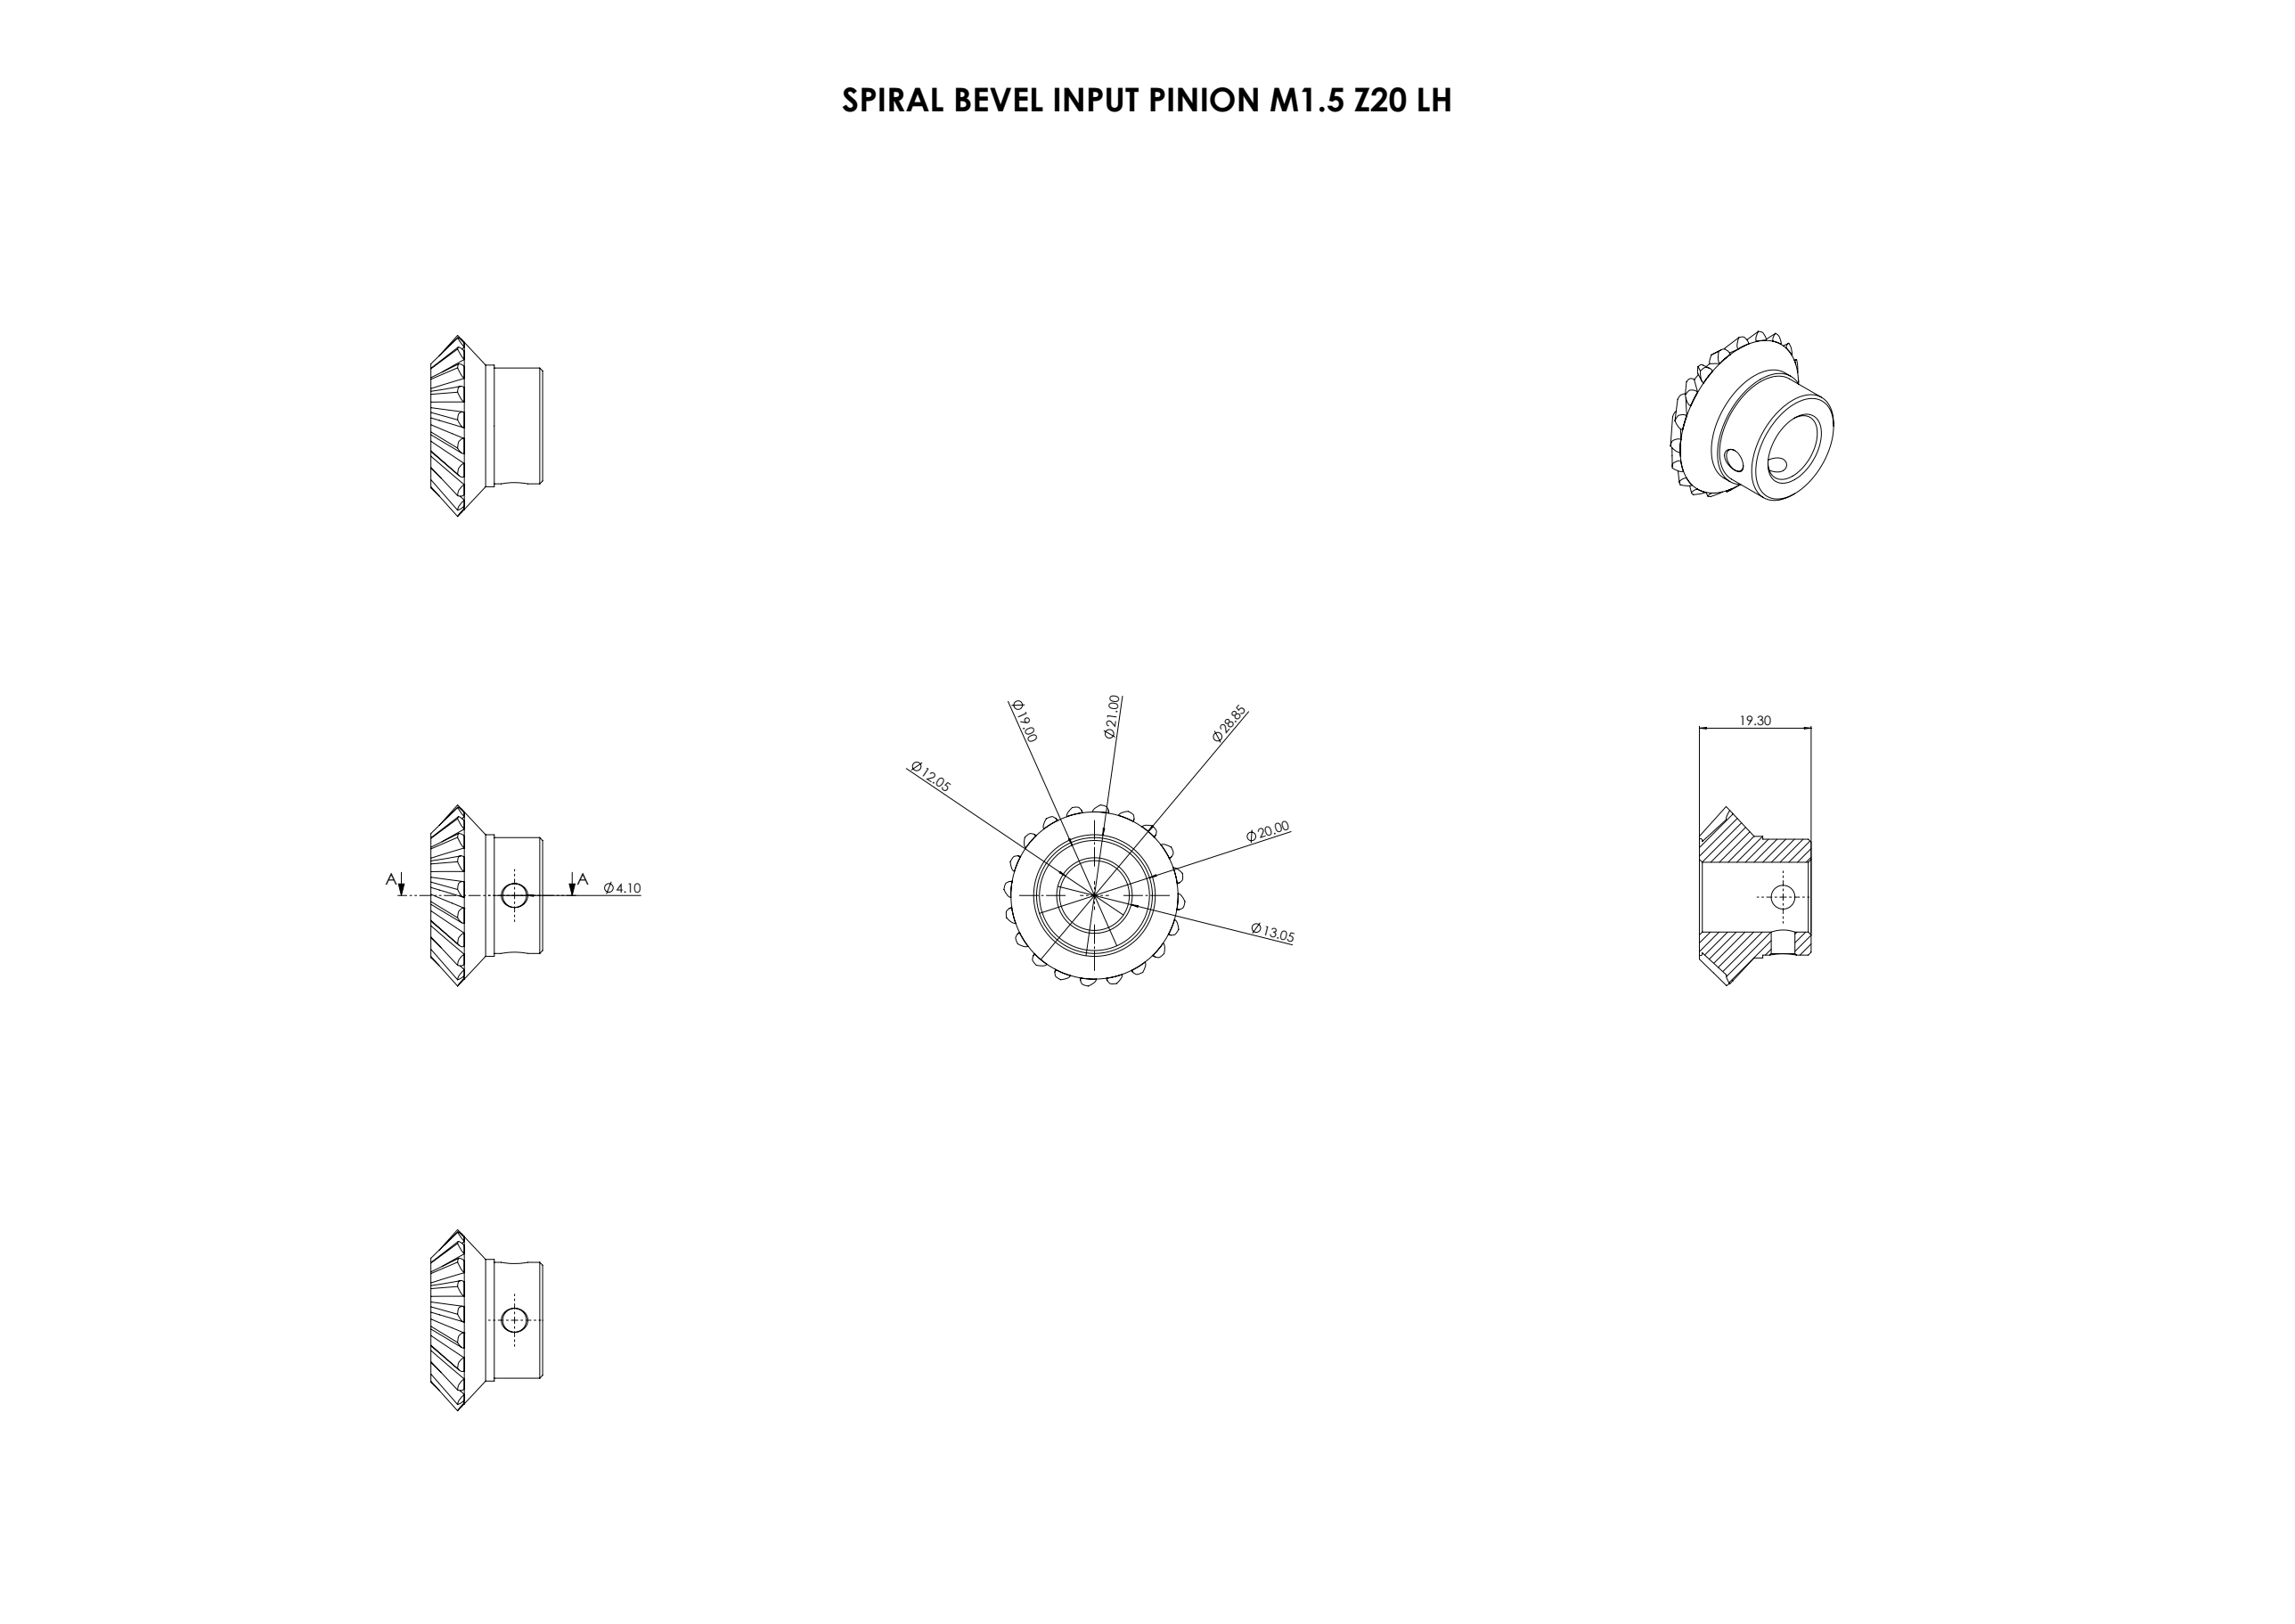
ISO-10303-21;
HEADER;
/* Generated by software containing ST-Developer
 * from STEP Tools, Inc. (www.steptools.com) 
 */

FILE_DESCRIPTION(
/* description */ (''),
/* implementation_level */ '2;1');

FILE_NAME(
/* name */ '02_Spiral_Bevel_Input_Pinion_M1.5_Z20_LH.step',
/* time_stamp */ '2026-10-11T09:12:28-07:00',
/* author */ (''),
/* organization */ (''),
/* preprocessor_version */ 'ST-DEVELOPER v20.2',
/* originating_system */ 'Autodesk Translation Framework v15.15.0.0',
/* authorisation */ '');

FILE_SCHEMA (('AUTOMOTIVE_DESIGN { 1 0 10303 214 3 1 1 }'));
ENDSEC;

DATA;
#10=MECHANICAL_DESIGN_GEOMETRIC_PRESENTATION_REPRESENTATION('',(#648),#23254);
#93=B_SPLINE_SURFACE_WITH_KNOTS('',3,3,((#12095,#12096,#12097,#12098),(#12099,
#12100,#12101,#12102),(#12103,#12104,#12105,#12106),(#12107,#12108,#12109,
#12110),(#12111,#12112,#12113,#12114),(#12115,#12116,#12117,#12118)),
 .UNSPECIFIED.,.F.,.F.,.F.,(4,1,1,4),(4,4),(0.,0.285714285714286,0.571428571428571,
1.),(0.,1.),.UNSPECIFIED.);
#94=B_SPLINE_SURFACE_WITH_KNOTS('',3,3,((#12155,#12156,#12157,#12158),(#12159,
#12160,#12161,#12162),(#12163,#12164,#12165,#12166),(#12167,#12168,#12169,
#12170),(#12171,#12172,#12173,#12174),(#12175,#12176,#12177,#12178)),
 .UNSPECIFIED.,.F.,.F.,.F.,(4,1,1,4),(4,4),(0.,0.285714285714286,0.571428571428571,
1.),(0.,1.),.UNSPECIFIED.);
#95=B_SPLINE_SURFACE_WITH_KNOTS('',3,3,((#12215,#12216,#12217,#12218),(#12219,
#12220,#12221,#12222),(#12223,#12224,#12225,#12226),(#12227,#12228,#12229,
#12230),(#12231,#12232,#12233,#12234),(#12235,#12236,#12237,#12238)),
 .UNSPECIFIED.,.F.,.F.,.F.,(4,1,1,4),(4,4),(0.,0.285714285714286,0.571428571428571,
1.),(0.,1.),.UNSPECIFIED.);
#96=B_SPLINE_SURFACE_WITH_KNOTS('',3,3,((#12275,#12276,#12277,#12278),(#12279,
#12280,#12281,#12282),(#12283,#12284,#12285,#12286),(#12287,#12288,#12289,
#12290),(#12291,#12292,#12293,#12294),(#12295,#12296,#12297,#12298)),
 .UNSPECIFIED.,.F.,.F.,.F.,(4,1,1,4),(4,4),(0.,0.285714285714286,0.571428571428571,
1.),(0.,1.),.UNSPECIFIED.);
#97=B_SPLINE_SURFACE_WITH_KNOTS('',3,3,((#12335,#12336,#12337,#12338),(#12339,
#12340,#12341,#12342),(#12343,#12344,#12345,#12346),(#12347,#12348,#12349,
#12350),(#12351,#12352,#12353,#12354),(#12355,#12356,#12357,#12358)),
 .UNSPECIFIED.,.F.,.F.,.F.,(4,1,1,4),(4,4),(0.,0.285714285714286,0.571428571428571,
1.),(0.,1.),.UNSPECIFIED.);
#98=B_SPLINE_SURFACE_WITH_KNOTS('',3,3,((#12395,#12396,#12397,#12398),(#12399,
#12400,#12401,#12402),(#12403,#12404,#12405,#12406),(#12407,#12408,#12409,
#12410),(#12411,#12412,#12413,#12414),(#12415,#12416,#12417,#12418)),
 .UNSPECIFIED.,.F.,.F.,.F.,(4,1,1,4),(4,4),(0.,0.285714285714286,0.571428571428571,
1.),(0.,1.),.UNSPECIFIED.);
#99=B_SPLINE_SURFACE_WITH_KNOTS('',3,3,((#12455,#12456,#12457,#12458),(#12459,
#12460,#12461,#12462),(#12463,#12464,#12465,#12466),(#12467,#12468,#12469,
#12470),(#12471,#12472,#12473,#12474),(#12475,#12476,#12477,#12478)),
 .UNSPECIFIED.,.F.,.F.,.F.,(4,1,1,4),(4,4),(0.,0.285714285714286,0.571428571428571,
1.),(0.,1.),.UNSPECIFIED.);
#100=B_SPLINE_SURFACE_WITH_KNOTS('',3,3,((#12515,#12516,#12517,#12518),
(#12519,#12520,#12521,#12522),(#12523,#12524,#12525,#12526),(#12527,#12528,
#12529,#12530),(#12531,#12532,#12533,#12534),(#12535,#12536,#12537,#12538)),
 .UNSPECIFIED.,.F.,.F.,.F.,(4,1,1,4),(4,4),(0.,0.285714285714286,0.571428571428571,
1.),(0.,1.),.UNSPECIFIED.);
#101=B_SPLINE_SURFACE_WITH_KNOTS('',3,3,((#12575,#12576,#12577,#12578),
(#12579,#12580,#12581,#12582),(#12583,#12584,#12585,#12586),(#12587,#12588,
#12589,#12590),(#12591,#12592,#12593,#12594),(#12595,#12596,#12597,#12598)),
 .UNSPECIFIED.,.F.,.F.,.F.,(4,1,1,4),(4,4),(0.,0.285714285714286,0.571428571428571,
1.),(0.,1.),.UNSPECIFIED.);
#102=B_SPLINE_SURFACE_WITH_KNOTS('',3,3,((#12635,#12636,#12637,#12638),
(#12639,#12640,#12641,#12642),(#12643,#12644,#12645,#12646),(#12647,#12648,
#12649,#12650),(#12651,#12652,#12653,#12654),(#12655,#12656,#12657,#12658)),
 .UNSPECIFIED.,.F.,.F.,.F.,(4,1,1,4),(4,4),(0.,0.285714285714286,0.571428571428571,
1.),(0.,1.),.UNSPECIFIED.);
#103=B_SPLINE_SURFACE_WITH_KNOTS('',3,3,((#12695,#12696,#12697,#12698),
(#12699,#12700,#12701,#12702),(#12703,#12704,#12705,#12706),(#12707,#12708,
#12709,#12710),(#12711,#12712,#12713,#12714),(#12715,#12716,#12717,#12718)),
 .UNSPECIFIED.,.F.,.F.,.F.,(4,1,1,4),(4,4),(0.,0.285714285714286,0.571428571428571,
1.),(0.,1.),.UNSPECIFIED.);
#104=B_SPLINE_SURFACE_WITH_KNOTS('',3,3,((#12731,#12732,#12733,#12734),
(#12735,#12736,#12737,#12738),(#12739,#12740,#12741,#12742),(#12743,#12744,
#12745,#12746),(#12747,#12748,#12749,#12750),(#12751,#12752,#12753,#12754)),
 .UNSPECIFIED.,.F.,.F.,.F.,(4,1,1,4),(4,4),(0.,0.285714285714286,0.571428571428571,
1.),(0.,1.),.UNSPECIFIED.);
#105=B_SPLINE_SURFACE_WITH_KNOTS('',3,3,((#12791,#12792,#12793,#12794),
(#12795,#12796,#12797,#12798),(#12799,#12800,#12801,#12802),(#12803,#12804,
#12805,#12806),(#12807,#12808,#12809,#12810),(#12811,#12812,#12813,#12814)),
 .UNSPECIFIED.,.F.,.F.,.F.,(4,1,1,4),(4,4),(0.,0.285714285714286,0.571428571428571,
1.),(0.,1.),.UNSPECIFIED.);
#106=B_SPLINE_SURFACE_WITH_KNOTS('',3,3,((#12851,#12852,#12853,#12854),
(#12855,#12856,#12857,#12858),(#12859,#12860,#12861,#12862),(#12863,#12864,
#12865,#12866),(#12867,#12868,#12869,#12870),(#12871,#12872,#12873,#12874)),
 .UNSPECIFIED.,.F.,.F.,.F.,(4,1,1,4),(4,4),(0.,0.285714285714286,0.571428571428571,
1.),(0.,1.),.UNSPECIFIED.);
#107=B_SPLINE_SURFACE_WITH_KNOTS('',3,3,((#12911,#12912,#12913,#12914),
(#12915,#12916,#12917,#12918),(#12919,#12920,#12921,#12922),(#12923,#12924,
#12925,#12926),(#12927,#12928,#12929,#12930),(#12931,#12932,#12933,#12934)),
 .UNSPECIFIED.,.F.,.F.,.F.,(4,1,1,4),(4,4),(0.,0.285714285714286,0.571428571428571,
1.),(0.,1.),.UNSPECIFIED.);
#108=B_SPLINE_SURFACE_WITH_KNOTS('',3,3,((#12971,#12972,#12973,#12974),
(#12975,#12976,#12977,#12978),(#12979,#12980,#12981,#12982),(#12983,#12984,
#12985,#12986),(#12987,#12988,#12989,#12990),(#12991,#12992,#12993,#12994)),
 .UNSPECIFIED.,.F.,.F.,.F.,(4,1,1,4),(4,4),(0.,0.285714285714286,0.571428571428571,
1.),(0.,1.),.UNSPECIFIED.);
#109=B_SPLINE_SURFACE_WITH_KNOTS('',3,3,((#13031,#13032,#13033,#13034),
(#13035,#13036,#13037,#13038),(#13039,#13040,#13041,#13042),(#13043,#13044,
#13045,#13046),(#13047,#13048,#13049,#13050),(#13051,#13052,#13053,#13054)),
 .UNSPECIFIED.,.F.,.F.,.F.,(4,1,1,4),(4,4),(0.,0.285714285714286,0.571428571428571,
1.),(0.,1.),.UNSPECIFIED.);
#110=B_SPLINE_SURFACE_WITH_KNOTS('',3,3,((#13091,#13092,#13093,#13094),
(#13095,#13096,#13097,#13098),(#13099,#13100,#13101,#13102),(#13103,#13104,
#13105,#13106),(#13107,#13108,#13109,#13110),(#13111,#13112,#13113,#13114)),
 .UNSPECIFIED.,.F.,.F.,.F.,(4,1,1,4),(4,4),(0.,0.285714285714286,0.571428571428571,
1.),(0.,1.),.UNSPECIFIED.);
#111=B_SPLINE_SURFACE_WITH_KNOTS('',3,3,((#13151,#13152,#13153,#13154),
(#13155,#13156,#13157,#13158),(#13159,#13160,#13161,#13162),(#13163,#13164,
#13165,#13166),(#13167,#13168,#13169,#13170),(#13171,#13172,#13173,#13174)),
 .UNSPECIFIED.,.F.,.F.,.F.,(4,1,1,4),(4,4),(0.,0.285714285714286,0.571428571428571,
1.),(0.,1.),.UNSPECIFIED.);
#112=B_SPLINE_SURFACE_WITH_KNOTS('',3,3,((#13211,#13212,#13213,#13214),
(#13215,#13216,#13217,#13218),(#13219,#13220,#13221,#13222),(#13223,#13224,
#13225,#13226),(#13227,#13228,#13229,#13230),(#13231,#13232,#13233,#13234)),
 .UNSPECIFIED.,.F.,.F.,.F.,(4,1,1,4),(4,4),(0.,0.285714285714286,0.571428571428571,
1.),(0.,1.),.UNSPECIFIED.);
#113=B_SPLINE_SURFACE_WITH_KNOTS('',3,3,((#13271,#13272,#13273,#13274,#13275,
#13276,#13277,#13278,#13279,#13280),(#13281,#13282,#13283,#13284,#13285,
#13286,#13287,#13288,#13289,#13290),(#13291,#13292,#13293,#13294,#13295,
#13296,#13297,#13298,#13299,#13300),(#13301,#13302,#13303,#13304,#13305,
#13306,#13307,#13308,#13309,#13310),(#13311,#13312,#13313,#13314,#13315,
#13316,#13317,#13318,#13319,#13320),(#13321,#13322,#13323,#13324,#13325,
#13326,#13327,#13328,#13329,#13330),(#13331,#13332,#13333,#13334,#13335,
#13336,#13337,#13338,#13339,#13340),(#13341,#13342,#13343,#13344,#13345,
#13346,#13347,#13348,#13349,#13350),(#13351,#13352,#13353,#13354,#13355,
#13356,#13357,#13358,#13359,#13360),(#13361,#13362,#13363,#13364,#13365,
#13366,#13367,#13368,#13369,#13370),(#13371,#13372,#13373,#13374,#13375,
#13376,#13377,#13378,#13379,#13380)),.UNSPECIFIED.,.F.,.F.,.F.,(4,1,1,1,
1,1,1,1,4),(4,1,1,1,1,1,1,4),(0.,0.142857142857143,0.285714285714286,0.357142857142857,
0.428571428571429,0.571428571428571,0.785714285714286,0.857142857142857,
1.),(0.,0.571428571428571,0.642857142857143,0.714285714285714,0.857142857142857,
0.928571428571429,0.964285714285714,1.),.UNSPECIFIED.);
#114=B_SPLINE_SURFACE_WITH_KNOTS('',3,3,((#14114,#14115,#14116,#14117,#14118,
#14119,#14120,#14121,#14122,#14123),(#14124,#14125,#14126,#14127,#14128,
#14129,#14130,#14131,#14132,#14133),(#14134,#14135,#14136,#14137,#14138,
#14139,#14140,#14141,#14142,#14143),(#14144,#14145,#14146,#14147,#14148,
#14149,#14150,#14151,#14152,#14153),(#14154,#14155,#14156,#14157,#14158,
#14159,#14160,#14161,#14162,#14163),(#14164,#14165,#14166,#14167,#14168,
#14169,#14170,#14171,#14172,#14173),(#14174,#14175,#14176,#14177,#14178,
#14179,#14180,#14181,#14182,#14183),(#14184,#14185,#14186,#14187,#14188,
#14189,#14190,#14191,#14192,#14193),(#14194,#14195,#14196,#14197,#14198,
#14199,#14200,#14201,#14202,#14203),(#14204,#14205,#14206,#14207,#14208,
#14209,#14210,#14211,#14212,#14213),(#14214,#14215,#14216,#14217,#14218,
#14219,#14220,#14221,#14222,#14223)),.UNSPECIFIED.,.F.,.F.,.F.,(4,1,1,1,
1,1,1,1,4),(4,1,1,1,1,1,1,4),(0.,0.142857142857143,0.285714285714286,0.357142857142857,
0.428571428571429,0.571428571428571,0.785714285714286,0.857142857142857,
1.),(0.,0.571428571428571,0.642857142857143,0.714285714285714,0.857142857142857,
0.928571428571429,0.964285714285714,1.),.UNSPECIFIED.);
#115=B_SPLINE_SURFACE_WITH_KNOTS('',3,3,((#14231,#14232,#14233,#14234,#14235,
#14236,#14237,#14238,#14239,#14240),(#14241,#14242,#14243,#14244,#14245,
#14246,#14247,#14248,#14249,#14250),(#14251,#14252,#14253,#14254,#14255,
#14256,#14257,#14258,#14259,#14260),(#14261,#14262,#14263,#14264,#14265,
#14266,#14267,#14268,#14269,#14270),(#14271,#14272,#14273,#14274,#14275,
#14276,#14277,#14278,#14279,#14280),(#14281,#14282,#14283,#14284,#14285,
#14286,#14287,#14288,#14289,#14290),(#14291,#14292,#14293,#14294,#14295,
#14296,#14297,#14298,#14299,#14300),(#14301,#14302,#14303,#14304,#14305,
#14306,#14307,#14308,#14309,#14310),(#14311,#14312,#14313,#14314,#14315,
#14316,#14317,#14318,#14319,#14320),(#14321,#14322,#14323,#14324,#14325,
#14326,#14327,#14328,#14329,#14330),(#14331,#14332,#14333,#14334,#14335,
#14336,#14337,#14338,#14339,#14340)),.UNSPECIFIED.,.F.,.F.,.F.,(4,1,1,1,
1,1,1,1,4),(4,1,1,1,1,1,1,4),(0.,0.142857142857143,0.285714285714286,0.357142857142857,
0.428571428571429,0.571428571428571,0.785714285714286,0.857142857142857,
1.),(0.,0.571428571428571,0.642857142857143,0.714285714285714,0.857142857142857,
0.928571428571429,0.964285714285714,1.),.UNSPECIFIED.);
#116=B_SPLINE_SURFACE_WITH_KNOTS('',3,3,((#14348,#14349,#14350,#14351),
(#14352,#14353,#14354,#14355),(#14356,#14357,#14358,#14359),(#14360,#14361,
#14362,#14363),(#14364,#14365,#14366,#14367),(#14368,#14369,#14370,#14371),
(#14372,#14373,#14374,#14375),(#14376,#14377,#14378,#14379),(#14380,#14381,
#14382,#14383),(#14384,#14385,#14386,#14387),(#14388,#14389,#14390,#14391),
(#14392,#14393,#14394,#14395)),.UNSPECIFIED.,.F.,.F.,.F.,(4,1,1,1,1,1,1,
1,1,4),(4,4),(0.,0.142857142857143,0.285714285714286,0.321428571428571,
0.357142857142857,0.428571428571429,0.571428571428571,0.785714285714286,
0.857142857142857,1.),(0.,1.),.UNSPECIFIED.);
#117=B_SPLINE_SURFACE_WITH_KNOTS('',3,3,((#14403,#14404,#14405,#14406),
(#14407,#14408,#14409,#14410),(#14411,#14412,#14413,#14414),(#14415,#14416,
#14417,#14418),(#14419,#14420,#14421,#14422),(#14423,#14424,#14425,#14426),
(#14427,#14428,#14429,#14430),(#14431,#14432,#14433,#14434),(#14435,#14436,
#14437,#14438),(#14439,#14440,#14441,#14442),(#14443,#14444,#14445,#14446),
(#14447,#14448,#14449,#14450)),.UNSPECIFIED.,.F.,.F.,.F.,(4,1,1,1,1,1,1,
1,1,4),(4,4),(0.,0.142857142857143,0.285714285714286,0.321428571428571,
0.357142857142857,0.428571428571429,0.571428571428571,0.785714285714286,
0.857142857142857,1.),(0.,1.),.UNSPECIFIED.);
#118=B_SPLINE_SURFACE_WITH_KNOTS('',3,3,((#14458,#14459,#14460,#14461,#14462,
#14463,#14464,#14465,#14466,#14467),(#14468,#14469,#14470,#14471,#14472,
#14473,#14474,#14475,#14476,#14477),(#14478,#14479,#14480,#14481,#14482,
#14483,#14484,#14485,#14486,#14487),(#14488,#14489,#14490,#14491,#14492,
#14493,#14494,#14495,#14496,#14497),(#14498,#14499,#14500,#14501,#14502,
#14503,#14504,#14505,#14506,#14507),(#14508,#14509,#14510,#14511,#14512,
#14513,#14514,#14515,#14516,#14517),(#14518,#14519,#14520,#14521,#14522,
#14523,#14524,#14525,#14526,#14527),(#14528,#14529,#14530,#14531,#14532,
#14533,#14534,#14535,#14536,#14537),(#14538,#14539,#14540,#14541,#14542,
#14543,#14544,#14545,#14546,#14547),(#14548,#14549,#14550,#14551,#14552,
#14553,#14554,#14555,#14556,#14557),(#14558,#14559,#14560,#14561,#14562,
#14563,#14564,#14565,#14566,#14567)),.UNSPECIFIED.,.F.,.F.,.F.,(4,1,1,1,
1,1,1,1,4),(4,1,1,1,1,1,1,4),(0.,0.142857142857143,0.285714285714286,0.357142857142857,
0.428571428571429,0.571428571428571,0.785714285714286,0.857142857142857,
1.),(0.,0.571428571428571,0.642857142857143,0.714285714285714,0.857142857142857,
0.928571428571429,0.964285714285714,1.),.UNSPECIFIED.);
#119=B_SPLINE_SURFACE_WITH_KNOTS('',3,3,((#14575,#14576,#14577,#14578,#14579,
#14580,#14581,#14582,#14583,#14584),(#14585,#14586,#14587,#14588,#14589,
#14590,#14591,#14592,#14593,#14594),(#14595,#14596,#14597,#14598,#14599,
#14600,#14601,#14602,#14603,#14604),(#14605,#14606,#14607,#14608,#14609,
#14610,#14611,#14612,#14613,#14614),(#14615,#14616,#14617,#14618,#14619,
#14620,#14621,#14622,#14623,#14624),(#14625,#14626,#14627,#14628,#14629,
#14630,#14631,#14632,#14633,#14634),(#14635,#14636,#14637,#14638,#14639,
#14640,#14641,#14642,#14643,#14644),(#14645,#14646,#14647,#14648,#14649,
#14650,#14651,#14652,#14653,#14654),(#14655,#14656,#14657,#14658,#14659,
#14660,#14661,#14662,#14663,#14664),(#14665,#14666,#14667,#14668,#14669,
#14670,#14671,#14672,#14673,#14674),(#14675,#14676,#14677,#14678,#14679,
#14680,#14681,#14682,#14683,#14684)),.UNSPECIFIED.,.F.,.F.,.F.,(4,1,1,1,
1,1,1,1,4),(4,1,1,1,1,1,1,4),(0.,0.142857142857143,0.285714285714286,0.357142857142857,
0.428571428571429,0.571428571428571,0.785714285714286,0.857142857142857,
1.),(0.,0.571428571428571,0.642857142857143,0.714285714285714,0.857142857142857,
0.928571428571429,0.964285714285714,1.),.UNSPECIFIED.);
#120=B_SPLINE_SURFACE_WITH_KNOTS('',3,3,((#14692,#14693,#14694,#14695,#14696,
#14697,#14698,#14699,#14700,#14701),(#14702,#14703,#14704,#14705,#14706,
#14707,#14708,#14709,#14710,#14711),(#14712,#14713,#14714,#14715,#14716,
#14717,#14718,#14719,#14720,#14721),(#14722,#14723,#14724,#14725,#14726,
#14727,#14728,#14729,#14730,#14731),(#14732,#14733,#14734,#14735,#14736,
#14737,#14738,#14739,#14740,#14741),(#14742,#14743,#14744,#14745,#14746,
#14747,#14748,#14749,#14750,#14751),(#14752,#14753,#14754,#14755,#14756,
#14757,#14758,#14759,#14760,#14761),(#14762,#14763,#14764,#14765,#14766,
#14767,#14768,#14769,#14770,#14771),(#14772,#14773,#14774,#14775,#14776,
#14777,#14778,#14779,#14780,#14781),(#14782,#14783,#14784,#14785,#14786,
#14787,#14788,#14789,#14790,#14791),(#14792,#14793,#14794,#14795,#14796,
#14797,#14798,#14799,#14800,#14801)),.UNSPECIFIED.,.F.,.F.,.F.,(4,1,1,1,
1,1,1,1,4),(4,1,1,1,1,1,1,4),(0.,0.142857142857143,0.285714285714286,0.357142857142857,
0.428571428571429,0.571428571428571,0.785714285714286,0.857142857142857,
1.),(0.,0.571428571428571,0.642857142857143,0.714285714285714,0.857142857142857,
0.928571428571429,0.964285714285714,1.),.UNSPECIFIED.);
#121=B_SPLINE_SURFACE_WITH_KNOTS('',3,3,((#14809,#14810,#14811,#14812),
(#14813,#14814,#14815,#14816),(#14817,#14818,#14819,#14820),(#14821,#14822,
#14823,#14824),(#14825,#14826,#14827,#14828),(#14829,#14830,#14831,#14832),
(#14833,#14834,#14835,#14836),(#14837,#14838,#14839,#14840),(#14841,#14842,
#14843,#14844),(#14845,#14846,#14847,#14848),(#14849,#14850,#14851,#14852),
(#14853,#14854,#14855,#14856)),.UNSPECIFIED.,.F.,.F.,.F.,(4,1,1,1,1,1,1,
1,1,4),(4,4),(0.,0.142857142857143,0.285714285714286,0.321428571428571,
0.357142857142857,0.428571428571429,0.571428571428571,0.785714285714286,
0.857142857142857,1.),(0.,1.),.UNSPECIFIED.);
#122=B_SPLINE_SURFACE_WITH_KNOTS('',3,3,((#14864,#14865,#14866,#14867),
(#14868,#14869,#14870,#14871),(#14872,#14873,#14874,#14875),(#14876,#14877,
#14878,#14879),(#14880,#14881,#14882,#14883),(#14884,#14885,#14886,#14887),
(#14888,#14889,#14890,#14891),(#14892,#14893,#14894,#14895),(#14896,#14897,
#14898,#14899),(#14900,#14901,#14902,#14903),(#14904,#14905,#14906,#14907),
(#14908,#14909,#14910,#14911)),.UNSPECIFIED.,.F.,.F.,.F.,(4,1,1,1,1,1,1,
1,1,4),(4,4),(0.,0.142857142857143,0.285714285714286,0.321428571428571,
0.357142857142857,0.428571428571429,0.571428571428571,0.785714285714286,
0.857142857142857,1.),(0.,1.),.UNSPECIFIED.);
#123=B_SPLINE_SURFACE_WITH_KNOTS('',3,3,((#14919,#14920,#14921,#14922,#14923,
#14924,#14925,#14926,#14927,#14928),(#14929,#14930,#14931,#14932,#14933,
#14934,#14935,#14936,#14937,#14938),(#14939,#14940,#14941,#14942,#14943,
#14944,#14945,#14946,#14947,#14948),(#14949,#14950,#14951,#14952,#14953,
#14954,#14955,#14956,#14957,#14958),(#14959,#14960,#14961,#14962,#14963,
#14964,#14965,#14966,#14967,#14968),(#14969,#14970,#14971,#14972,#14973,
#14974,#14975,#14976,#14977,#14978),(#14979,#14980,#14981,#14982,#14983,
#14984,#14985,#14986,#14987,#14988),(#14989,#14990,#14991,#14992,#14993,
#14994,#14995,#14996,#14997,#14998),(#14999,#15000,#15001,#15002,#15003,
#15004,#15005,#15006,#15007,#15008),(#15009,#15010,#15011,#15012,#15013,
#15014,#15015,#15016,#15017,#15018),(#15019,#15020,#15021,#15022,#15023,
#15024,#15025,#15026,#15027,#15028)),.UNSPECIFIED.,.F.,.F.,.F.,(4,1,1,1,
1,1,1,1,4),(4,1,1,1,1,1,1,4),(0.,0.142857142857143,0.285714285714286,0.357142857142857,
0.428571428571429,0.571428571428571,0.785714285714286,0.857142857142857,
1.),(0.,0.571428571428571,0.642857142857143,0.714285714285714,0.857142857142857,
0.928571428571429,0.964285714285714,1.),.UNSPECIFIED.);
#124=B_SPLINE_SURFACE_WITH_KNOTS('',3,3,((#15036,#15037,#15038,#15039,#15040,
#15041,#15042,#15043,#15044,#15045),(#15046,#15047,#15048,#15049,#15050,
#15051,#15052,#15053,#15054,#15055),(#15056,#15057,#15058,#15059,#15060,
#15061,#15062,#15063,#15064,#15065),(#15066,#15067,#15068,#15069,#15070,
#15071,#15072,#15073,#15074,#15075),(#15076,#15077,#15078,#15079,#15080,
#15081,#15082,#15083,#15084,#15085),(#15086,#15087,#15088,#15089,#15090,
#15091,#15092,#15093,#15094,#15095),(#15096,#15097,#15098,#15099,#15100,
#15101,#15102,#15103,#15104,#15105),(#15106,#15107,#15108,#15109,#15110,
#15111,#15112,#15113,#15114,#15115),(#15116,#15117,#15118,#15119,#15120,
#15121,#15122,#15123,#15124,#15125),(#15126,#15127,#15128,#15129,#15130,
#15131,#15132,#15133,#15134,#15135),(#15136,#15137,#15138,#15139,#15140,
#15141,#15142,#15143,#15144,#15145)),.UNSPECIFIED.,.F.,.F.,.F.,(4,1,1,1,
1,1,1,1,4),(4,1,1,1,1,1,1,4),(0.,0.142857142857143,0.285714285714286,0.357142857142857,
0.428571428571429,0.571428571428571,0.785714285714286,0.857142857142857,
1.),(0.,0.571428571428571,0.642857142857143,0.714285714285714,0.857142857142857,
0.928571428571429,0.964285714285714,1.),.UNSPECIFIED.);
#125=B_SPLINE_SURFACE_WITH_KNOTS('',3,3,((#15153,#15154,#15155,#15156,#15157,
#15158,#15159,#15160,#15161,#15162),(#15163,#15164,#15165,#15166,#15167,
#15168,#15169,#15170,#15171,#15172),(#15173,#15174,#15175,#15176,#15177,
#15178,#15179,#15180,#15181,#15182),(#15183,#15184,#15185,#15186,#15187,
#15188,#15189,#15190,#15191,#15192),(#15193,#15194,#15195,#15196,#15197,
#15198,#15199,#15200,#15201,#15202),(#15203,#15204,#15205,#15206,#15207,
#15208,#15209,#15210,#15211,#15212),(#15213,#15214,#15215,#15216,#15217,
#15218,#15219,#15220,#15221,#15222),(#15223,#15224,#15225,#15226,#15227,
#15228,#15229,#15230,#15231,#15232),(#15233,#15234,#15235,#15236,#15237,
#15238,#15239,#15240,#15241,#15242),(#15243,#15244,#15245,#15246,#15247,
#15248,#15249,#15250,#15251,#15252),(#15253,#15254,#15255,#15256,#15257,
#15258,#15259,#15260,#15261,#15262)),.UNSPECIFIED.,.F.,.F.,.F.,(4,1,1,1,
1,1,1,1,4),(4,1,1,1,1,1,1,4),(0.,0.142857142857143,0.285714285714286,0.357142857142857,
0.428571428571429,0.571428571428571,0.785714285714286,0.857142857142857,
1.),(0.,0.571428571428571,0.642857142857143,0.714285714285714,0.857142857142857,
0.928571428571429,0.964285714285714,1.),.UNSPECIFIED.);
#126=B_SPLINE_SURFACE_WITH_KNOTS('',3,3,((#15270,#15271,#15272,#15273),
(#15274,#15275,#15276,#15277),(#15278,#15279,#15280,#15281),(#15282,#15283,
#15284,#15285),(#15286,#15287,#15288,#15289),(#15290,#15291,#15292,#15293),
(#15294,#15295,#15296,#15297),(#15298,#15299,#15300,#15301),(#15302,#15303,
#15304,#15305),(#15306,#15307,#15308,#15309),(#15310,#15311,#15312,#15313),
(#15314,#15315,#15316,#15317)),.UNSPECIFIED.,.F.,.F.,.F.,(4,1,1,1,1,1,1,
1,1,4),(4,4),(0.,0.142857142857143,0.285714285714286,0.321428571428571,
0.357142857142857,0.428571428571429,0.571428571428571,0.785714285714286,
0.857142857142857,1.),(0.,1.),.UNSPECIFIED.);
#127=B_SPLINE_SURFACE_WITH_KNOTS('',3,3,((#15325,#15326,#15327,#15328),
(#15329,#15330,#15331,#15332),(#15333,#15334,#15335,#15336),(#15337,#15338,
#15339,#15340),(#15341,#15342,#15343,#15344),(#15345,#15346,#15347,#15348),
(#15349,#15350,#15351,#15352),(#15353,#15354,#15355,#15356),(#15357,#15358,
#15359,#15360),(#15361,#15362,#15363,#15364),(#15365,#15366,#15367,#15368),
(#15369,#15370,#15371,#15372)),.UNSPECIFIED.,.F.,.F.,.F.,(4,1,1,1,1,1,1,
1,1,4),(4,4),(0.,0.142857142857143,0.285714285714286,0.321428571428571,
0.357142857142857,0.428571428571429,0.571428571428571,0.785714285714286,
0.857142857142857,1.),(0.,1.),.UNSPECIFIED.);
#128=B_SPLINE_SURFACE_WITH_KNOTS('',3,3,((#15380,#15381,#15382,#15383,#15384,
#15385,#15386,#15387,#15388,#15389),(#15390,#15391,#15392,#15393,#15394,
#15395,#15396,#15397,#15398,#15399),(#15400,#15401,#15402,#15403,#15404,
#15405,#15406,#15407,#15408,#15409),(#15410,#15411,#15412,#15413,#15414,
#15415,#15416,#15417,#15418,#15419),(#15420,#15421,#15422,#15423,#15424,
#15425,#15426,#15427,#15428,#15429),(#15430,#15431,#15432,#15433,#15434,
#15435,#15436,#15437,#15438,#15439),(#15440,#15441,#15442,#15443,#15444,
#15445,#15446,#15447,#15448,#15449),(#15450,#15451,#15452,#15453,#15454,
#15455,#15456,#15457,#15458,#15459),(#15460,#15461,#15462,#15463,#15464,
#15465,#15466,#15467,#15468,#15469),(#15470,#15471,#15472,#15473,#15474,
#15475,#15476,#15477,#15478,#15479),(#15480,#15481,#15482,#15483,#15484,
#15485,#15486,#15487,#15488,#15489)),.UNSPECIFIED.,.F.,.F.,.F.,(4,1,1,1,
1,1,1,1,4),(4,1,1,1,1,1,1,4),(0.,0.142857142857143,0.285714285714286,0.357142857142857,
0.428571428571429,0.571428571428571,0.785714285714286,0.857142857142857,
1.),(0.,0.571428571428571,0.642857142857143,0.714285714285714,0.857142857142857,
0.928571428571429,0.964285714285714,1.),.UNSPECIFIED.);
#129=B_SPLINE_SURFACE_WITH_KNOTS('',3,3,((#15497,#15498,#15499,#15500,#15501,
#15502,#15503,#15504,#15505,#15506),(#15507,#15508,#15509,#15510,#15511,
#15512,#15513,#15514,#15515,#15516),(#15517,#15518,#15519,#15520,#15521,
#15522,#15523,#15524,#15525,#15526),(#15527,#15528,#15529,#15530,#15531,
#15532,#15533,#15534,#15535,#15536),(#15537,#15538,#15539,#15540,#15541,
#15542,#15543,#15544,#15545,#15546),(#15547,#15548,#15549,#15550,#15551,
#15552,#15553,#15554,#15555,#15556),(#15557,#15558,#15559,#15560,#15561,
#15562,#15563,#15564,#15565,#15566),(#15567,#15568,#15569,#15570,#15571,
#15572,#15573,#15574,#15575,#15576),(#15577,#15578,#15579,#15580,#15581,
#15582,#15583,#15584,#15585,#15586),(#15587,#15588,#15589,#15590,#15591,
#15592,#15593,#15594,#15595,#15596),(#15597,#15598,#15599,#15600,#15601,
#15602,#15603,#15604,#15605,#15606)),.UNSPECIFIED.,.F.,.F.,.F.,(4,1,1,1,
1,1,1,1,4),(4,1,1,1,1,1,1,4),(0.,0.142857142857143,0.285714285714286,0.357142857142857,
0.428571428571429,0.571428571428571,0.785714285714286,0.857142857142857,
1.),(0.,0.571428571428571,0.642857142857143,0.714285714285714,0.857142857142857,
0.928571428571429,0.964285714285714,1.),.UNSPECIFIED.);
#130=B_SPLINE_SURFACE_WITH_KNOTS('',3,3,((#15614,#15615,#15616,#15617,#15618,
#15619,#15620,#15621,#15622,#15623),(#15624,#15625,#15626,#15627,#15628,
#15629,#15630,#15631,#15632,#15633),(#15634,#15635,#15636,#15637,#15638,
#15639,#15640,#15641,#15642,#15643),(#15644,#15645,#15646,#15647,#15648,
#15649,#15650,#15651,#15652,#15653),(#15654,#15655,#15656,#15657,#15658,
#15659,#15660,#15661,#15662,#15663),(#15664,#15665,#15666,#15667,#15668,
#15669,#15670,#15671,#15672,#15673),(#15674,#15675,#15676,#15677,#15678,
#15679,#15680,#15681,#15682,#15683),(#15684,#15685,#15686,#15687,#15688,
#15689,#15690,#15691,#15692,#15693),(#15694,#15695,#15696,#15697,#15698,
#15699,#15700,#15701,#15702,#15703),(#15704,#15705,#15706,#15707,#15708,
#15709,#15710,#15711,#15712,#15713),(#15714,#15715,#15716,#15717,#15718,
#15719,#15720,#15721,#15722,#15723)),.UNSPECIFIED.,.F.,.F.,.F.,(4,1,1,1,
1,1,1,1,4),(4,1,1,1,1,1,1,4),(0.,0.142857142857143,0.285714285714286,0.357142857142857,
0.428571428571429,0.571428571428571,0.785714285714286,0.857142857142857,
1.),(0.,0.571428571428571,0.642857142857143,0.714285714285714,0.857142857142857,
0.928571428571429,0.964285714285714,1.),.UNSPECIFIED.);
#131=B_SPLINE_SURFACE_WITH_KNOTS('',3,3,((#15731,#15732,#15733,#15734),
(#15735,#15736,#15737,#15738),(#15739,#15740,#15741,#15742),(#15743,#15744,
#15745,#15746),(#15747,#15748,#15749,#15750),(#15751,#15752,#15753,#15754),
(#15755,#15756,#15757,#15758),(#15759,#15760,#15761,#15762),(#15763,#15764,
#15765,#15766),(#15767,#15768,#15769,#15770),(#15771,#15772,#15773,#15774),
(#15775,#15776,#15777,#15778)),.UNSPECIFIED.,.F.,.F.,.F.,(4,1,1,1,1,1,1,
1,1,4),(4,4),(0.,0.142857142857143,0.285714285714286,0.321428571428571,
0.357142857142857,0.428571428571429,0.571428571428571,0.785714285714286,
0.857142857142857,1.),(0.,1.),.UNSPECIFIED.);
#132=B_SPLINE_SURFACE_WITH_KNOTS('',3,3,((#15786,#15787,#15788,#15789),
(#15790,#15791,#15792,#15793),(#15794,#15795,#15796,#15797),(#15798,#15799,
#15800,#15801),(#15802,#15803,#15804,#15805),(#15806,#15807,#15808,#15809),
(#15810,#15811,#15812,#15813),(#15814,#15815,#15816,#15817),(#15818,#15819,
#15820,#15821),(#15822,#15823,#15824,#15825),(#15826,#15827,#15828,#15829),
(#15830,#15831,#15832,#15833)),.UNSPECIFIED.,.F.,.F.,.F.,(4,1,1,1,1,1,1,
1,1,4),(4,4),(0.,0.142857142857143,0.285714285714286,0.321428571428571,
0.357142857142857,0.428571428571429,0.571428571428571,0.785714285714286,
0.857142857142857,1.),(0.,1.),.UNSPECIFIED.);
#175=(
BOUNDED_CURVE()
B_SPLINE_CURVE(5,(#9974,#9975,#9976,#9977,#9978,#9979,#9980,#9981,#9982,
#9983,#9984,#9985,#9986,#9987,#9988,#9989,#9990,#9991,#9992,#9993,#9994,
#9995,#9996,#9997,#9998,#9999,#10000,#10001,#10002,#10003,#10004,#10005,
#10006,#10007,#10008),.UNSPECIFIED.,.F.,.F.)
B_SPLINE_CURVE_WITH_KNOTS((6,1,1,1,1,1,1,1,1,1,1,1,1,1,1,1,1,1,1,1,1,1,
1,1,1,1,1,1,1,1,6),(0.,0.0333333333333333,0.0666666666666667,0.1,0.133333333333333,
0.166666666666667,0.2,0.233333333333333,0.266666666666667,0.3,0.333333333333333,
0.366666666666667,0.4,0.433333333333333,0.466666666666667,0.5,0.533333333333333,
0.566666666666667,0.6,0.633333333333333,0.666666666666667,0.7,0.733333333333333,
0.766666666666667,0.8,0.833333333333333,0.866666666666667,0.9,0.933333333333333,
0.966666666666667,1.),.UNSPECIFIED.)
CURVE()
GEOMETRIC_REPRESENTATION_ITEM()
RATIONAL_B_SPLINE_CURVE((1.,1.,1.,1.,1.,1.,1.,1.,1.,1.,1.,1.,1.,1.,1.,1.,
1.,1.,1.,1.,1.,1.,1.,1.,1.,1.,1.,1.,1.,1.,1.,1.,1.,1.,1.))
REPRESENTATION_ITEM('')
);
#176=(
BOUNDED_CURVE()
B_SPLINE_CURVE(5,(#10010,#10011,#10012,#10013,#10014,#10015,#10016,#10017,
#10018,#10019,#10020,#10021,#10022,#10023,#10024,#10025,#10026,#10027,#10028,
#10029,#10030,#10031,#10032,#10033,#10034,#10035,#10036,#10037,#10038,#10039,
#10040,#10041,#10042,#10043,#10044),.UNSPECIFIED.,.F.,.F.)
B_SPLINE_CURVE_WITH_KNOTS((6,1,1,1,1,1,1,1,1,1,1,1,1,1,1,1,1,1,1,1,1,1,
1,1,1,1,1,1,1,1,6),(0.,0.0333333333333333,0.0666666666666667,0.1,0.133333333333333,
0.166666666666667,0.2,0.233333333333333,0.266666666666667,0.3,0.333333333333333,
0.366666666666667,0.4,0.433333333333333,0.466666666666667,0.5,0.533333333333333,
0.566666666666667,0.6,0.633333333333333,0.666666666666667,0.7,0.733333333333333,
0.766666666666667,0.8,0.833333333333333,0.866666666666667,0.9,0.933333333333333,
0.966666666666667,1.),.UNSPECIFIED.)
CURVE()
GEOMETRIC_REPRESENTATION_ITEM()
RATIONAL_B_SPLINE_CURVE((1.,1.,1.,1.,1.,1.,1.,1.,1.,1.,1.,1.,1.,1.,1.,1.,
1.,1.,1.,1.,1.,1.,1.,1.,1.,1.,1.,1.,1.,1.,1.,1.,1.,1.,1.))
REPRESENTATION_ITEM('')
);
#177=(
BOUNDED_CURVE()
B_SPLINE_CURVE(5,(#10048,#10049,#10050,#10051,#10052,#10053,#10054,#10055,
#10056,#10057,#10058,#10059,#10060,#10061,#10062,#10063,#10064,#10065,#10066,
#10067,#10068,#10069,#10070,#10071,#10072,#10073,#10074,#10075,#10076,#10077,
#10078,#10079,#10080,#10081,#10082),.UNSPECIFIED.,.F.,.F.)
B_SPLINE_CURVE_WITH_KNOTS((6,1,1,1,1,1,1,1,1,1,1,1,1,1,1,1,1,1,1,1,1,1,
1,1,1,1,1,1,1,1,6),(0.,0.0333333333333333,0.0666666666666667,0.1,0.133333333333333,
0.166666666666667,0.2,0.233333333333333,0.266666666666667,0.3,0.333333333333333,
0.366666666666667,0.4,0.433333333333333,0.466666666666667,0.5,0.533333333333333,
0.566666666666667,0.6,0.633333333333333,0.666666666666667,0.7,0.733333333333333,
0.766666666666667,0.8,0.833333333333333,0.866666666666667,0.9,0.933333333333333,
0.966666666666667,1.),.UNSPECIFIED.)
CURVE()
GEOMETRIC_REPRESENTATION_ITEM()
RATIONAL_B_SPLINE_CURVE((1.,1.,1.,1.,1.,1.,1.,1.,1.,1.,1.,1.,1.,1.,1.,1.,
1.,1.,1.,1.,1.,1.,1.,1.,1.,1.,1.,1.,1.,1.,1.,1.,1.,1.,1.))
REPRESENTATION_ITEM('')
);
#178=(
BOUNDED_CURVE()
B_SPLINE_CURVE(5,(#10084,#10085,#10086,#10087,#10088,#10089,#10090,#10091,
#10092,#10093,#10094,#10095,#10096,#10097,#10098,#10099,#10100,#10101,#10102,
#10103,#10104,#10105,#10106,#10107,#10108,#10109,#10110,#10111,#10112,#10113,
#10114,#10115,#10116,#10117,#10118),.UNSPECIFIED.,.F.,.F.)
B_SPLINE_CURVE_WITH_KNOTS((6,1,1,1,1,1,1,1,1,1,1,1,1,1,1,1,1,1,1,1,1,1,
1,1,1,1,1,1,1,1,6),(0.,0.0333333333333333,0.0666666666666667,0.1,0.133333333333333,
0.166666666666667,0.2,0.233333333333333,0.266666666666667,0.3,0.333333333333333,
0.366666666666667,0.4,0.433333333333333,0.466666666666667,0.5,0.533333333333333,
0.566666666666667,0.6,0.633333333333333,0.666666666666667,0.7,0.733333333333333,
0.766666666666667,0.8,0.833333333333333,0.866666666666667,0.9,0.933333333333333,
0.966666666666667,1.),.UNSPECIFIED.)
CURVE()
GEOMETRIC_REPRESENTATION_ITEM()
RATIONAL_B_SPLINE_CURVE((1.,1.,1.,1.,1.,1.,1.,1.,1.,1.,1.,1.,1.,1.,1.,1.,
1.,1.,1.,1.,1.,1.,1.,1.,1.,1.,1.,1.,1.,1.,1.,1.,1.,1.,1.))
REPRESENTATION_ITEM('')
);
#179=(
BOUNDED_CURVE()
B_SPLINE_CURVE(5,(#10122,#10123,#10124,#10125,#10126,#10127,#10128,#10129,
#10130,#10131,#10132,#10133,#10134,#10135,#10136,#10137,#10138,#10139,#10140,
#10141,#10142,#10143,#10144,#10145,#10146,#10147,#10148,#10149,#10150,#10151,
#10152,#10153,#10154,#10155,#10156),.UNSPECIFIED.,.F.,.F.)
B_SPLINE_CURVE_WITH_KNOTS((6,1,1,1,1,1,1,1,1,1,1,1,1,1,1,1,1,1,1,1,1,1,
1,1,1,1,1,1,1,1,6),(0.,0.0333333333333333,0.0666666666666667,0.1,0.133333333333333,
0.166666666666667,0.2,0.233333333333333,0.266666666666667,0.3,0.333333333333333,
0.366666666666667,0.4,0.433333333333333,0.466666666666667,0.5,0.533333333333333,
0.566666666666667,0.6,0.633333333333333,0.666666666666667,0.7,0.733333333333333,
0.766666666666667,0.8,0.833333333333333,0.866666666666667,0.9,0.933333333333333,
0.966666666666667,1.),.UNSPECIFIED.)
CURVE()
GEOMETRIC_REPRESENTATION_ITEM()
RATIONAL_B_SPLINE_CURVE((1.,1.,1.,1.,1.,1.,1.,1.,1.,1.,1.,1.,1.,1.,1.,1.,
1.,1.,1.,1.,1.,1.,1.,1.,1.,1.,1.,1.,1.,1.,1.,1.,1.,1.,1.))
REPRESENTATION_ITEM('')
);
#180=(
BOUNDED_CURVE()
B_SPLINE_CURVE(5,(#10158,#10159,#10160,#10161,#10162,#10163,#10164,#10165,
#10166,#10167,#10168,#10169,#10170,#10171,#10172,#10173,#10174,#10175,#10176,
#10177,#10178,#10179,#10180,#10181,#10182,#10183,#10184,#10185,#10186,#10187,
#10188,#10189,#10190,#10191,#10192),.UNSPECIFIED.,.F.,.F.)
B_SPLINE_CURVE_WITH_KNOTS((6,1,1,1,1,1,1,1,1,1,1,1,1,1,1,1,1,1,1,1,1,1,
1,1,1,1,1,1,1,1,6),(0.,0.0333333333333333,0.0666666666666667,0.1,0.133333333333333,
0.166666666666667,0.2,0.233333333333333,0.266666666666667,0.3,0.333333333333333,
0.366666666666667,0.4,0.433333333333333,0.466666666666667,0.5,0.533333333333333,
0.566666666666667,0.6,0.633333333333333,0.666666666666667,0.7,0.733333333333333,
0.766666666666667,0.8,0.833333333333333,0.866666666666667,0.9,0.933333333333333,
0.966666666666667,1.),.UNSPECIFIED.)
CURVE()
GEOMETRIC_REPRESENTATION_ITEM()
RATIONAL_B_SPLINE_CURVE((1.,1.,1.,1.,1.,1.,1.,1.,1.,1.,1.,1.,1.,1.,1.,1.,
1.,1.,1.,1.,1.,1.,1.,1.,1.,1.,1.,1.,1.,1.,1.,1.,1.,1.,1.))
REPRESENTATION_ITEM('')
);
#181=(
BOUNDED_CURVE()
B_SPLINE_CURVE(5,(#10196,#10197,#10198,#10199,#10200,#10201,#10202,#10203,
#10204,#10205,#10206,#10207,#10208,#10209,#10210,#10211,#10212,#10213,#10214,
#10215,#10216,#10217,#10218,#10219,#10220,#10221,#10222,#10223,#10224,#10225,
#10226,#10227,#10228,#10229,#10230),.UNSPECIFIED.,.F.,.F.)
B_SPLINE_CURVE_WITH_KNOTS((6,1,1,1,1,1,1,1,1,1,1,1,1,1,1,1,1,1,1,1,1,1,
1,1,1,1,1,1,1,1,6),(0.,0.0333333333333333,0.0666666666666667,0.1,0.133333333333333,
0.166666666666667,0.2,0.233333333333333,0.266666666666667,0.3,0.333333333333333,
0.366666666666667,0.4,0.433333333333333,0.466666666666667,0.5,0.533333333333333,
0.566666666666667,0.6,0.633333333333333,0.666666666666667,0.7,0.733333333333333,
0.766666666666667,0.8,0.833333333333333,0.866666666666667,0.9,0.933333333333333,
0.966666666666667,1.),.UNSPECIFIED.)
CURVE()
GEOMETRIC_REPRESENTATION_ITEM()
RATIONAL_B_SPLINE_CURVE((1.,1.,1.,1.,1.,1.,1.,1.,1.,1.,1.,1.,1.,1.,1.,1.,
1.,1.,1.,1.,1.,1.,1.,1.,1.,1.,1.,1.,1.,1.,1.,1.,1.,1.,1.))
REPRESENTATION_ITEM('')
);
#182=(
BOUNDED_CURVE()
B_SPLINE_CURVE(5,(#10232,#10233,#10234,#10235,#10236,#10237,#10238,#10239,
#10240,#10241,#10242,#10243,#10244,#10245,#10246,#10247,#10248,#10249,#10250,
#10251,#10252,#10253,#10254,#10255,#10256,#10257,#10258,#10259,#10260,#10261,
#10262,#10263,#10264,#10265,#10266),.UNSPECIFIED.,.F.,.F.)
B_SPLINE_CURVE_WITH_KNOTS((6,1,1,1,1,1,1,1,1,1,1,1,1,1,1,1,1,1,1,1,1,1,
1,1,1,1,1,1,1,1,6),(0.,0.0333333333333333,0.0666666666666667,0.1,0.133333333333333,
0.166666666666667,0.2,0.233333333333333,0.266666666666667,0.3,0.333333333333333,
0.366666666666667,0.4,0.433333333333333,0.466666666666667,0.5,0.533333333333333,
0.566666666666667,0.6,0.633333333333333,0.666666666666667,0.7,0.733333333333333,
0.766666666666667,0.8,0.833333333333333,0.866666666666667,0.9,0.933333333333333,
0.966666666666667,1.),.UNSPECIFIED.)
CURVE()
GEOMETRIC_REPRESENTATION_ITEM()
RATIONAL_B_SPLINE_CURVE((1.,1.,1.,1.,1.,1.,1.,1.,1.,1.,1.,1.,1.,1.,1.,1.,
1.,1.,1.,1.,1.,1.,1.,1.,1.,1.,1.,1.,1.,1.,1.,1.,1.,1.,1.))
REPRESENTATION_ITEM('')
);
#183=(
BOUNDED_CURVE()
B_SPLINE_CURVE(5,(#10270,#10271,#10272,#10273,#10274,#10275,#10276,#10277,
#10278,#10279,#10280,#10281,#10282,#10283,#10284,#10285,#10286,#10287,#10288,
#10289,#10290,#10291,#10292,#10293,#10294,#10295,#10296,#10297,#10298,#10299,
#10300,#10301,#10302,#10303,#10304),.UNSPECIFIED.,.F.,.F.)
B_SPLINE_CURVE_WITH_KNOTS((6,1,1,1,1,1,1,1,1,1,1,1,1,1,1,1,1,1,1,1,1,1,
1,1,1,1,1,1,1,1,6),(0.,0.0333333333333333,0.0666666666666667,0.1,0.133333333333333,
0.166666666666667,0.2,0.233333333333333,0.266666666666667,0.3,0.333333333333333,
0.366666666666667,0.4,0.433333333333333,0.466666666666667,0.5,0.533333333333333,
0.566666666666667,0.6,0.633333333333333,0.666666666666667,0.7,0.733333333333333,
0.766666666666667,0.8,0.833333333333333,0.866666666666667,0.9,0.933333333333333,
0.966666666666667,1.),.UNSPECIFIED.)
CURVE()
GEOMETRIC_REPRESENTATION_ITEM()
RATIONAL_B_SPLINE_CURVE((1.,1.,1.,1.,1.,1.,1.,1.,1.,1.,1.,1.,1.,1.,1.,1.,
1.,1.,1.,1.,1.,1.,1.,1.,1.,1.,1.,1.,1.,1.,1.,1.,1.,1.,1.))
REPRESENTATION_ITEM('')
);
#184=(
BOUNDED_CURVE()
B_SPLINE_CURVE(5,(#10306,#10307,#10308,#10309,#10310,#10311,#10312,#10313,
#10314,#10315,#10316,#10317,#10318,#10319,#10320,#10321,#10322,#10323,#10324,
#10325,#10326,#10327,#10328,#10329,#10330,#10331,#10332,#10333,#10334,#10335,
#10336,#10337,#10338,#10339,#10340),.UNSPECIFIED.,.F.,.F.)
B_SPLINE_CURVE_WITH_KNOTS((6,1,1,1,1,1,1,1,1,1,1,1,1,1,1,1,1,1,1,1,1,1,
1,1,1,1,1,1,1,1,6),(0.,0.0333333333333333,0.0666666666666667,0.1,0.133333333333333,
0.166666666666667,0.2,0.233333333333333,0.266666666666667,0.3,0.333333333333333,
0.366666666666667,0.4,0.433333333333333,0.466666666666667,0.5,0.533333333333333,
0.566666666666667,0.6,0.633333333333333,0.666666666666667,0.7,0.733333333333333,
0.766666666666667,0.8,0.833333333333333,0.866666666666667,0.9,0.933333333333333,
0.966666666666667,1.),.UNSPECIFIED.)
CURVE()
GEOMETRIC_REPRESENTATION_ITEM()
RATIONAL_B_SPLINE_CURVE((1.,1.,1.,1.,1.,1.,1.,1.,1.,1.,1.,1.,1.,1.,1.,1.,
1.,1.,1.,1.,1.,1.,1.,1.,1.,1.,1.,1.,1.,1.,1.,1.,1.,1.,1.))
REPRESENTATION_ITEM('')
);
#185=(
BOUNDED_CURVE()
B_SPLINE_CURVE(5,(#10344,#10345,#10346,#10347,#10348,#10349,#10350,#10351,
#10352,#10353,#10354,#10355,#10356,#10357,#10358,#10359,#10360,#10361,#10362,
#10363,#10364,#10365,#10366,#10367,#10368,#10369,#10370,#10371,#10372,#10373,
#10374,#10375,#10376,#10377,#10378),.UNSPECIFIED.,.F.,.F.)
B_SPLINE_CURVE_WITH_KNOTS((6,1,1,1,1,1,1,1,1,1,1,1,1,1,1,1,1,1,1,1,1,1,
1,1,1,1,1,1,1,1,6),(0.,0.0333333333333333,0.0666666666666667,0.1,0.133333333333333,
0.166666666666667,0.2,0.233333333333333,0.266666666666667,0.3,0.333333333333333,
0.366666666666667,0.4,0.433333333333333,0.466666666666667,0.5,0.533333333333333,
0.566666666666667,0.6,0.633333333333333,0.666666666666667,0.7,0.733333333333333,
0.766666666666667,0.8,0.833333333333333,0.866666666666667,0.9,0.933333333333333,
0.966666666666667,1.),.UNSPECIFIED.)
CURVE()
GEOMETRIC_REPRESENTATION_ITEM()
RATIONAL_B_SPLINE_CURVE((1.,1.,1.,1.,1.,1.,1.,1.,1.,1.,1.,1.,1.,1.,1.,1.,
1.,1.,1.,1.,1.,1.,1.,1.,1.,1.,1.,1.,1.,1.,1.,1.,1.,1.,1.))
REPRESENTATION_ITEM('')
);
#186=(
BOUNDED_CURVE()
B_SPLINE_CURVE(5,(#10380,#10381,#10382,#10383,#10384,#10385,#10386,#10387,
#10388,#10389,#10390,#10391,#10392,#10393,#10394,#10395,#10396,#10397,#10398,
#10399,#10400,#10401,#10402,#10403,#10404,#10405,#10406,#10407,#10408,#10409,
#10410,#10411,#10412,#10413,#10414),.UNSPECIFIED.,.F.,.F.)
B_SPLINE_CURVE_WITH_KNOTS((6,1,1,1,1,1,1,1,1,1,1,1,1,1,1,1,1,1,1,1,1,1,
1,1,1,1,1,1,1,1,6),(0.,0.0333333333333333,0.0666666666666667,0.1,0.133333333333333,
0.166666666666667,0.2,0.233333333333333,0.266666666666667,0.3,0.333333333333333,
0.366666666666667,0.4,0.433333333333333,0.466666666666667,0.5,0.533333333333333,
0.566666666666667,0.6,0.633333333333333,0.666666666666667,0.7,0.733333333333333,
0.766666666666667,0.8,0.833333333333333,0.866666666666667,0.9,0.933333333333333,
0.966666666666667,1.),.UNSPECIFIED.)
CURVE()
GEOMETRIC_REPRESENTATION_ITEM()
RATIONAL_B_SPLINE_CURVE((1.,1.,1.,1.,1.,1.,1.,1.,1.,1.,1.,1.,1.,1.,1.,1.,
1.,1.,1.,1.,1.,1.,1.,1.,1.,1.,1.,1.,1.,1.,1.,1.,1.,1.,1.))
REPRESENTATION_ITEM('')
);
#187=(
BOUNDED_CURVE()
B_SPLINE_CURVE(5,(#10418,#10419,#10420,#10421,#10422,#10423,#10424,#10425,
#10426,#10427,#10428,#10429,#10430,#10431,#10432,#10433,#10434,#10435,#10436,
#10437,#10438,#10439,#10440,#10441,#10442,#10443,#10444,#10445,#10446,#10447,
#10448,#10449,#10450,#10451,#10452),.UNSPECIFIED.,.F.,.F.)
B_SPLINE_CURVE_WITH_KNOTS((6,1,1,1,1,1,1,1,1,1,1,1,1,1,1,1,1,1,1,1,1,1,
1,1,1,1,1,1,1,1,6),(0.,0.0333333333333333,0.0666666666666667,0.1,0.133333333333333,
0.166666666666667,0.2,0.233333333333333,0.266666666666667,0.3,0.333333333333333,
0.366666666666667,0.4,0.433333333333333,0.466666666666667,0.5,0.533333333333333,
0.566666666666667,0.6,0.633333333333333,0.666666666666667,0.7,0.733333333333333,
0.766666666666667,0.8,0.833333333333333,0.866666666666667,0.9,0.933333333333333,
0.966666666666667,1.),.UNSPECIFIED.)
CURVE()
GEOMETRIC_REPRESENTATION_ITEM()
RATIONAL_B_SPLINE_CURVE((1.,1.,1.,1.,1.,1.,1.,1.,1.,1.,1.,1.,1.,1.,1.,1.,
1.,1.,1.,1.,1.,1.,1.,1.,1.,1.,1.,1.,1.,1.,1.,1.,1.,1.,1.))
REPRESENTATION_ITEM('')
);
#188=(
BOUNDED_CURVE()
B_SPLINE_CURVE(5,(#10454,#10455,#10456,#10457,#10458,#10459,#10460,#10461,
#10462,#10463,#10464,#10465,#10466,#10467,#10468,#10469,#10470,#10471,#10472,
#10473,#10474,#10475,#10476,#10477,#10478,#10479,#10480,#10481,#10482,#10483,
#10484,#10485,#10486,#10487,#10488),.UNSPECIFIED.,.F.,.F.)
B_SPLINE_CURVE_WITH_KNOTS((6,1,1,1,1,1,1,1,1,1,1,1,1,1,1,1,1,1,1,1,1,1,
1,1,1,1,1,1,1,1,6),(0.,0.0333333333333333,0.0666666666666667,0.1,0.133333333333333,
0.166666666666667,0.2,0.233333333333333,0.266666666666667,0.3,0.333333333333333,
0.366666666666667,0.4,0.433333333333333,0.466666666666667,0.5,0.533333333333333,
0.566666666666667,0.6,0.633333333333333,0.666666666666667,0.7,0.733333333333333,
0.766666666666667,0.8,0.833333333333333,0.866666666666667,0.9,0.933333333333333,
0.966666666666667,1.),.UNSPECIFIED.)
CURVE()
GEOMETRIC_REPRESENTATION_ITEM()
RATIONAL_B_SPLINE_CURVE((1.,1.,1.,1.,1.,1.,1.,1.,1.,1.,1.,1.,1.,1.,1.,1.,
1.,1.,1.,1.,1.,1.,1.,1.,1.,1.,1.,1.,1.,1.,1.,1.,1.,1.,1.))
REPRESENTATION_ITEM('')
);
#189=(
BOUNDED_CURVE()
B_SPLINE_CURVE(5,(#10492,#10493,#10494,#10495,#10496,#10497,#10498,#10499,
#10500,#10501,#10502,#10503,#10504,#10505,#10506,#10507,#10508,#10509,#10510,
#10511,#10512,#10513,#10514,#10515,#10516,#10517,#10518,#10519,#10520,#10521,
#10522,#10523,#10524,#10525,#10526),.UNSPECIFIED.,.F.,.F.)
B_SPLINE_CURVE_WITH_KNOTS((6,1,1,1,1,1,1,1,1,1,1,1,1,1,1,1,1,1,1,1,1,1,
1,1,1,1,1,1,1,1,6),(0.,0.0333333333333333,0.0666666666666667,0.1,0.133333333333333,
0.166666666666667,0.2,0.233333333333333,0.266666666666667,0.3,0.333333333333333,
0.366666666666667,0.4,0.433333333333333,0.466666666666667,0.5,0.533333333333333,
0.566666666666667,0.6,0.633333333333333,0.666666666666667,0.7,0.733333333333333,
0.766666666666667,0.8,0.833333333333333,0.866666666666667,0.9,0.933333333333333,
0.966666666666667,1.),.UNSPECIFIED.)
CURVE()
GEOMETRIC_REPRESENTATION_ITEM()
RATIONAL_B_SPLINE_CURVE((1.,1.,1.,1.,1.,1.,1.,1.,1.,1.,1.,1.,1.,1.,1.,1.,
1.,1.,1.,1.,1.,1.,1.,1.,1.,1.,1.,1.,1.,1.,1.,1.,1.,1.,1.))
REPRESENTATION_ITEM('')
);
#190=(
BOUNDED_CURVE()
B_SPLINE_CURVE(5,(#10528,#10529,#10530,#10531,#10532,#10533,#10534,#10535,
#10536,#10537,#10538,#10539,#10540,#10541,#10542,#10543,#10544,#10545,#10546,
#10547,#10548,#10549,#10550,#10551,#10552,#10553,#10554,#10555,#10556,#10557,
#10558,#10559,#10560,#10561,#10562),.UNSPECIFIED.,.F.,.F.)
B_SPLINE_CURVE_WITH_KNOTS((6,1,1,1,1,1,1,1,1,1,1,1,1,1,1,1,1,1,1,1,1,1,
1,1,1,1,1,1,1,1,6),(0.,0.0333333333333333,0.0666666666666667,0.1,0.133333333333333,
0.166666666666667,0.2,0.233333333333333,0.266666666666667,0.3,0.333333333333333,
0.366666666666667,0.4,0.433333333333333,0.466666666666667,0.5,0.533333333333333,
0.566666666666667,0.6,0.633333333333333,0.666666666666667,0.7,0.733333333333333,
0.766666666666667,0.8,0.833333333333333,0.866666666666667,0.9,0.933333333333333,
0.966666666666667,1.),.UNSPECIFIED.)
CURVE()
GEOMETRIC_REPRESENTATION_ITEM()
RATIONAL_B_SPLINE_CURVE((1.,1.,1.,1.,1.,1.,1.,1.,1.,1.,1.,1.,1.,1.,1.,1.,
1.,1.,1.,1.,1.,1.,1.,1.,1.,1.,1.,1.,1.,1.,1.,1.,1.,1.,1.))
REPRESENTATION_ITEM('')
);
#191=(
BOUNDED_CURVE()
B_SPLINE_CURVE(5,(#10566,#10567,#10568,#10569,#10570,#10571,#10572,#10573,
#10574,#10575,#10576,#10577,#10578,#10579,#10580,#10581,#10582,#10583,#10584,
#10585,#10586,#10587,#10588,#10589,#10590,#10591,#10592,#10593,#10594,#10595,
#10596,#10597,#10598,#10599,#10600),.UNSPECIFIED.,.F.,.F.)
B_SPLINE_CURVE_WITH_KNOTS((6,1,1,1,1,1,1,1,1,1,1,1,1,1,1,1,1,1,1,1,1,1,
1,1,1,1,1,1,1,1,6),(0.,0.0333333333333333,0.0666666666666667,0.1,0.133333333333333,
0.166666666666667,0.2,0.233333333333333,0.266666666666667,0.3,0.333333333333333,
0.366666666666667,0.4,0.433333333333333,0.466666666666667,0.5,0.533333333333333,
0.566666666666667,0.6,0.633333333333333,0.666666666666667,0.7,0.733333333333333,
0.766666666666667,0.8,0.833333333333333,0.866666666666667,0.9,0.933333333333333,
0.966666666666667,1.),.UNSPECIFIED.)
CURVE()
GEOMETRIC_REPRESENTATION_ITEM()
RATIONAL_B_SPLINE_CURVE((1.,1.,1.,1.,1.,1.,1.,1.,1.,1.,1.,1.,1.,1.,1.,1.,
1.,1.,1.,1.,1.,1.,1.,1.,1.,1.,1.,1.,1.,1.,1.,1.,1.,1.,1.))
REPRESENTATION_ITEM('')
);
#192=(
BOUNDED_CURVE()
B_SPLINE_CURVE(5,(#10601,#10602,#10603,#10604,#10605,#10606,#10607,#10608,
#10609,#10610,#10611,#10612,#10613,#10614,#10615,#10616,#10617,#10618,#10619,
#10620,#10621,#10622,#10623,#10624,#10625,#10626,#10627,#10628,#10629,#10630,
#10631,#10632,#10633,#10634,#10635),.UNSPECIFIED.,.F.,.F.)
B_SPLINE_CURVE_WITH_KNOTS((6,1,1,1,1,1,1,1,1,1,1,1,1,1,1,1,1,1,1,1,1,1,
1,1,1,1,1,1,1,1,6),(0.,0.0333333333333333,0.0666666666666667,0.1,0.133333333333333,
0.166666666666667,0.2,0.233333333333333,0.266666666666667,0.3,0.333333333333333,
0.366666666666667,0.4,0.433333333333333,0.466666666666667,0.5,0.533333333333333,
0.566666666666667,0.6,0.633333333333333,0.666666666666667,0.7,0.733333333333333,
0.766666666666667,0.8,0.833333333333333,0.866666666666667,0.9,0.933333333333333,
0.966666666666667,1.),.UNSPECIFIED.)
CURVE()
GEOMETRIC_REPRESENTATION_ITEM()
RATIONAL_B_SPLINE_CURVE((1.,1.,1.,1.,1.,1.,1.,1.,1.,1.,1.,1.,1.,1.,1.,1.,
1.,1.,1.,1.,1.,1.,1.,1.,1.,1.,1.,1.,1.,1.,1.,1.,1.,1.,1.))
REPRESENTATION_ITEM('')
);
#193=(
BOUNDED_CURVE()
B_SPLINE_CURVE(5,(#10637,#10638,#10639,#10640,#10641,#10642,#10643,#10644,
#10645,#10646,#10647,#10648,#10649,#10650,#10651,#10652,#10653,#10654,#10655,
#10656,#10657,#10658,#10659,#10660,#10661,#10662,#10663,#10664,#10665,#10666,
#10667,#10668,#10669,#10670,#10671),.UNSPECIFIED.,.F.,.F.)
B_SPLINE_CURVE_WITH_KNOTS((6,1,1,1,1,1,1,1,1,1,1,1,1,1,1,1,1,1,1,1,1,1,
1,1,1,1,1,1,1,1,6),(0.,0.0333333333333333,0.0666666666666667,0.1,0.133333333333333,
0.166666666666667,0.2,0.233333333333333,0.266666666666667,0.3,0.333333333333333,
0.366666666666667,0.4,0.433333333333333,0.466666666666667,0.5,0.533333333333333,
0.566666666666667,0.6,0.633333333333333,0.666666666666667,0.7,0.733333333333333,
0.766666666666667,0.8,0.833333333333333,0.866666666666667,0.9,0.933333333333333,
0.966666666666667,1.),.UNSPECIFIED.)
CURVE()
GEOMETRIC_REPRESENTATION_ITEM()
RATIONAL_B_SPLINE_CURVE((1.,1.,1.,1.,1.,1.,1.,1.,1.,1.,1.,1.,1.,1.,1.,1.,
1.,1.,1.,1.,1.,1.,1.,1.,1.,1.,1.,1.,1.,1.,1.,1.,1.,1.,1.))
REPRESENTATION_ITEM('')
);
#194=(
BOUNDED_CURVE()
B_SPLINE_CURVE(5,(#10673,#10674,#10675,#10676,#10677,#10678,#10679,#10680,
#10681,#10682,#10683,#10684,#10685,#10686,#10687,#10688,#10689,#10690,#10691,
#10692,#10693,#10694,#10695,#10696,#10697,#10698,#10699,#10700,#10701,#10702,
#10703,#10704,#10705,#10706,#10707),.UNSPECIFIED.,.F.,.F.)
B_SPLINE_CURVE_WITH_KNOTS((6,1,1,1,1,1,1,1,1,1,1,1,1,1,1,1,1,1,1,1,1,1,
1,1,1,1,1,1,1,1,6),(0.,0.0333333333333333,0.0666666666666667,0.1,0.133333333333333,
0.166666666666667,0.2,0.233333333333333,0.266666666666667,0.3,0.333333333333333,
0.366666666666667,0.4,0.433333333333333,0.466666666666667,0.5,0.533333333333333,
0.566666666666667,0.6,0.633333333333333,0.666666666666667,0.7,0.733333333333333,
0.766666666666667,0.8,0.833333333333333,0.866666666666667,0.9,0.933333333333333,
0.966666666666667,1.),.UNSPECIFIED.)
CURVE()
GEOMETRIC_REPRESENTATION_ITEM()
RATIONAL_B_SPLINE_CURVE((1.,1.,1.,1.,1.,1.,1.,1.,1.,1.,1.,1.,1.,1.,1.,1.,
1.,1.,1.,1.,1.,1.,1.,1.,1.,1.,1.,1.,1.,1.,1.,1.,1.,1.,1.))
REPRESENTATION_ITEM('')
);
#195=(
BOUNDED_CURVE()
B_SPLINE_CURVE(5,(#10711,#10712,#10713,#10714,#10715,#10716,#10717,#10718,
#10719,#10720,#10721,#10722,#10723,#10724,#10725,#10726,#10727,#10728,#10729,
#10730,#10731,#10732,#10733,#10734,#10735,#10736,#10737,#10738,#10739,#10740,
#10741,#10742,#10743,#10744,#10745),.UNSPECIFIED.,.F.,.F.)
B_SPLINE_CURVE_WITH_KNOTS((6,1,1,1,1,1,1,1,1,1,1,1,1,1,1,1,1,1,1,1,1,1,
1,1,1,1,1,1,1,1,6),(0.,0.0333333333333333,0.0666666666666667,0.1,0.133333333333333,
0.166666666666667,0.2,0.233333333333333,0.266666666666667,0.3,0.333333333333333,
0.366666666666667,0.4,0.433333333333333,0.466666666666667,0.5,0.533333333333333,
0.566666666666667,0.6,0.633333333333333,0.666666666666667,0.7,0.733333333333333,
0.766666666666667,0.8,0.833333333333333,0.866666666666667,0.9,0.933333333333333,
0.966666666666667,1.),.UNSPECIFIED.)
CURVE()
GEOMETRIC_REPRESENTATION_ITEM()
RATIONAL_B_SPLINE_CURVE((1.,1.,1.,1.,1.,1.,1.,1.,1.,1.,1.,1.,1.,1.,1.,1.,
1.,1.,1.,1.,1.,1.,1.,1.,1.,1.,1.,1.,1.,1.,1.,1.,1.,1.,1.))
REPRESENTATION_ITEM('')
);
#196=(
BOUNDED_CURVE()
B_SPLINE_CURVE(5,(#10747,#10748,#10749,#10750,#10751,#10752,#10753,#10754,
#10755,#10756,#10757,#10758,#10759,#10760,#10761,#10762,#10763,#10764,#10765,
#10766,#10767,#10768,#10769,#10770,#10771,#10772,#10773,#10774,#10775,#10776,
#10777,#10778,#10779,#10780,#10781),.UNSPECIFIED.,.F.,.F.)
B_SPLINE_CURVE_WITH_KNOTS((6,1,1,1,1,1,1,1,1,1,1,1,1,1,1,1,1,1,1,1,1,1,
1,1,1,1,1,1,1,1,6),(0.,0.0333333333333333,0.0666666666666667,0.1,0.133333333333333,
0.166666666666667,0.2,0.233333333333333,0.266666666666667,0.3,0.333333333333333,
0.366666666666667,0.4,0.433333333333333,0.466666666666667,0.5,0.533333333333333,
0.566666666666667,0.6,0.633333333333333,0.666666666666667,0.7,0.733333333333333,
0.766666666666667,0.8,0.833333333333333,0.866666666666667,0.9,0.933333333333333,
0.966666666666667,1.),.UNSPECIFIED.)
CURVE()
GEOMETRIC_REPRESENTATION_ITEM()
RATIONAL_B_SPLINE_CURVE((1.,1.,1.,1.,1.,1.,1.,1.,1.,1.,1.,1.,1.,1.,1.,1.,
1.,1.,1.,1.,1.,1.,1.,1.,1.,1.,1.,1.,1.,1.,1.,1.,1.,1.,1.))
REPRESENTATION_ITEM('')
);
#197=(
BOUNDED_CURVE()
B_SPLINE_CURVE(5,(#10785,#10786,#10787,#10788,#10789,#10790,#10791,#10792,
#10793,#10794,#10795,#10796,#10797,#10798,#10799,#10800,#10801,#10802,#10803,
#10804,#10805,#10806,#10807,#10808,#10809,#10810,#10811,#10812,#10813,#10814,
#10815,#10816,#10817,#10818,#10819),.UNSPECIFIED.,.F.,.F.)
B_SPLINE_CURVE_WITH_KNOTS((6,1,1,1,1,1,1,1,1,1,1,1,1,1,1,1,1,1,1,1,1,1,
1,1,1,1,1,1,1,1,6),(0.,0.0333333333333333,0.0666666666666667,0.1,0.133333333333333,
0.166666666666667,0.2,0.233333333333333,0.266666666666667,0.3,0.333333333333333,
0.366666666666667,0.4,0.433333333333333,0.466666666666667,0.5,0.533333333333333,
0.566666666666667,0.6,0.633333333333333,0.666666666666667,0.7,0.733333333333333,
0.766666666666667,0.8,0.833333333333333,0.866666666666667,0.9,0.933333333333333,
0.966666666666667,1.),.UNSPECIFIED.)
CURVE()
GEOMETRIC_REPRESENTATION_ITEM()
RATIONAL_B_SPLINE_CURVE((1.,1.,1.,1.,1.,1.,1.,1.,1.,1.,1.,1.,1.,1.,1.,1.,
1.,1.,1.,1.,1.,1.,1.,1.,1.,1.,1.,1.,1.,1.,1.,1.,1.,1.,1.))
REPRESENTATION_ITEM('')
);
#198=(
BOUNDED_CURVE()
B_SPLINE_CURVE(5,(#10821,#10822,#10823,#10824,#10825,#10826,#10827,#10828,
#10829,#10830,#10831,#10832,#10833,#10834,#10835,#10836,#10837,#10838,#10839,
#10840,#10841,#10842,#10843,#10844,#10845,#10846,#10847,#10848,#10849,#10850,
#10851,#10852,#10853,#10854,#10855),.UNSPECIFIED.,.F.,.F.)
B_SPLINE_CURVE_WITH_KNOTS((6,1,1,1,1,1,1,1,1,1,1,1,1,1,1,1,1,1,1,1,1,1,
1,1,1,1,1,1,1,1,6),(0.,0.0333333333333333,0.0666666666666667,0.1,0.133333333333333,
0.166666666666667,0.2,0.233333333333333,0.266666666666667,0.3,0.333333333333333,
0.366666666666667,0.4,0.433333333333333,0.466666666666667,0.5,0.533333333333333,
0.566666666666667,0.6,0.633333333333333,0.666666666666667,0.7,0.733333333333333,
0.766666666666667,0.8,0.833333333333333,0.866666666666667,0.9,0.933333333333333,
0.966666666666667,1.),.UNSPECIFIED.)
CURVE()
GEOMETRIC_REPRESENTATION_ITEM()
RATIONAL_B_SPLINE_CURVE((1.,1.,1.,1.,1.,1.,1.,1.,1.,1.,1.,1.,1.,1.,1.,1.,
1.,1.,1.,1.,1.,1.,1.,1.,1.,1.,1.,1.,1.,1.,1.,1.,1.,1.,1.))
REPRESENTATION_ITEM('')
);
#199=(
BOUNDED_CURVE()
B_SPLINE_CURVE(5,(#10859,#10860,#10861,#10862,#10863,#10864,#10865,#10866,
#10867,#10868,#10869,#10870,#10871,#10872,#10873,#10874,#10875,#10876,#10877,
#10878,#10879,#10880,#10881,#10882,#10883,#10884,#10885,#10886,#10887,#10888,
#10889,#10890,#10891,#10892,#10893),.UNSPECIFIED.,.F.,.F.)
B_SPLINE_CURVE_WITH_KNOTS((6,1,1,1,1,1,1,1,1,1,1,1,1,1,1,1,1,1,1,1,1,1,
1,1,1,1,1,1,1,1,6),(0.,0.0333333333333333,0.0666666666666667,0.1,0.133333333333333,
0.166666666666667,0.2,0.233333333333333,0.266666666666667,0.3,0.333333333333333,
0.366666666666667,0.4,0.433333333333333,0.466666666666667,0.5,0.533333333333333,
0.566666666666667,0.6,0.633333333333333,0.666666666666667,0.7,0.733333333333333,
0.766666666666667,0.8,0.833333333333333,0.866666666666667,0.9,0.933333333333333,
0.966666666666667,1.),.UNSPECIFIED.)
CURVE()
GEOMETRIC_REPRESENTATION_ITEM()
RATIONAL_B_SPLINE_CURVE((1.,1.,1.,1.,1.,1.,1.,1.,1.,1.,1.,1.,1.,1.,1.,1.,
1.,1.,1.,1.,1.,1.,1.,1.,1.,1.,1.,1.,1.,1.,1.,1.,1.,1.,1.))
REPRESENTATION_ITEM('')
);
#200=(
BOUNDED_CURVE()
B_SPLINE_CURVE(5,(#10895,#10896,#10897,#10898,#10899,#10900,#10901,#10902,
#10903,#10904,#10905,#10906,#10907,#10908,#10909,#10910,#10911,#10912,#10913,
#10914,#10915,#10916,#10917,#10918,#10919,#10920,#10921,#10922,#10923,#10924,
#10925,#10926,#10927,#10928,#10929),.UNSPECIFIED.,.F.,.F.)
B_SPLINE_CURVE_WITH_KNOTS((6,1,1,1,1,1,1,1,1,1,1,1,1,1,1,1,1,1,1,1,1,1,
1,1,1,1,1,1,1,1,6),(0.,0.0333333333333333,0.0666666666666667,0.1,0.133333333333333,
0.166666666666667,0.2,0.233333333333333,0.266666666666667,0.3,0.333333333333333,
0.366666666666667,0.4,0.433333333333333,0.466666666666667,0.5,0.533333333333333,
0.566666666666667,0.6,0.633333333333333,0.666666666666667,0.7,0.733333333333333,
0.766666666666667,0.8,0.833333333333333,0.866666666666667,0.9,0.933333333333333,
0.966666666666667,1.),.UNSPECIFIED.)
CURVE()
GEOMETRIC_REPRESENTATION_ITEM()
RATIONAL_B_SPLINE_CURVE((1.,1.,1.,1.,1.,1.,1.,1.,1.,1.,1.,1.,1.,1.,1.,1.,
1.,1.,1.,1.,1.,1.,1.,1.,1.,1.,1.,1.,1.,1.,1.,1.,1.,1.,1.))
REPRESENTATION_ITEM('')
);
#201=(
BOUNDED_CURVE()
B_SPLINE_CURVE(5,(#10933,#10934,#10935,#10936,#10937,#10938,#10939,#10940,
#10941,#10942,#10943,#10944,#10945,#10946,#10947,#10948,#10949,#10950,#10951,
#10952,#10953,#10954,#10955,#10956,#10957,#10958,#10959,#10960,#10961,#10962,
#10963,#10964,#10965,#10966,#10967),.UNSPECIFIED.,.F.,.F.)
B_SPLINE_CURVE_WITH_KNOTS((6,1,1,1,1,1,1,1,1,1,1,1,1,1,1,1,1,1,1,1,1,1,
1,1,1,1,1,1,1,1,6),(0.,0.0333333333333333,0.0666666666666667,0.1,0.133333333333333,
0.166666666666667,0.2,0.233333333333333,0.266666666666667,0.3,0.333333333333333,
0.366666666666667,0.4,0.433333333333333,0.466666666666667,0.5,0.533333333333333,
0.566666666666667,0.6,0.633333333333333,0.666666666666667,0.7,0.733333333333333,
0.766666666666667,0.8,0.833333333333333,0.866666666666667,0.9,0.933333333333333,
0.966666666666667,1.),.UNSPECIFIED.)
CURVE()
GEOMETRIC_REPRESENTATION_ITEM()
RATIONAL_B_SPLINE_CURVE((1.,1.,1.,1.,1.,1.,1.,1.,1.,1.,1.,1.,1.,1.,1.,1.,
1.,1.,1.,1.,1.,1.,1.,1.,1.,1.,1.,1.,1.,1.,1.,1.,1.,1.,1.))
REPRESENTATION_ITEM('')
);
#202=(
BOUNDED_CURVE()
B_SPLINE_CURVE(5,(#10969,#10970,#10971,#10972,#10973,#10974,#10975,#10976,
#10977,#10978,#10979,#10980,#10981,#10982,#10983,#10984,#10985,#10986,#10987,
#10988,#10989,#10990,#10991,#10992,#10993,#10994,#10995,#10996,#10997,#10998,
#10999,#11000,#11001,#11002,#11003),.UNSPECIFIED.,.F.,.F.)
B_SPLINE_CURVE_WITH_KNOTS((6,1,1,1,1,1,1,1,1,1,1,1,1,1,1,1,1,1,1,1,1,1,
1,1,1,1,1,1,1,1,6),(0.,0.0333333333333333,0.0666666666666667,0.1,0.133333333333333,
0.166666666666667,0.2,0.233333333333333,0.266666666666667,0.3,0.333333333333333,
0.366666666666667,0.4,0.433333333333333,0.466666666666667,0.5,0.533333333333333,
0.566666666666667,0.6,0.633333333333333,0.666666666666667,0.7,0.733333333333333,
0.766666666666667,0.8,0.833333333333333,0.866666666666667,0.9,0.933333333333333,
0.966666666666667,1.),.UNSPECIFIED.)
CURVE()
GEOMETRIC_REPRESENTATION_ITEM()
RATIONAL_B_SPLINE_CURVE((1.,1.,1.,1.,1.,1.,1.,1.,1.,1.,1.,1.,1.,1.,1.,1.,
1.,1.,1.,1.,1.,1.,1.,1.,1.,1.,1.,1.,1.,1.,1.,1.,1.,1.,1.))
REPRESENTATION_ITEM('')
);
#203=(
BOUNDED_CURVE()
B_SPLINE_CURVE(5,(#11007,#11008,#11009,#11010,#11011,#11012,#11013,#11014,
#11015,#11016,#11017,#11018,#11019,#11020,#11021,#11022,#11023,#11024,#11025,
#11026,#11027,#11028,#11029,#11030,#11031,#11032,#11033,#11034,#11035,#11036,
#11037,#11038,#11039,#11040,#11041),.UNSPECIFIED.,.F.,.F.)
B_SPLINE_CURVE_WITH_KNOTS((6,1,1,1,1,1,1,1,1,1,1,1,1,1,1,1,1,1,1,1,1,1,
1,1,1,1,1,1,1,1,6),(0.,0.0333333333333333,0.0666666666666667,0.1,0.133333333333333,
0.166666666666667,0.2,0.233333333333333,0.266666666666667,0.3,0.333333333333333,
0.366666666666667,0.4,0.433333333333333,0.466666666666667,0.5,0.533333333333333,
0.566666666666667,0.6,0.633333333333333,0.666666666666667,0.7,0.733333333333333,
0.766666666666667,0.8,0.833333333333333,0.866666666666667,0.9,0.933333333333333,
0.966666666666667,1.),.UNSPECIFIED.)
CURVE()
GEOMETRIC_REPRESENTATION_ITEM()
RATIONAL_B_SPLINE_CURVE((1.,1.,1.,1.,1.,1.,1.,1.,1.,1.,1.,1.,1.,1.,1.,1.,
1.,1.,1.,1.,1.,1.,1.,1.,1.,1.,1.,1.,1.,1.,1.,1.,1.,1.,1.))
REPRESENTATION_ITEM('')
);
#204=(
BOUNDED_CURVE()
B_SPLINE_CURVE(5,(#11043,#11044,#11045,#11046,#11047,#11048,#11049,#11050,
#11051,#11052,#11053,#11054,#11055,#11056,#11057,#11058,#11059,#11060,#11061,
#11062,#11063,#11064,#11065,#11066,#11067,#11068,#11069,#11070,#11071,#11072,
#11073,#11074,#11075,#11076,#11077),.UNSPECIFIED.,.F.,.F.)
B_SPLINE_CURVE_WITH_KNOTS((6,1,1,1,1,1,1,1,1,1,1,1,1,1,1,1,1,1,1,1,1,1,
1,1,1,1,1,1,1,1,6),(0.,0.0333333333333333,0.0666666666666667,0.1,0.133333333333333,
0.166666666666667,0.2,0.233333333333333,0.266666666666667,0.3,0.333333333333333,
0.366666666666667,0.4,0.433333333333333,0.466666666666667,0.5,0.533333333333333,
0.566666666666667,0.6,0.633333333333333,0.666666666666667,0.7,0.733333333333333,
0.766666666666667,0.8,0.833333333333333,0.866666666666667,0.9,0.933333333333333,
0.966666666666667,1.),.UNSPECIFIED.)
CURVE()
GEOMETRIC_REPRESENTATION_ITEM()
RATIONAL_B_SPLINE_CURVE((1.,1.,1.,1.,1.,1.,1.,1.,1.,1.,1.,1.,1.,1.,1.,1.,
1.,1.,1.,1.,1.,1.,1.,1.,1.,1.,1.,1.,1.,1.,1.,1.,1.,1.,1.))
REPRESENTATION_ITEM('')
);
#205=(
BOUNDED_CURVE()
B_SPLINE_CURVE(5,(#11081,#11082,#11083,#11084,#11085,#11086,#11087,#11088,
#11089,#11090,#11091,#11092,#11093,#11094,#11095,#11096,#11097,#11098,#11099,
#11100,#11101,#11102,#11103,#11104,#11105,#11106,#11107,#11108,#11109,#11110,
#11111,#11112,#11113,#11114,#11115),.UNSPECIFIED.,.F.,.F.)
B_SPLINE_CURVE_WITH_KNOTS((6,1,1,1,1,1,1,1,1,1,1,1,1,1,1,1,1,1,1,1,1,1,
1,1,1,1,1,1,1,1,6),(0.,0.0333333333333333,0.0666666666666667,0.1,0.133333333333333,
0.166666666666667,0.2,0.233333333333333,0.266666666666667,0.3,0.333333333333333,
0.366666666666667,0.4,0.433333333333333,0.466666666666667,0.5,0.533333333333333,
0.566666666666667,0.6,0.633333333333333,0.666666666666667,0.7,0.733333333333333,
0.766666666666667,0.8,0.833333333333333,0.866666666666667,0.9,0.933333333333333,
0.966666666666667,1.),.UNSPECIFIED.)
CURVE()
GEOMETRIC_REPRESENTATION_ITEM()
RATIONAL_B_SPLINE_CURVE((1.,1.,1.,1.,1.,1.,1.,1.,1.,1.,1.,1.,1.,1.,1.,1.,
1.,1.,1.,1.,1.,1.,1.,1.,1.,1.,1.,1.,1.,1.,1.,1.,1.,1.,1.))
REPRESENTATION_ITEM('')
);
#206=(
BOUNDED_CURVE()
B_SPLINE_CURVE(5,(#11117,#11118,#11119,#11120,#11121,#11122,#11123,#11124,
#11125,#11126,#11127,#11128,#11129,#11130,#11131,#11132,#11133,#11134,#11135,
#11136,#11137,#11138,#11139,#11140,#11141,#11142,#11143,#11144,#11145,#11146,
#11147,#11148,#11149,#11150,#11151),.UNSPECIFIED.,.F.,.F.)
B_SPLINE_CURVE_WITH_KNOTS((6,1,1,1,1,1,1,1,1,1,1,1,1,1,1,1,1,1,1,1,1,1,
1,1,1,1,1,1,1,1,6),(0.,0.0333333333333333,0.0666666666666667,0.1,0.133333333333333,
0.166666666666667,0.2,0.233333333333333,0.266666666666667,0.3,0.333333333333333,
0.366666666666667,0.4,0.433333333333333,0.466666666666667,0.5,0.533333333333333,
0.566666666666667,0.6,0.633333333333333,0.666666666666667,0.7,0.733333333333333,
0.766666666666667,0.8,0.833333333333333,0.866666666666667,0.9,0.933333333333333,
0.966666666666667,1.),.UNSPECIFIED.)
CURVE()
GEOMETRIC_REPRESENTATION_ITEM()
RATIONAL_B_SPLINE_CURVE((1.,1.,1.,1.,1.,1.,1.,1.,1.,1.,1.,1.,1.,1.,1.,1.,
1.,1.,1.,1.,1.,1.,1.,1.,1.,1.,1.,1.,1.,1.,1.,1.,1.,1.,1.))
REPRESENTATION_ITEM('')
);
#207=(
BOUNDED_CURVE()
B_SPLINE_CURVE(5,(#11155,#11156,#11157,#11158,#11159,#11160,#11161,#11162,
#11163,#11164,#11165,#11166,#11167,#11168,#11169,#11170,#11171,#11172,#11173,
#11174,#11175,#11176,#11177,#11178,#11179,#11180,#11181,#11182,#11183,#11184,
#11185,#11186,#11187,#11188,#11189),.UNSPECIFIED.,.F.,.F.)
B_SPLINE_CURVE_WITH_KNOTS((6,1,1,1,1,1,1,1,1,1,1,1,1,1,1,1,1,1,1,1,1,1,
1,1,1,1,1,1,1,1,6),(0.,0.0333333333333333,0.0666666666666667,0.1,0.133333333333333,
0.166666666666667,0.2,0.233333333333333,0.266666666666667,0.3,0.333333333333333,
0.366666666666667,0.4,0.433333333333333,0.466666666666667,0.5,0.533333333333333,
0.566666666666667,0.6,0.633333333333333,0.666666666666667,0.7,0.733333333333333,
0.766666666666667,0.8,0.833333333333333,0.866666666666667,0.9,0.933333333333333,
0.966666666666667,1.),.UNSPECIFIED.)
CURVE()
GEOMETRIC_REPRESENTATION_ITEM()
RATIONAL_B_SPLINE_CURVE((1.,1.,1.,1.,1.,1.,1.,1.,1.,1.,1.,1.,1.,1.,1.,1.,
1.,1.,1.,1.,1.,1.,1.,1.,1.,1.,1.,1.,1.,1.,1.,1.,1.,1.,1.))
REPRESENTATION_ITEM('')
);
#208=(
BOUNDED_CURVE()
B_SPLINE_CURVE(5,(#11191,#11192,#11193,#11194,#11195,#11196,#11197,#11198,
#11199,#11200,#11201,#11202,#11203,#11204,#11205,#11206,#11207,#11208,#11209,
#11210,#11211,#11212,#11213,#11214,#11215,#11216,#11217,#11218,#11219,#11220,
#11221,#11222,#11223,#11224,#11225),.UNSPECIFIED.,.F.,.F.)
B_SPLINE_CURVE_WITH_KNOTS((6,1,1,1,1,1,1,1,1,1,1,1,1,1,1,1,1,1,1,1,1,1,
1,1,1,1,1,1,1,1,6),(0.,0.0333333333333333,0.0666666666666667,0.1,0.133333333333333,
0.166666666666667,0.2,0.233333333333333,0.266666666666667,0.3,0.333333333333333,
0.366666666666667,0.4,0.433333333333333,0.466666666666667,0.5,0.533333333333333,
0.566666666666667,0.6,0.633333333333333,0.666666666666667,0.7,0.733333333333333,
0.766666666666667,0.8,0.833333333333333,0.866666666666667,0.9,0.933333333333333,
0.966666666666667,1.),.UNSPECIFIED.)
CURVE()
GEOMETRIC_REPRESENTATION_ITEM()
RATIONAL_B_SPLINE_CURVE((1.,1.,1.,1.,1.,1.,1.,1.,1.,1.,1.,1.,1.,1.,1.,1.,
1.,1.,1.,1.,1.,1.,1.,1.,1.,1.,1.,1.,1.,1.,1.,1.,1.,1.,1.))
REPRESENTATION_ITEM('')
);
#209=(
BOUNDED_CURVE()
B_SPLINE_CURVE(5,(#11229,#11230,#11231,#11232,#11233,#11234,#11235,#11236,
#11237,#11238,#11239,#11240,#11241,#11242,#11243,#11244,#11245,#11246,#11247,
#11248,#11249,#11250,#11251,#11252,#11253,#11254,#11255,#11256,#11257,#11258,
#11259,#11260,#11261,#11262,#11263),.UNSPECIFIED.,.F.,.F.)
B_SPLINE_CURVE_WITH_KNOTS((6,1,1,1,1,1,1,1,1,1,1,1,1,1,1,1,1,1,1,1,1,1,
1,1,1,1,1,1,1,1,6),(0.,0.0333333333333333,0.0666666666666667,0.1,0.133333333333333,
0.166666666666667,0.2,0.233333333333333,0.266666666666667,0.3,0.333333333333333,
0.366666666666667,0.4,0.433333333333333,0.466666666666667,0.5,0.533333333333333,
0.566666666666667,0.6,0.633333333333333,0.666666666666667,0.7,0.733333333333333,
0.766666666666667,0.8,0.833333333333333,0.866666666666667,0.9,0.933333333333333,
0.966666666666667,1.),.UNSPECIFIED.)
CURVE()
GEOMETRIC_REPRESENTATION_ITEM()
RATIONAL_B_SPLINE_CURVE((1.,1.,1.,1.,1.,1.,1.,1.,1.,1.,1.,1.,1.,1.,1.,1.,
1.,1.,1.,1.,1.,1.,1.,1.,1.,1.,1.,1.,1.,1.,1.,1.,1.,1.,1.))
REPRESENTATION_ITEM('')
);
#210=(
BOUNDED_CURVE()
B_SPLINE_CURVE(5,(#11265,#11266,#11267,#11268,#11269,#11270,#11271,#11272,
#11273,#11274,#11275,#11276,#11277,#11278,#11279,#11280,#11281,#11282,#11283,
#11284,#11285,#11286,#11287,#11288,#11289,#11290,#11291,#11292,#11293,#11294,
#11295,#11296,#11297,#11298,#11299),.UNSPECIFIED.,.F.,.F.)
B_SPLINE_CURVE_WITH_KNOTS((6,1,1,1,1,1,1,1,1,1,1,1,1,1,1,1,1,1,1,1,1,1,
1,1,1,1,1,1,1,1,6),(0.,0.0333333333333333,0.0666666666666667,0.1,0.133333333333333,
0.166666666666667,0.2,0.233333333333333,0.266666666666667,0.3,0.333333333333333,
0.366666666666667,0.4,0.433333333333333,0.466666666666667,0.5,0.533333333333333,
0.566666666666667,0.6,0.633333333333333,0.666666666666667,0.7,0.733333333333333,
0.766666666666667,0.8,0.833333333333333,0.866666666666667,0.9,0.933333333333333,
0.966666666666667,1.),.UNSPECIFIED.)
CURVE()
GEOMETRIC_REPRESENTATION_ITEM()
RATIONAL_B_SPLINE_CURVE((1.,1.,1.,1.,1.,1.,1.,1.,1.,1.,1.,1.,1.,1.,1.,1.,
1.,1.,1.,1.,1.,1.,1.,1.,1.,1.,1.,1.,1.,1.,1.,1.,1.,1.,1.))
REPRESENTATION_ITEM('')
);
#211=(
BOUNDED_CURVE()
B_SPLINE_CURVE(5,(#11303,#11304,#11305,#11306,#11307,#11308,#11309,#11310,
#11311,#11312,#11313,#11314,#11315,#11316,#11317,#11318,#11319,#11320,#11321,
#11322,#11323,#11324,#11325,#11326,#11327,#11328,#11329,#11330,#11331,#11332,
#11333,#11334,#11335,#11336,#11337),.UNSPECIFIED.,.F.,.F.)
B_SPLINE_CURVE_WITH_KNOTS((6,1,1,1,1,1,1,1,1,1,1,1,1,1,1,1,1,1,1,1,1,1,
1,1,1,1,1,1,1,1,6),(0.,0.0333333333333333,0.0666666666666667,0.1,0.133333333333333,
0.166666666666667,0.2,0.233333333333333,0.266666666666667,0.3,0.333333333333333,
0.366666666666667,0.4,0.433333333333333,0.466666666666667,0.5,0.533333333333333,
0.566666666666667,0.6,0.633333333333333,0.666666666666667,0.7,0.733333333333333,
0.766666666666667,0.8,0.833333333333333,0.866666666666667,0.9,0.933333333333333,
0.966666666666667,1.),.UNSPECIFIED.)
CURVE()
GEOMETRIC_REPRESENTATION_ITEM()
RATIONAL_B_SPLINE_CURVE((1.,1.,1.,1.,1.,1.,1.,1.,1.,1.,1.,1.,1.,1.,1.,1.,
1.,1.,1.,1.,1.,1.,1.,1.,1.,1.,1.,1.,1.,1.,1.,1.,1.,1.,1.))
REPRESENTATION_ITEM('')
);
#212=(
BOUNDED_CURVE()
B_SPLINE_CURVE(5,(#11339,#11340,#11341,#11342,#11343,#11344,#11345,#11346,
#11347,#11348,#11349,#11350,#11351,#11352,#11353,#11354,#11355,#11356,#11357,
#11358,#11359,#11360,#11361,#11362,#11363,#11364,#11365,#11366,#11367,#11368,
#11369,#11370,#11371,#11372,#11373),.UNSPECIFIED.,.F.,.F.)
B_SPLINE_CURVE_WITH_KNOTS((6,1,1,1,1,1,1,1,1,1,1,1,1,1,1,1,1,1,1,1,1,1,
1,1,1,1,1,1,1,1,6),(0.,0.0333333333333333,0.0666666666666667,0.1,0.133333333333333,
0.166666666666667,0.2,0.233333333333333,0.266666666666667,0.3,0.333333333333333,
0.366666666666667,0.4,0.433333333333333,0.466666666666667,0.5,0.533333333333333,
0.566666666666667,0.6,0.633333333333333,0.666666666666667,0.7,0.733333333333333,
0.766666666666667,0.8,0.833333333333333,0.866666666666667,0.9,0.933333333333333,
0.966666666666667,1.),.UNSPECIFIED.)
CURVE()
GEOMETRIC_REPRESENTATION_ITEM()
RATIONAL_B_SPLINE_CURVE((1.,1.,1.,1.,1.,1.,1.,1.,1.,1.,1.,1.,1.,1.,1.,1.,
1.,1.,1.,1.,1.,1.,1.,1.,1.,1.,1.,1.,1.,1.,1.,1.,1.,1.,1.))
REPRESENTATION_ITEM('')
);
#213=(
BOUNDED_CURVE()
B_SPLINE_CURVE(5,(#11377,#11378,#11379,#11380,#11381,#11382,#11383,#11384,
#11385,#11386,#11387,#11388,#11389,#11390,#11391,#11392,#11393,#11394,#11395,
#11396,#11397,#11398,#11399,#11400,#11401,#11402,#11403,#11404,#11405,#11406,
#11407,#11408,#11409,#11410,#11411),.UNSPECIFIED.,.F.,.F.)
B_SPLINE_CURVE_WITH_KNOTS((6,1,1,1,1,1,1,1,1,1,1,1,1,1,1,1,1,1,1,1,1,1,
1,1,1,1,1,1,1,1,6),(0.,0.0333333333333333,0.0666666666666667,0.1,0.133333333333333,
0.166666666666667,0.2,0.233333333333333,0.266666666666667,0.3,0.333333333333333,
0.366666666666667,0.4,0.433333333333333,0.466666666666667,0.5,0.533333333333333,
0.566666666666667,0.6,0.633333333333333,0.666666666666667,0.7,0.733333333333333,
0.766666666666667,0.8,0.833333333333333,0.866666666666667,0.9,0.933333333333333,
0.966666666666667,1.),.UNSPECIFIED.)
CURVE()
GEOMETRIC_REPRESENTATION_ITEM()
RATIONAL_B_SPLINE_CURVE((1.,1.,1.,1.,1.,1.,1.,1.,1.,1.,1.,1.,1.,1.,1.,1.,
1.,1.,1.,1.,1.,1.,1.,1.,1.,1.,1.,1.,1.,1.,1.,1.,1.,1.,1.))
REPRESENTATION_ITEM('')
);
#214=(
BOUNDED_CURVE()
B_SPLINE_CURVE(5,(#11412,#11413,#11414,#11415,#11416,#11417,#11418,#11419,
#11420,#11421,#11422,#11423,#11424,#11425,#11426,#11427,#11428,#11429,#11430,
#11431,#11432,#11433,#11434,#11435,#11436,#11437,#11438,#11439,#11440,#11441,
#11442,#11443,#11444,#11445,#11446),.UNSPECIFIED.,.F.,.F.)
B_SPLINE_CURVE_WITH_KNOTS((6,1,1,1,1,1,1,1,1,1,1,1,1,1,1,1,1,1,1,1,1,1,
1,1,1,1,1,1,1,1,6),(0.,0.0333333333333333,0.0666666666666667,0.1,0.133333333333333,
0.166666666666667,0.2,0.233333333333333,0.266666666666667,0.3,0.333333333333333,
0.366666666666667,0.4,0.433333333333333,0.466666666666667,0.5,0.533333333333333,
0.566666666666667,0.6,0.633333333333333,0.666666666666667,0.7,0.733333333333333,
0.766666666666667,0.8,0.833333333333333,0.866666666666667,0.9,0.933333333333333,
0.966666666666667,1.),.UNSPECIFIED.)
CURVE()
GEOMETRIC_REPRESENTATION_ITEM()
RATIONAL_B_SPLINE_CURVE((1.,1.,1.,1.,1.,1.,1.,1.,1.,1.,1.,1.,1.,1.,1.,1.,
1.,1.,1.,1.,1.,1.,1.,1.,1.,1.,1.,1.,1.,1.,1.,1.,1.,1.,1.))
REPRESENTATION_ITEM('')
);
#215=(
BOUNDED_CURVE()
B_SPLINE_CURVE(5,(#12149,#12150,#12151,#12152,#12153,#12154),
 .UNSPECIFIED.,.F.,.F.)
B_SPLINE_CURVE_WITH_KNOTS((6,6),(0.,0.0167044419747604),.UNSPECIFIED.)
CURVE()
GEOMETRIC_REPRESENTATION_ITEM()
RATIONAL_B_SPLINE_CURVE((1.,1.,1.,1.,1.,1.))
REPRESENTATION_ITEM('')
);
#216=(
BOUNDED_CURVE()
B_SPLINE_CURVE(5,(#12209,#12210,#12211,#12212,#12213,#12214),
 .UNSPECIFIED.,.F.,.F.)
B_SPLINE_CURVE_WITH_KNOTS((6,6),(0.,0.0167044419747598),.UNSPECIFIED.)
CURVE()
GEOMETRIC_REPRESENTATION_ITEM()
RATIONAL_B_SPLINE_CURVE((1.,1.,1.,1.,1.,1.))
REPRESENTATION_ITEM('')
);
#217=(
BOUNDED_CURVE()
B_SPLINE_CURVE(5,(#12269,#12270,#12271,#12272,#12273,#12274),
 .UNSPECIFIED.,.F.,.F.)
B_SPLINE_CURVE_WITH_KNOTS((6,6),(0.,0.0167044419747601),.UNSPECIFIED.)
CURVE()
GEOMETRIC_REPRESENTATION_ITEM()
RATIONAL_B_SPLINE_CURVE((1.,1.,1.,1.,1.,1.))
REPRESENTATION_ITEM('')
);
#218=(
BOUNDED_CURVE()
B_SPLINE_CURVE(5,(#12329,#12330,#12331,#12332,#12333,#12334),
 .UNSPECIFIED.,.F.,.F.)
B_SPLINE_CURVE_WITH_KNOTS((6,6),(0.,0.0167044419747607),.UNSPECIFIED.)
CURVE()
GEOMETRIC_REPRESENTATION_ITEM()
RATIONAL_B_SPLINE_CURVE((1.,1.,1.,1.,1.,1.))
REPRESENTATION_ITEM('')
);
#219=(
BOUNDED_CURVE()
B_SPLINE_CURVE(5,(#12389,#12390,#12391,#12392,#12393,#12394),
 .UNSPECIFIED.,.F.,.F.)
B_SPLINE_CURVE_WITH_KNOTS((6,6),(0.,0.0167044419747605),.UNSPECIFIED.)
CURVE()
GEOMETRIC_REPRESENTATION_ITEM()
RATIONAL_B_SPLINE_CURVE((1.,1.,1.,1.,1.,1.))
REPRESENTATION_ITEM('')
);
#220=(
BOUNDED_CURVE()
B_SPLINE_CURVE(5,(#12449,#12450,#12451,#12452,#12453,#12454),
 .UNSPECIFIED.,.F.,.F.)
B_SPLINE_CURVE_WITH_KNOTS((6,6),(0.,0.0167044419747612),.UNSPECIFIED.)
CURVE()
GEOMETRIC_REPRESENTATION_ITEM()
RATIONAL_B_SPLINE_CURVE((1.,1.,1.,1.,1.,1.))
REPRESENTATION_ITEM('')
);
#221=(
BOUNDED_CURVE()
B_SPLINE_CURVE(5,(#12509,#12510,#12511,#12512,#12513,#12514),
 .UNSPECIFIED.,.F.,.F.)
B_SPLINE_CURVE_WITH_KNOTS((6,6),(0.,0.01670444197476),.UNSPECIFIED.)
CURVE()
GEOMETRIC_REPRESENTATION_ITEM()
RATIONAL_B_SPLINE_CURVE((1.,1.,1.,1.,1.,1.))
REPRESENTATION_ITEM('')
);
#222=(
BOUNDED_CURVE()
B_SPLINE_CURVE(5,(#12569,#12570,#12571,#12572,#12573,#12574),
 .UNSPECIFIED.,.F.,.F.)
B_SPLINE_CURVE_WITH_KNOTS((6,6),(0.,0.0167044419747599),.UNSPECIFIED.)
CURVE()
GEOMETRIC_REPRESENTATION_ITEM()
RATIONAL_B_SPLINE_CURVE((1.,1.,1.,1.,1.,1.))
REPRESENTATION_ITEM('')
);
#223=(
BOUNDED_CURVE()
B_SPLINE_CURVE(5,(#12629,#12630,#12631,#12632,#12633,#12634),
 .UNSPECIFIED.,.F.,.F.)
B_SPLINE_CURVE_WITH_KNOTS((6,6),(0.,0.01670444197476),.UNSPECIFIED.)
CURVE()
GEOMETRIC_REPRESENTATION_ITEM()
RATIONAL_B_SPLINE_CURVE((1.,1.,1.,1.,1.,1.))
REPRESENTATION_ITEM('')
);
#224=(
BOUNDED_CURVE()
B_SPLINE_CURVE(5,(#12689,#12690,#12691,#12692,#12693,#12694),
 .UNSPECIFIED.,.F.,.F.)
B_SPLINE_CURVE_WITH_KNOTS((6,6),(0.,0.0167044419747604),.UNSPECIFIED.)
CURVE()
GEOMETRIC_REPRESENTATION_ITEM()
RATIONAL_B_SPLINE_CURVE((1.,1.,1.,1.,1.,1.))
REPRESENTATION_ITEM('')
);
#225=(
BOUNDED_CURVE()
B_SPLINE_CURVE(5,(#12725,#12726,#12727,#12728,#12729,#12730),
 .UNSPECIFIED.,.F.,.F.)
B_SPLINE_CURVE_WITH_KNOTS((6,6),(0.,0.0167044419747612),.UNSPECIFIED.)
CURVE()
GEOMETRIC_REPRESENTATION_ITEM()
RATIONAL_B_SPLINE_CURVE((1.,1.,1.,1.,1.,1.))
REPRESENTATION_ITEM('')
);
#226=(
BOUNDED_CURVE()
B_SPLINE_CURVE(5,(#12785,#12786,#12787,#12788,#12789,#12790),
 .UNSPECIFIED.,.F.,.F.)
B_SPLINE_CURVE_WITH_KNOTS((6,6),(0.,0.01670444197476),.UNSPECIFIED.)
CURVE()
GEOMETRIC_REPRESENTATION_ITEM()
RATIONAL_B_SPLINE_CURVE((1.,1.,1.,1.,1.,1.))
REPRESENTATION_ITEM('')
);
#227=(
BOUNDED_CURVE()
B_SPLINE_CURVE(5,(#12845,#12846,#12847,#12848,#12849,#12850),
 .UNSPECIFIED.,.F.,.F.)
B_SPLINE_CURVE_WITH_KNOTS((6,6),(0.,0.0167044419747599),.UNSPECIFIED.)
CURVE()
GEOMETRIC_REPRESENTATION_ITEM()
RATIONAL_B_SPLINE_CURVE((1.,1.,1.,1.,1.,1.))
REPRESENTATION_ITEM('')
);
#228=(
BOUNDED_CURVE()
B_SPLINE_CURVE(5,(#12905,#12906,#12907,#12908,#12909,#12910),
 .UNSPECIFIED.,.F.,.F.)
B_SPLINE_CURVE_WITH_KNOTS((6,6),(0.,0.01670444197476),.UNSPECIFIED.)
CURVE()
GEOMETRIC_REPRESENTATION_ITEM()
RATIONAL_B_SPLINE_CURVE((1.,1.,1.,1.,1.,1.))
REPRESENTATION_ITEM('')
);
#229=(
BOUNDED_CURVE()
B_SPLINE_CURVE(5,(#12965,#12966,#12967,#12968,#12969,#12970),
 .UNSPECIFIED.,.F.,.F.)
B_SPLINE_CURVE_WITH_KNOTS((6,6),(0.,0.0167044419747602),.UNSPECIFIED.)
CURVE()
GEOMETRIC_REPRESENTATION_ITEM()
RATIONAL_B_SPLINE_CURVE((1.,1.,1.,1.,1.,1.))
REPRESENTATION_ITEM('')
);
#230=(
BOUNDED_CURVE()
B_SPLINE_CURVE(5,(#13025,#13026,#13027,#13028,#13029,#13030),
 .UNSPECIFIED.,.F.,.F.)
B_SPLINE_CURVE_WITH_KNOTS((6,6),(0.,0.0167044419747598),.UNSPECIFIED.)
CURVE()
GEOMETRIC_REPRESENTATION_ITEM()
RATIONAL_B_SPLINE_CURVE((1.,1.,1.,1.,1.,1.))
REPRESENTATION_ITEM('')
);
#231=(
BOUNDED_CURVE()
B_SPLINE_CURVE(5,(#13085,#13086,#13087,#13088,#13089,#13090),
 .UNSPECIFIED.,.F.,.F.)
B_SPLINE_CURVE_WITH_KNOTS((6,6),(0.,0.0167044419747605),.UNSPECIFIED.)
CURVE()
GEOMETRIC_REPRESENTATION_ITEM()
RATIONAL_B_SPLINE_CURVE((1.,1.,1.,1.,1.,1.))
REPRESENTATION_ITEM('')
);
#232=(
BOUNDED_CURVE()
B_SPLINE_CURVE(5,(#13145,#13146,#13147,#13148,#13149,#13150),
 .UNSPECIFIED.,.F.,.F.)
B_SPLINE_CURVE_WITH_KNOTS((6,6),(0.,0.0167044419747605),.UNSPECIFIED.)
CURVE()
GEOMETRIC_REPRESENTATION_ITEM()
RATIONAL_B_SPLINE_CURVE((1.,1.,1.,1.,1.,1.))
REPRESENTATION_ITEM('')
);
#233=(
BOUNDED_CURVE()
B_SPLINE_CURVE(5,(#13205,#13206,#13207,#13208,#13209,#13210),
 .UNSPECIFIED.,.F.,.F.)
B_SPLINE_CURVE_WITH_KNOTS((6,6),(0.,0.0167044419747594),.UNSPECIFIED.)
CURVE()
GEOMETRIC_REPRESENTATION_ITEM()
RATIONAL_B_SPLINE_CURVE((1.,1.,1.,1.,1.,1.))
REPRESENTATION_ITEM('')
);
#234=(
BOUNDED_CURVE()
B_SPLINE_CURVE(5,(#13265,#13266,#13267,#13268,#13269,#13270),
 .UNSPECIFIED.,.F.,.F.)
B_SPLINE_CURVE_WITH_KNOTS((6,6),(0.,0.0167044419747601),.UNSPECIFIED.)
CURVE()
GEOMETRIC_REPRESENTATION_ITEM()
RATIONAL_B_SPLINE_CURVE((1.,1.,1.,1.,1.,1.))
REPRESENTATION_ITEM('')
);
#235=(
BOUNDED_CURVE()
B_SPLINE_CURVE(5,(#13382,#13383,#13384,#13385,#13386,#13387),
 .UNSPECIFIED.,.F.,.F.)
B_SPLINE_CURVE_WITH_KNOTS((6,6),(0.984324037881406,1.),.UNSPECIFIED.)
CURVE()
GEOMETRIC_REPRESENTATION_ITEM()
RATIONAL_B_SPLINE_CURVE((1.,1.,1.,1.,1.,1.))
REPRESENTATION_ITEM('')
);
#236=(
BOUNDED_CURVE()
B_SPLINE_CURVE(5,(#14224,#14225,#14226,#14227,#14228,#14229),
 .UNSPECIFIED.,.F.,.F.)
B_SPLINE_CURVE_WITH_KNOTS((6,6),(0.984324037881406,1.),.UNSPECIFIED.)
CURVE()
GEOMETRIC_REPRESENTATION_ITEM()
RATIONAL_B_SPLINE_CURVE((1.,1.,1.,1.,1.,1.))
REPRESENTATION_ITEM('')
);
#237=(
BOUNDED_CURVE()
B_SPLINE_CURVE(5,(#14341,#14342,#14343,#14344,#14345,#14346),
 .UNSPECIFIED.,.F.,.F.)
B_SPLINE_CURVE_WITH_KNOTS((6,6),(0.984324037881405,1.),.UNSPECIFIED.)
CURVE()
GEOMETRIC_REPRESENTATION_ITEM()
RATIONAL_B_SPLINE_CURVE((1.,1.,1.,1.,1.,1.))
REPRESENTATION_ITEM('')
);
#238=(
BOUNDED_CURVE()
B_SPLINE_CURVE(5,(#14396,#14397,#14398,#14399,#14400,#14401),
 .UNSPECIFIED.,.F.,.F.)
B_SPLINE_CURVE_WITH_KNOTS((6,6),(0.984324037881405,1.),.UNSPECIFIED.)
CURVE()
GEOMETRIC_REPRESENTATION_ITEM()
RATIONAL_B_SPLINE_CURVE((1.,1.,1.,1.,1.,1.))
REPRESENTATION_ITEM('')
);
#239=(
BOUNDED_CURVE()
B_SPLINE_CURVE(5,(#14451,#14452,#14453,#14454,#14455,#14456),
 .UNSPECIFIED.,.F.,.F.)
B_SPLINE_CURVE_WITH_KNOTS((6,6),(0.984324037881405,1.),.UNSPECIFIED.)
CURVE()
GEOMETRIC_REPRESENTATION_ITEM()
RATIONAL_B_SPLINE_CURVE((1.,1.,1.,1.,1.,1.))
REPRESENTATION_ITEM('')
);
#240=(
BOUNDED_CURVE()
B_SPLINE_CURVE(5,(#14568,#14569,#14570,#14571,#14572,#14573),
 .UNSPECIFIED.,.F.,.F.)
B_SPLINE_CURVE_WITH_KNOTS((6,6),(0.984324037881406,1.),.UNSPECIFIED.)
CURVE()
GEOMETRIC_REPRESENTATION_ITEM()
RATIONAL_B_SPLINE_CURVE((1.,1.,1.,1.,1.,1.))
REPRESENTATION_ITEM('')
);
#241=(
BOUNDED_CURVE()
B_SPLINE_CURVE(5,(#14685,#14686,#14687,#14688,#14689,#14690),
 .UNSPECIFIED.,.F.,.F.)
B_SPLINE_CURVE_WITH_KNOTS((6,6),(0.984324037881406,1.),.UNSPECIFIED.)
CURVE()
GEOMETRIC_REPRESENTATION_ITEM()
RATIONAL_B_SPLINE_CURVE((1.,1.,1.,1.,1.,1.))
REPRESENTATION_ITEM('')
);
#242=(
BOUNDED_CURVE()
B_SPLINE_CURVE(5,(#14802,#14803,#14804,#14805,#14806,#14807),
 .UNSPECIFIED.,.F.,.F.)
B_SPLINE_CURVE_WITH_KNOTS((6,6),(0.984324037881406,1.),.UNSPECIFIED.)
CURVE()
GEOMETRIC_REPRESENTATION_ITEM()
RATIONAL_B_SPLINE_CURVE((1.,1.,1.,1.,1.,1.))
REPRESENTATION_ITEM('')
);
#243=(
BOUNDED_CURVE()
B_SPLINE_CURVE(5,(#14857,#14858,#14859,#14860,#14861,#14862),
 .UNSPECIFIED.,.F.,.F.)
B_SPLINE_CURVE_WITH_KNOTS((6,6),(0.984324037881405,1.),.UNSPECIFIED.)
CURVE()
GEOMETRIC_REPRESENTATION_ITEM()
RATIONAL_B_SPLINE_CURVE((1.,1.,1.,1.,1.,1.))
REPRESENTATION_ITEM('')
);
#244=(
BOUNDED_CURVE()
B_SPLINE_CURVE(5,(#14912,#14913,#14914,#14915,#14916,#14917),
 .UNSPECIFIED.,.F.,.F.)
B_SPLINE_CURVE_WITH_KNOTS((6,6),(0.984324037881405,1.),.UNSPECIFIED.)
CURVE()
GEOMETRIC_REPRESENTATION_ITEM()
RATIONAL_B_SPLINE_CURVE((1.,1.,1.,1.,1.,1.))
REPRESENTATION_ITEM('')
);
#245=(
BOUNDED_CURVE()
B_SPLINE_CURVE(5,(#15029,#15030,#15031,#15032,#15033,#15034),
 .UNSPECIFIED.,.F.,.F.)
B_SPLINE_CURVE_WITH_KNOTS((6,6),(0.984324037881406,1.),.UNSPECIFIED.)
CURVE()
GEOMETRIC_REPRESENTATION_ITEM()
RATIONAL_B_SPLINE_CURVE((1.,1.,1.,1.,1.,1.))
REPRESENTATION_ITEM('')
);
#246=(
BOUNDED_CURVE()
B_SPLINE_CURVE(5,(#15146,#15147,#15148,#15149,#15150,#15151),
 .UNSPECIFIED.,.F.,.F.)
B_SPLINE_CURVE_WITH_KNOTS((6,6),(0.984324037881406,1.),.UNSPECIFIED.)
CURVE()
GEOMETRIC_REPRESENTATION_ITEM()
RATIONAL_B_SPLINE_CURVE((1.,1.,1.,1.,1.,1.))
REPRESENTATION_ITEM('')
);
#247=(
BOUNDED_CURVE()
B_SPLINE_CURVE(5,(#15263,#15264,#15265,#15266,#15267,#15268),
 .UNSPECIFIED.,.F.,.F.)
B_SPLINE_CURVE_WITH_KNOTS((6,6),(0.984324037881406,1.),.UNSPECIFIED.)
CURVE()
GEOMETRIC_REPRESENTATION_ITEM()
RATIONAL_B_SPLINE_CURVE((1.,1.,1.,1.,1.,1.))
REPRESENTATION_ITEM('')
);
#248=(
BOUNDED_CURVE()
B_SPLINE_CURVE(5,(#15318,#15319,#15320,#15321,#15322,#15323),
 .UNSPECIFIED.,.F.,.F.)
B_SPLINE_CURVE_WITH_KNOTS((6,6),(0.984324037881405,1.),.UNSPECIFIED.)
CURVE()
GEOMETRIC_REPRESENTATION_ITEM()
RATIONAL_B_SPLINE_CURVE((1.,1.,1.,1.,1.,1.))
REPRESENTATION_ITEM('')
);
#249=(
BOUNDED_CURVE()
B_SPLINE_CURVE(5,(#15373,#15374,#15375,#15376,#15377,#15378),
 .UNSPECIFIED.,.F.,.F.)
B_SPLINE_CURVE_WITH_KNOTS((6,6),(0.984324037881405,1.),.UNSPECIFIED.)
CURVE()
GEOMETRIC_REPRESENTATION_ITEM()
RATIONAL_B_SPLINE_CURVE((1.,1.,1.,1.,1.,1.))
REPRESENTATION_ITEM('')
);
#250=(
BOUNDED_CURVE()
B_SPLINE_CURVE(5,(#15490,#15491,#15492,#15493,#15494,#15495),
 .UNSPECIFIED.,.F.,.F.)
B_SPLINE_CURVE_WITH_KNOTS((6,6),(0.984324037881406,1.),.UNSPECIFIED.)
CURVE()
GEOMETRIC_REPRESENTATION_ITEM()
RATIONAL_B_SPLINE_CURVE((1.,1.,1.,1.,1.,1.))
REPRESENTATION_ITEM('')
);
#251=(
BOUNDED_CURVE()
B_SPLINE_CURVE(5,(#15607,#15608,#15609,#15610,#15611,#15612),
 .UNSPECIFIED.,.F.,.F.)
B_SPLINE_CURVE_WITH_KNOTS((6,6),(0.984324037881406,1.),.UNSPECIFIED.)
CURVE()
GEOMETRIC_REPRESENTATION_ITEM()
RATIONAL_B_SPLINE_CURVE((1.,1.,1.,1.,1.,1.))
REPRESENTATION_ITEM('')
);
#252=(
BOUNDED_CURVE()
B_SPLINE_CURVE(5,(#15724,#15725,#15726,#15727,#15728,#15729),
 .UNSPECIFIED.,.F.,.F.)
B_SPLINE_CURVE_WITH_KNOTS((6,6),(0.984324037881405,1.),.UNSPECIFIED.)
CURVE()
GEOMETRIC_REPRESENTATION_ITEM()
RATIONAL_B_SPLINE_CURVE((1.,1.,1.,1.,1.,1.))
REPRESENTATION_ITEM('')
);
#253=(
BOUNDED_CURVE()
B_SPLINE_CURVE(5,(#15779,#15780,#15781,#15782,#15783,#15784),
 .UNSPECIFIED.,.F.,.F.)
B_SPLINE_CURVE_WITH_KNOTS((6,6),(0.984324037881406,1.),.UNSPECIFIED.)
CURVE()
GEOMETRIC_REPRESENTATION_ITEM()
RATIONAL_B_SPLINE_CURVE((1.,1.,1.,1.,1.,1.))
REPRESENTATION_ITEM('')
);
#254=(
BOUNDED_CURVE()
B_SPLINE_CURVE(5,(#15834,#15835,#15836,#15837,#15838,#15839),
 .UNSPECIFIED.,.F.,.F.)
B_SPLINE_CURVE_WITH_KNOTS((6,6),(0.984324037881405,1.),.UNSPECIFIED.)
CURVE()
GEOMETRIC_REPRESENTATION_ITEM()
RATIONAL_B_SPLINE_CURVE((1.,1.,1.,1.,1.,1.))
REPRESENTATION_ITEM('')
);
#335=B_SPLINE_CURVE_WITH_KNOTS('',3,(#9770,#9771,#9772,#9773,#9774,#9775),
 .UNSPECIFIED.,.F.,.F.,(4,2,4),(0.150716059332096,0.396655662727104,0.79918856408106),
 .UNSPECIFIED.);
#336=B_SPLINE_CURVE_WITH_KNOTS('',3,(#9778,#9779,#9780,#9781),
 .UNSPECIFIED.,.F.,.F.,(4,4),(0.,0.07026331290575),.UNSPECIFIED.);
#337=B_SPLINE_CURVE_WITH_KNOTS('',3,(#9785,#9786,#9787,#9788,#9789,#9790,
#9791,#9792,#9793,#9794),.UNSPECIFIED.,.F.,.F.,(4,2,2,2,4),(0.331186461688063,
0.41497096063171,0.498755459575358,0.580564191475742,0.662372923376126),
 .UNSPECIFIED.);
#338=B_SPLINE_CURVE_WITH_KNOTS('',3,(#9796,#9797,#9798,#9799,#9800,#9801,
#9802,#9803,#9804,#9805,#9806,#9807,#9808,#9809,#9810,#9811,#9812,#9813,
#9814),.UNSPECIFIED.,.F.,.F.,(4,2,2,2,3,2,2,2,4),(0.993559385064188,1.07734388400784,
1.16112838295148,1.24293711485187,1.32474584675225,1.40655457865263,1.48836331055302,
1.57214780949667,1.65593230844031),.UNSPECIFIED.);
#339=B_SPLINE_CURVE_WITH_KNOTS('',3,(#9815,#9816,#9817,#9818,#9819,#9820,
#9821,#9822,#9823,#9824),.UNSPECIFIED.,.F.,.F.,(4,2,2,2,4),(0.662372923376126,
0.744181655276509,0.825990387176893,0.909774886120541,0.993559385064188),
 .UNSPECIFIED.);
#340=B_SPLINE_CURVE_WITH_KNOTS('',3,(#9832,#9833,#9834,#9835,#9836,#9837,
#9838,#9839,#9840,#9841),.UNSPECIFIED.,.F.,.F.,(4,2,2,2,4),(0.934777550778115,
1.01265597092338,1.09053439106865,1.1684522293864,1.24637006770415),
 .UNSPECIFIED.);
#341=B_SPLINE_CURVE_WITH_KNOTS('',3,(#9843,#9844,#9845,#9846,#9847,#9848,
#9849,#9850,#9851,#9852,#9853,#9854,#9855,#9856,#9857,#9858,#9859,#9860),
 .UNSPECIFIED.,.F.,.F.,(4,2,2,2,2,2,2,2,4),(0.311592516926038,0.389470937071308,
0.467349357216578,0.545267195534327,0.623185033852077,0.701102872169826,
0.779020710487576,0.856899130632846,0.934777550778115),.UNSPECIFIED.);
#342=B_SPLINE_CURVE_WITH_KNOTS('',3,(#9861,#9862,#9863,#9864,#9865,#9866,
#9867,#9868,#9869,#9870),.UNSPECIFIED.,.F.,.F.,(4,2,2,2,4),(0.,0.0779178383177495,
0.155835676635499,0.233714096780769,0.311592516926038),.UNSPECIFIED.);
#343=B_SPLINE_CURVE_WITH_KNOTS('',3,(#9874,#9875,#9876,#9877,#9878,#9879,
#9880,#9881,#9882,#9883,#9884,#9885,#9886,#9887,#9888,#9889,#9890,#9891),
 .UNSPECIFIED.,.F.,.F.,(4,2,2,2,2,2,2,2,4),(0.331186461688063,0.41497096063171,
0.498755459575358,0.580564191475742,0.662372923376126,0.744181655276509,
0.825990387176893,0.909774886120541,0.993559385064188),.UNSPECIFIED.);
#344=B_SPLINE_CURVE_WITH_KNOTS('',3,(#9895,#9896,#9897,#9898,#9899,#9900,
#9901,#9902,#9903,#9904,#9905,#9906,#9907,#9908,#9909,#9910,#9911,#9912,
#9913),.UNSPECIFIED.,.F.,.F.,(4,2,2,2,3,2,2,2,4),(0.993559385064188,1.07734388400784,
1.16112838295148,1.24293711485187,1.32474584675225,1.40655457865263,1.48836331055302,
1.57214780949667,1.65593230844031),.UNSPECIFIED.);
#345=B_SPLINE_CURVE_WITH_KNOTS('',3,(#9918,#9919,#9920,#9921,#9922,#9923,
#9924,#9925,#9926,#9927),.UNSPECIFIED.,.F.,.F.,(4,2,2,2,4),(0.,0.0779178383177495,
0.155835676635499,0.233714096780769,0.311592516926038),.UNSPECIFIED.);
#346=B_SPLINE_CURVE_WITH_KNOTS('',3,(#9928,#9929,#9930,#9931,#9932,#9933,
#9934,#9935,#9936,#9937,#9938,#9939,#9940,#9941,#9942,#9943,#9944,#9945,
#9946,#9947,#9948,#9949,#9950,#9951,#9952,#9953),.UNSPECIFIED.,.F.,.F.,
(4,2,2,2,2,2,2,2,2,2,2,2,4),(0.311592516926038,0.389470937071308,0.467349357216578,
0.545267195534327,0.623185033852077,0.701102872169826,0.779020710487576,
0.856899130632846,0.934777550778115,1.01265597092338,1.09053439106865,1.1684522293864,
1.24637006770415),.UNSPECIFIED.);
#347=B_SPLINE_CURVE_WITH_KNOTS('',3,(#11468,#11469,#11470,#11471,#11472,
#11473,#11474,#11475,#11476,#11477,#11478,#11479,#11480,#11481,#11482,#11483),
 .UNSPECIFIED.,.F.,.F.,(4,2,2,2,2,2,2,4),(-0.530628370665211,-0.438179590528544,
-0.368258168563918,-0.304848975856517,-0.18363749529654,-0.110124331620288,
-0.0450078568694679,0.),.UNSPECIFIED.);
#348=B_SPLINE_CURVE_WITH_KNOTS('',3,(#11485,#11486,#11487,#11488,#11489,
#11490,#11491,#11492,#11493,#11494),.UNSPECIFIED.,.F.,.F.,(4,2,2,2,4),(-0.385870474914649,
-0.314059136023987,-0.239369291310806,-0.135126671385033,0.),
 .UNSPECIFIED.);
#349=B_SPLINE_CURVE_WITH_KNOTS('',3,(#11499,#11500,#11501,#11502,#11503,
#11504,#11505,#11506,#11507,#11508,#11509,#11510,#11511,#11512,#11513,#11514),
 .UNSPECIFIED.,.F.,.F.,(4,2,2,2,2,2,2,4),(-0.530628370644343,-0.438179590518134,
-0.368258168560348,-0.304848975855471,-0.183637495295765,-0.110124331619939,
-0.0450078568693863,0.),.UNSPECIFIED.);
#350=B_SPLINE_CURVE_WITH_KNOTS('',3,(#11516,#11517,#11518,#11519,#11520,
#11521,#11522,#11523,#11524,#11525),.UNSPECIFIED.,.F.,.F.,(4,2,2,2,4),(-0.385870474933965,
-0.314059136035213,-0.239369291313655,-0.135126671384286,0.),
 .UNSPECIFIED.);
#351=B_SPLINE_CURVE_WITH_KNOTS('',3,(#11530,#11531,#11532,#11533,#11534,
#11535,#11536,#11537,#11538,#11539,#11540,#11541,#11542,#11543,#11544,#11545),
 .UNSPECIFIED.,.F.,.F.,(4,2,2,2,2,2,2,4),(-0.530628370635536,-0.438179590504702,
-0.368258168546477,-0.304848975844171,-0.183637495294767,-0.110124331621409,
-0.0450078568700918,0.),.UNSPECIFIED.);
#352=B_SPLINE_CURVE_WITH_KNOTS('',3,(#11547,#11548,#11549,#11550,#11551,
#11552,#11553,#11554,#11555,#11556),.UNSPECIFIED.,.F.,.F.,(4,2,2,2,4),(-0.38587047497607,
-0.314059136063502,-0.239369291327215,-0.135126671388375,0.),
 .UNSPECIFIED.);
#353=B_SPLINE_CURVE_WITH_KNOTS('',3,(#11561,#11562,#11563,#11564,#11565,
#11566,#11567,#11568,#11569,#11570,#11571,#11572,#11573,#11574,#11575,#11576),
 .UNSPECIFIED.,.F.,.F.,(4,2,2,2,2,2,2,4),(-0.530628370675815,-0.438179590528513,
-0.368258168562559,-0.304848975858297,-0.18363749529809,-0.110124331620912,
-0.0450078568696886,0.),.UNSPECIFIED.);
#354=B_SPLINE_CURVE_WITH_KNOTS('',3,(#11578,#11579,#11580,#11581,#11582,
#11583,#11584,#11585,#11586,#11587),.UNSPECIFIED.,.F.,.F.,(4,2,2,2,4),(-0.38587047490018,
-0.31405913601548,-0.239369291308653,-0.135126671385624,0.),
 .UNSPECIFIED.);
#355=B_SPLINE_CURVE_WITH_KNOTS('',3,(#11592,#11593,#11594,#11595,#11596,
#11597,#11598,#11599,#11600,#11601,#11602,#11603,#11604,#11605,#11606,#11607),
 .UNSPECIFIED.,.F.,.F.,(4,2,2,2,2,2,2,4),(-0.530628370637572,-0.438179590515746,
-0.36825816856043,-0.304848975855941,-0.183637495296692,-0.11012433162041,
-0.0450078568695264,0.),.UNSPECIFIED.);
#356=B_SPLINE_CURVE_WITH_KNOTS('',3,(#11609,#11610,#11611,#11612,#11613,
#11614,#11615,#11616,#11617,#11618),.UNSPECIFIED.,.F.,.F.,(4,2,2,2,4),(-0.385870474947031,
-0.314059136043926,-0.239369291317936,-0.135126671385535,0.),
 .UNSPECIFIED.);
#357=B_SPLINE_CURVE_WITH_KNOTS('',3,(#11623,#11624,#11625,#11626,#11627,
#11628,#11629,#11630,#11631,#11632,#11633,#11634,#11635,#11636,#11637,#11638),
 .UNSPECIFIED.,.F.,.F.,(4,2,2,2,2,2,2,4),(-0.530628370654682,-0.438179590523996,
-0.368258168563118,-0.304848975857009,-0.18363749529649,-0.11012433162027,
-0.0450078568694597,0.),.UNSPECIFIED.);
#358=B_SPLINE_CURVE_WITH_KNOTS('',3,(#11640,#11641,#11642,#11643,#11644,
#11645,#11646,#11647,#11648,#11649),.UNSPECIFIED.,.F.,.F.,(4,2,2,2,4),(-0.385870474959562,
-0.314059136052487,-0.239369291321785,-0.135126671386547,0.),
 .UNSPECIFIED.);
#359=B_SPLINE_CURVE_WITH_KNOTS('',3,(#11654,#11655,#11656,#11657,#11658,
#11659,#11660,#11661,#11662,#11663,#11664,#11665,#11666,#11667,#11668,#11669),
 .UNSPECIFIED.,.F.,.F.,(4,2,2,2,2,2,2,4),(-0.530628370674281,-0.438179590531451,
-0.368258168567116,-0.304848975861869,-0.183637495299954,-0.110124331621691,
-0.0450078568699812,0.),.UNSPECIFIED.);
#360=B_SPLINE_CURVE_WITH_KNOTS('',3,(#11671,#11672,#11673,#11674,#11675,
#11676,#11677,#11678,#11679,#11680),.UNSPECIFIED.,.F.,.F.,(4,2,2,2,4),(-0.385870474910037,
-0.314059136021404,-0.239369291308962,-0.135126671384126,0.),
 .UNSPECIFIED.);
#361=B_SPLINE_CURVE_WITH_KNOTS('',3,(#11685,#11686,#11687,#11688,#11689,
#11690,#11691,#11692,#11693,#11694,#11695,#11696,#11697,#11698,#11699,#11700),
 .UNSPECIFIED.,.F.,.F.,(4,2,2,2,2,2,2,4),(-0.530628370695727,-0.438179590541344,
-0.368258168569252,-0.304848975860891,-0.183637495301317,-0.110124331622579,
-0.0450078568703517,0.),.UNSPECIFIED.);
#362=B_SPLINE_CURVE_WITH_KNOTS('',3,(#11702,#11703,#11704,#11705,#11706,
#11707,#11708,#11709,#11710,#11711),.UNSPECIFIED.,.F.,.F.,(4,2,2,2,4),(-0.385870474968525,
-0.314059136057782,-0.239369291326298,-0.135126671389261,0.),
 .UNSPECIFIED.);
#363=B_SPLINE_CURVE_WITH_KNOTS('',3,(#11716,#11717,#11718,#11719,#11720,
#11721,#11722,#11723,#11724,#11725,#11726,#11727,#11728,#11729,#11730,#11731),
 .UNSPECIFIED.,.F.,.F.,(4,2,2,2,2,2,2,4),(-0.530628370650825,-0.438179590522418,
-0.368258168560991,-0.304848975853564,-0.183637495295637,-0.110124331620217,
-0.0450078568694996,0.),.UNSPECIFIED.);
#364=B_SPLINE_CURVE_WITH_KNOTS('',3,(#11733,#11734,#11735,#11736,#11737,
#11738,#11739,#11740,#11741,#11742),.UNSPECIFIED.,.F.,.F.,(4,2,2,2,4),(-0.385870474779879,
-0.314059135940437,-0.239369291280562,-0.135126671382187,0.),
 .UNSPECIFIED.);
#365=B_SPLINE_CURVE_WITH_KNOTS('',3,(#11747,#11748,#11749,#11750,#11751,
#11752,#11753,#11754,#11755,#11756,#11757,#11758,#11759,#11760,#11761,#11762),
 .UNSPECIFIED.,.F.,.F.,(4,2,2,2,2,2,2,4),(-0.530628370676019,-0.438179590538652,
-0.36825816857226,-0.30484897586235,-0.1836374952988,-0.110124331620691,
-0.0450078568695567,0.),.UNSPECIFIED.);
#366=B_SPLINE_CURVE_WITH_KNOTS('',3,(#11764,#11765,#11766,#11767,#11768,
#11769,#11770,#11771,#11772,#11773),.UNSPECIFIED.,.F.,.F.,(4,2,2,2,4),(-0.385870474961872,
-0.314059136052803,-0.23936929132047,-0.135126671385201,0.),
 .UNSPECIFIED.);
#367=B_SPLINE_CURVE_WITH_KNOTS('',3,(#11778,#11779,#11780,#11781,#11782,
#11783,#11784,#11785,#11786,#11787,#11788,#11789,#11790,#11791,#11792,#11793),
 .UNSPECIFIED.,.F.,.F.,(4,2,2,2,2,2,2,4),(-0.530628370643928,-0.43817959051309,
-0.368258168552352,-0.30484897584762,-0.183637495292806,-0.110124331619433,
-0.0450078568692464,0.),.UNSPECIFIED.);
#368=B_SPLINE_CURVE_WITH_KNOTS('',3,(#11795,#11796,#11797,#11798,#11799,
#11800,#11801,#11802,#11803,#11804),.UNSPECIFIED.,.F.,.F.,(4,2,2,2,4),(-0.385870474963212,
-0.314059136054532,-0.239369291322363,-0.135126671386519,0.),
 .UNSPECIFIED.);
#369=B_SPLINE_CURVE_WITH_KNOTS('',3,(#11809,#11810,#11811,#11812,#11813,
#11814,#11815,#11816,#11817,#11818,#11819,#11820,#11821,#11822,#11823,#11824),
 .UNSPECIFIED.,.F.,.F.,(4,2,2,2,2,2,2,4),(-0.530628370650933,-0.438179590512731,
-0.368258168547674,-0.304848975842705,-0.18363749528933,-0.110124331617902,
-0.045007856868715,0.),.UNSPECIFIED.);
#370=B_SPLINE_CURVE_WITH_KNOTS('',3,(#11826,#11827,#11828,#11829,#11830,
#11831,#11832,#11833,#11834,#11835),.UNSPECIFIED.,.F.,.F.,(4,2,2,2,4),(-0.385870475012667,
-0.314059136085294,-0.239369291335385,-0.135126671389136,0.),
 .UNSPECIFIED.);
#371=B_SPLINE_CURVE_WITH_KNOTS('',3,(#11840,#11841,#11842,#11843,#11844,
#11845,#11846,#11847,#11848,#11849,#11850,#11851,#11852,#11853,#11854,#11855),
 .UNSPECIFIED.,.F.,.F.,(4,2,2,2,2,2,2,4),(-0.530628370751346,-0.438179590589213,
-0.368258168607749,-0.304848975890323,-0.183637495306509,-0.110124331620972,
-0.0450078568692966,0.),.UNSPECIFIED.);
#372=B_SPLINE_CURVE_WITH_KNOTS('',3,(#11857,#11858,#11859,#11860,#11861,
#11862,#11863,#11864,#11865,#11866),.UNSPECIFIED.,.F.,.F.,(4,2,2,2,4),(-0.38587047498259,
-0.314059136066901,-0.239369291329437,-0.135126671389429,0.),
 .UNSPECIFIED.);
#373=B_SPLINE_CURVE_WITH_KNOTS('',3,(#11871,#11872,#11873,#11874,#11875,
#11876,#11877,#11878,#11879,#11880,#11881,#11882,#11883,#11884,#11885,#11886),
 .UNSPECIFIED.,.F.,.F.,(4,2,2,2,2,2,2,4),(-0.5306283706486,-0.438179590513393,
-0.368258168552838,-0.304848975849369,-0.183637495296429,-0.110124331621205,
-0.0450078568699516,0.),.UNSPECIFIED.);
#374=B_SPLINE_CURVE_WITH_KNOTS('',3,(#11888,#11889,#11890,#11891,#11892,
#11893,#11894,#11895,#11896,#11897),.UNSPECIFIED.,.F.,.F.,(4,2,2,2,4),(-0.385870474786871,
-0.314059135944633,-0.23936929128179,-0.135126671382188,0.),
 .UNSPECIFIED.);
#375=B_SPLINE_CURVE_WITH_KNOTS('',3,(#11902,#11903,#11904,#11905,#11906,
#11907,#11908,#11909,#11910,#11911,#11912,#11913,#11914,#11915,#11916,#11917),
 .UNSPECIFIED.,.F.,.F.,(4,2,2,2,2,2,2,4),(-0.530628370663462,-0.438179590525026,
-0.368258168561372,-0.304848975855513,-0.183637495296643,-0.110124331620531,
-0.0450078568695819,0.),.UNSPECIFIED.);
#376=B_SPLINE_CURVE_WITH_KNOTS('',3,(#11919,#11920,#11921,#11922,#11923,
#11924,#11925,#11926,#11927,#11928),.UNSPECIFIED.,.F.,.F.,(4,2,2,2,4),(-0.385870474865139,
-0.31405913599211,-0.239369291297457,-0.135126671382209,0.),
 .UNSPECIFIED.);
#377=B_SPLINE_CURVE_WITH_KNOTS('',3,(#11933,#11934,#11935,#11936,#11937,
#11938,#11939,#11940,#11941,#11942,#11943,#11944,#11945,#11946,#11947,#11948),
 .UNSPECIFIED.,.F.,.F.,(4,2,2,2,2,2,2,4),(-0.5306283706703,-0.438179590528974,
-0.368258168563241,-0.304848975856583,-0.183637495296807,-0.11012433162058,
-0.0450078568695895,0.),.UNSPECIFIED.);
#378=B_SPLINE_CURVE_WITH_KNOTS('',3,(#11950,#11951,#11952,#11953,#11954,
#11955,#11956,#11957,#11958,#11959),.UNSPECIFIED.,.F.,.F.,(4,2,2,2,4),(-0.385870474981686,
-0.314059136066467,-0.23936929132688,-0.135126671387158,0.),
 .UNSPECIFIED.);
#379=B_SPLINE_CURVE_WITH_KNOTS('',3,(#11964,#11965,#11966,#11967,#11968,
#11969,#11970,#11971,#11972,#11973,#11974,#11975,#11976,#11977,#11978,#11979),
 .UNSPECIFIED.,.F.,.F.,(4,2,2,2,2,2,2,4),(-0.530628370630461,-0.438179590512618,
-0.368258168556241,-0.304848975849823,-0.183637495293183,-0.110124331618942,
-0.045007856869029,0.),.UNSPECIFIED.);
#380=B_SPLINE_CURVE_WITH_KNOTS('',3,(#11981,#11982,#11983,#11984,#11985,
#11986,#11987,#11988,#11989,#11990),.UNSPECIFIED.,.F.,.F.,(4,2,2,2,4),(-0.385870475012076,
-0.314059136083952,-0.239369291332893,-0.135126671387372,0.),
 .UNSPECIFIED.);
#381=B_SPLINE_CURVE_WITH_KNOTS('',3,(#11995,#11996,#11997,#11998,#11999,
#12000,#12001,#12002,#12003,#12004,#12005,#12006,#12007,#12008,#12009,#12010),
 .UNSPECIFIED.,.F.,.F.,(4,2,2,2,2,2,2,4),(-0.530628370690807,-0.438179590550982,
-0.36825816857982,-0.304848975865985,-0.183637495299133,-0.110124331620377,
-0.0450078568693689,0.),.UNSPECIFIED.);
#382=B_SPLINE_CURVE_WITH_KNOTS('',3,(#12012,#12013,#12014,#12015,#12016,
#12017,#12018,#12019,#12020,#12021),.UNSPECIFIED.,.F.,.F.,(4,2,2,2,4),(-0.385870474994837,
-0.314059136073306,-0.239369291329243,-0.135126671387283,0.),
 .UNSPECIFIED.);
#383=B_SPLINE_CURVE_WITH_KNOTS('',3,(#12026,#12027,#12028,#12029,#12030,
#12031,#12032,#12033,#12034,#12035,#12036,#12037,#12038,#12039,#12040,#12041),
 .UNSPECIFIED.,.F.,.F.,(4,2,2,2,2,2,2,4),(-0.530628370667125,-0.438179590523967,
-0.368258168558833,-0.304848975854,-0.183637495296909,-0.110124331621158,
-0.0450078568698694,0.),.UNSPECIFIED.);
#384=B_SPLINE_CURVE_WITH_KNOTS('',3,(#12043,#12044,#12045,#12046,#12047,
#12048,#12049,#12050,#12051,#12052),.UNSPECIFIED.,.F.,.F.,(4,2,2,2,4),(-0.385870474971746,
-0.31405913605961,-0.239369291323841,-0.135126671386237,0.),
 .UNSPECIFIED.);
#385=B_SPLINE_CURVE_WITH_KNOTS('',3,(#12067,#12068,#12069,#12070,#12071,
#12072,#12073,#12074,#12075,#12076,#12077,#12078,#12079,#12080,#12081,#12082),
 .UNSPECIFIED.,.F.,.F.,(4,2,2,2,2,2,2,4),(-0.530628370661766,-0.438179590520695,
-0.368258168559026,-0.304848975856584,-0.18363749529647,-0.110124331620193,
-0.0450078568694207,0.),.UNSPECIFIED.);
#386=B_SPLINE_CURVE_WITH_KNOTS('',3,(#12084,#12085,#12086,#12087,#12088,
#12089,#12090,#12091,#12092,#12093),.UNSPECIFIED.,.F.,.F.,(4,2,2,2,4),(-0.385870474867246,
-0.314059135993994,-0.239369291299197,-0.135126671383269,0.),
 .UNSPECIFIED.);
#387=B_SPLINE_CURVE_WITH_KNOTS('',3,(#12121,#12122,#12123,#12124,#12125,
#12126,#12127,#12128,#12129,#12130,#12131,#12132,#12133,#12134,#12135,#12136,
#12137,#12138,#12139,#12140,#12141,#12142,#12143,#12144,#12145,#12146,#12147,
#12148),.UNSPECIFIED.,.F.,.F.,(4,3,3,3,3,3,3,3,3,4),(0.,0.10535075562,0.211630470100858,
0.32063653562082,0.396655662726854,0.476762504776631,0.559142830371662,
0.643714126095473,0.734783989792354,0.799188564080633),.UNSPECIFIED.);
#388=B_SPLINE_CURVE_WITH_KNOTS('',3,(#12181,#12182,#12183,#12184,#12185,
#12186,#12187,#12188,#12189,#12190,#12191,#12192,#12193,#12194,#12195,#12196,
#12197,#12198,#12199,#12200,#12201,#12202,#12203,#12204,#12205,#12206,#12207,
#12208),.UNSPECIFIED.,.F.,.F.,(4,3,3,3,3,3,3,3,3,4),(0.,0.105350580727645,
0.211630157393727,0.320636018170041,0.39665566272708,0.476762496060542,
0.559143022698535,0.643714701417285,0.734784330146394,0.79918856408108),
 .UNSPECIFIED.);
#389=B_SPLINE_CURVE_WITH_KNOTS('',3,(#12241,#12242,#12243,#12244,#12245,
#12246,#12247,#12248,#12249,#12250,#12251,#12252,#12253,#12254,#12255,#12256,
#12257,#12258,#12259,#12260,#12261,#12262,#12263,#12264,#12265,#12266,#12267,
#12268),.UNSPECIFIED.,.F.,.F.,(4,3,3,3,3,3,3,3,3,4),(0.,0.105350505304636,
0.211630022763806,0.320635795967351,0.396655662726985,0.476762492451757,
0.559143105761226,0.643714949539588,0.734784479477035,0.799188564080899),
 .UNSPECIFIED.);
#390=B_SPLINE_CURVE_WITH_KNOTS('',3,(#12301,#12302,#12303,#12304,#12305,
#12306,#12307,#12308,#12309,#12310,#12311,#12312,#12313,#12314,#12315,#12316,
#12317,#12318,#12319,#12320,#12321,#12322,#12323,#12324,#12325,#12326,#12327,
#12328),.UNSPECIFIED.,.F.,.F.,(4,3,3,3,3,3,3,3,3,4),(0.,0.105350517029453,
0.21163004368367,0.320635830472424,0.39665566272694,0.476762493006737,0.559143092844083,
0.64371491096779,0.734784456165118,0.799188564080757),.UNSPECIFIED.);
#391=B_SPLINE_CURVE_WITH_KNOTS('',3,(#12361,#12362,#12363,#12364,#12365,
#12366,#12367,#12368,#12369,#12370,#12371,#12372,#12373,#12374,#12375,#12376,
#12377,#12378,#12379,#12380,#12381,#12382,#12383,#12384,#12385,#12386,#12387,
#12388),.UNSPECIFIED.,.F.,.F.,(4,3,3,3,3,3,3,3,3,4),(0.,0.105350617782938,
0.211630223586182,0.320636127543284,0.396655662726963,0.476762497865765,
0.559142981916141,0.643714579518275,0.734784257333252,0.79918856408084),
 .UNSPECIFIED.);
#392=B_SPLINE_CURVE_WITH_KNOTS('',3,(#12421,#12422,#12423,#12424,#12425,
#12426,#12427,#12428,#12429,#12430,#12431,#12432,#12433,#12434,#12435,#12436,
#12437,#12438,#12439,#12440,#12441,#12442,#12443,#12444,#12445,#12446,#12447,
#12448),.UNSPECIFIED.,.F.,.F.,(4,3,3,3,3,3,3,3,3,4),(0.,0.105350755620646,
0.211630470101819,0.320636535621585,0.396655662726938,0.476762504777025,
0.55914283037207,0.643714126095984,0.734783989792887,0.799188564080764),
 .UNSPECIFIED.);
#393=B_SPLINE_CURVE_WITH_KNOTS('',3,(#12481,#12482,#12483,#12484,#12485,
#12486,#12487,#12488,#12489,#12490,#12491,#12492,#12493,#12494,#12495,#12496,
#12497,#12498,#12499,#12500,#12501,#12502,#12503,#12504,#12505,#12506,#12507,
#12508),.UNSPECIFIED.,.F.,.F.,(4,3,3,3,3,3,3,3,3,4),(0.,0.105350580727718,
0.211630157393232,0.320636018169153,0.396655662726952,0.476762496060361,
0.559143022698262,0.643714701416882,0.734784330145906,0.799188564080778),
 .UNSPECIFIED.);
#394=B_SPLINE_CURVE_WITH_KNOTS('',3,(#12541,#12542,#12543,#12544,#12545,
#12546,#12547,#12548,#12549,#12550,#12551,#12552,#12553,#12554,#12555,#12556,
#12557,#12558,#12559,#12560,#12561,#12562,#12563,#12564,#12565,#12566,#12567,
#12568),.UNSPECIFIED.,.F.,.F.,(4,3,3,3,3,3,3,3,3,4),(0.,0.105350505304776,
0.211630022764475,0.320635795967906,0.396655662726964,0.476762492451559,
0.559143105761002,0.643714949539319,0.7347844794766,0.799188564080815),
 .UNSPECIFIED.);
#395=B_SPLINE_CURVE_WITH_KNOTS('',3,(#12601,#12602,#12603,#12604,#12605,
#12606,#12607,#12608,#12609,#12610,#12611,#12612,#12613,#12614,#12615,#12616,
#12617,#12618,#12619,#12620,#12621,#12622,#12623,#12624,#12625,#12626,#12627,
#12628),.UNSPECIFIED.,.F.,.F.,(4,3,3,3,3,3,3,3,3,4),(0.,0.105350517029029,
0.211630043683767,0.320635830472862,0.396655662727039,0.476762493006702,
0.559143092844054,0.643714910967833,0.734784456165161,0.799188564080931),
 .UNSPECIFIED.);
#396=B_SPLINE_CURVE_WITH_KNOTS('',3,(#12661,#12662,#12663,#12664,#12665,
#12666,#12667,#12668,#12669,#12670,#12671,#12672,#12673,#12674,#12675,#12676,
#12677,#12678,#12679,#12680,#12681,#12682,#12683,#12684,#12685,#12686,#12687,
#12688),.UNSPECIFIED.,.F.,.F.,(4,3,3,3,3,3,3,3,3,4),(0.,0.105350617782518,
0.211630223586211,0.320636127542873,0.396655662726838,0.476762497865674,
0.559142981916043,0.643714579518135,0.734784257333135,0.799188564080614),
 .UNSPECIFIED.);
#397=B_SPLINE_CURVE_WITH_KNOTS('',3,(#12721,#12722,#12723,#12724),
 .UNSPECIFIED.,.F.,.F.,(4,4),(0.,0.150716059332096),.UNSPECIFIED.);
#398=B_SPLINE_CURVE_WITH_KNOTS('',3,(#12757,#12758,#12759,#12760,#12761,
#12762,#12763,#12764,#12765,#12766,#12767,#12768,#12769,#12770,#12771,#12772,
#12773,#12774,#12775,#12776,#12777,#12778,#12779,#12780,#12781,#12782,#12783,
#12784),.UNSPECIFIED.,.F.,.F.,(4,3,3,3,3,3,3,3,3,4),(0.,0.1053505807278,
0.211630157393979,0.320636018170015,0.396655662727064,0.47676249606025,
0.559143022698166,0.643714701416806,0.734784330145882,0.799188564081011),
 .UNSPECIFIED.);
#399=B_SPLINE_CURVE_WITH_KNOTS('',3,(#12817,#12818,#12819,#12820,#12821,
#12822,#12823,#12824,#12825,#12826,#12827,#12828,#12829,#12830,#12831,#12832,
#12833,#12834,#12835,#12836,#12837,#12838,#12839,#12840,#12841,#12842,#12843,
#12844),.UNSPECIFIED.,.F.,.F.,(4,3,3,3,3,3,3,3,3,4),(0.,0.105350505304457,
0.21163002276398,0.320635795967329,0.396655662726986,0.476762492451752,
0.55914310576122,0.643714949539569,0.734784479476893,0.799188564080866),
 .UNSPECIFIED.);
#400=B_SPLINE_CURVE_WITH_KNOTS('',3,(#12877,#12878,#12879,#12880,#12881,
#12882,#12883,#12884,#12885,#12886,#12887,#12888,#12889,#12890,#12891,#12892,
#12893,#12894,#12895,#12896,#12897,#12898,#12899,#12900,#12901,#12902,#12903,
#12904),.UNSPECIFIED.,.F.,.F.,(4,3,3,3,3,3,3,3,3,4),(0.,0.105350517029183,
0.211630043683744,0.320635830472283,0.396655662726922,0.476762493006743,
0.559143092844057,0.6437149109678,0.734784456165119,0.799188564080692),
 .UNSPECIFIED.);
#401=B_SPLINE_CURVE_WITH_KNOTS('',3,(#12937,#12938,#12939,#12940,#12941,
#12942,#12943,#12944,#12945,#12946,#12947,#12948,#12949,#12950,#12951,#12952,
#12953,#12954,#12955,#12956,#12957,#12958,#12959,#12960,#12961,#12962,#12963,
#12964),.UNSPECIFIED.,.F.,.F.,(4,3,3,3,3,3,3,3,3,4),(0.,0.105350617782988,
0.211630223585978,0.320636127542671,0.396655662727022,0.476762497865844,
0.559142981916226,0.643714579518403,0.734784257333494,0.799188564080915),
 .UNSPECIFIED.);
#402=B_SPLINE_CURVE_WITH_KNOTS('',3,(#12997,#12998,#12999,#13000,#13001,
#13002,#13003,#13004,#13005,#13006,#13007,#13008,#13009,#13010,#13011,#13012,
#13013,#13014,#13015,#13016,#13017,#13018,#13019,#13020,#13021,#13022,#13023,
#13024),.UNSPECIFIED.,.F.,.F.,(4,3,3,3,3,3,3,3,3,4),(0.,0.105350755620161,
0.211630470100934,0.320636535620834,0.396655662727017,0.476762504776933,
0.559142830371988,0.643714126095916,0.734783989792824,0.799188564080951),
 .UNSPECIFIED.);
#403=B_SPLINE_CURVE_WITH_KNOTS('',3,(#13057,#13058,#13059,#13060,#13061,
#13062,#13063,#13064,#13065,#13066,#13067,#13068,#13069,#13070,#13071,#13072,
#13073,#13074,#13075,#13076,#13077,#13078,#13079,#13080,#13081,#13082,#13083,
#13084),.UNSPECIFIED.,.F.,.F.,(4,3,3,3,3,3,3,3,3,4),(0.,0.105350580727699,
0.211630157394061,0.320636018170424,0.396655662727046,0.476762496060293,
0.559143022698226,0.643714701416837,0.7347843301459,0.799188564080982),
 .UNSPECIFIED.);
#404=B_SPLINE_CURVE_WITH_KNOTS('',3,(#13117,#13118,#13119,#13120,#13121,
#13122,#13123,#13124,#13125,#13126,#13127,#13128,#13129,#13130,#13131,#13132,
#13133,#13134,#13135,#13136,#13137,#13138,#13139,#13140,#13141,#13142,#13143,
#13144),.UNSPECIFIED.,.F.,.F.,(4,3,3,3,3,3,3,3,3,4),(0.,0.105350505304653,
0.211630022764195,0.320635795967923,0.396655662727108,0.476762492451716,
0.559143105761212,0.643714949539593,0.734784479477028,0.79918856408114),
 .UNSPECIFIED.);
#405=B_SPLINE_CURVE_WITH_KNOTS('',3,(#13177,#13178,#13179,#13180,#13181,
#13182,#13183,#13184,#13185,#13186,#13187,#13188,#13189,#13190,#13191,#13192,
#13193,#13194,#13195,#13196,#13197,#13198,#13199,#13200,#13201,#13202,#13203,
#13204),.UNSPECIFIED.,.F.,.F.,(4,3,3,3,3,3,3,3,3,4),(0.,0.105350517029269,
0.211630043683721,0.320635830472785,0.396655662726906,0.476762493006721,
0.559143092844096,0.643714910967841,0.734784456165104,0.799188564080754),
 .UNSPECIFIED.);
#406=B_SPLINE_CURVE_WITH_KNOTS('',3,(#13237,#13238,#13239,#13240,#13241,
#13242,#13243,#13244,#13245,#13246,#13247,#13248,#13249,#13250,#13251,#13252,
#13253,#13254,#13255,#13256,#13257,#13258,#13259,#13260,#13261,#13262,#13263,
#13264),.UNSPECIFIED.,.F.,.F.,(4,3,3,3,3,3,3,3,3,4),(0.,0.105350617782791,
0.211630223586115,0.320636127543467,0.396655662727067,0.476762497865883,
0.559142981916264,0.643714579518415,0.734784257333419,0.799188564081055),
 .UNSPECIFIED.);
#407=B_SPLINE_CURVE_WITH_KNOTS('',3,(#13388,#13389,#13390,#13391,#13392,
#13393,#13394,#13395,#13396,#13397,#13398,#13399,#13400,#13401,#13402,#13403,
#13404,#13405,#13406,#13407,#13408,#13409,#13410,#13411,#13412,#13413,#13414,
#13415,#13416,#13417,#13418,#13419,#13420,#13421,#13422,#13423,#13424,#13425,
#13426,#13427),.UNSPECIFIED.,.F.,.F.,(4,3,3,3,3,3,3,3,3,3,3,3,3,4),(0.,
0.080816837337899,0.159744691662406,0.238272865643827,0.316637951909253,
0.39214567920225,0.451150927438286,0.506701203283771,0.5619638530984,0.663361603296831,
0.672200447289742,0.727455868377893,0.755180292788767,0.782993887761336),
 .UNSPECIFIED.);
#408=B_SPLINE_CURVE_WITH_KNOTS('',3,(#13435,#13436,#13437,#13438,#13439,
#13440),.UNSPECIFIED.,.F.,.F.,(4,2,4),(0.07026331290575,0.392145679202251,
0.782993887761363),.UNSPECIFIED.);
#409=B_SPLINE_CURVE_WITH_KNOTS('',3,(#13443,#13444,#13445,#13446,#13447,
#13448,#13449,#13450,#13451,#13452,#13453,#13454,#13455,#13456,#13457,#13458,
#13459,#13460,#13461,#13462,#13463,#13464,#13465,#13466,#13467,#13468,#13469,
#13470),.UNSPECIFIED.,.F.,.F.,(4,3,3,3,3,3,3,3,3,4),(0.,0.0804727531474491,
0.159375053173973,0.237925353906231,0.316349809181948,0.39214567920222,
0.495918215505369,0.598324344999396,0.699619020094378,0.782993887761245),
 .UNSPECIFIED.);
#410=B_SPLINE_CURVE_WITH_KNOTS('',3,(#13473,#13474,#13475,#13476,#13477,
#13478,#13479,#13480,#13481,#13482,#13483,#13484,#13485,#13486,#13487,#13488,
#13489,#13490,#13491,#13492,#13493,#13494,#13495,#13496,#13497,#13498,#13499,
#13500,#13501,#13502,#13503,#13504,#13505,#13506,#13507,#13508,#13509,#13510,
#13511,#13512),.UNSPECIFIED.,.F.,.F.,(4,3,3,3,3,3,3,3,3,3,3,3,3,4),(0.,
0.0808237501538664,0.159752125840751,0.238279961562834,0.31664406989611,
0.392145679202288,0.45115092743835,0.50670120328386,0.561963853098512,0.663377487277087,
0.672200447289889,0.727455868378047,0.755180292788921,0.782993887761487),
 .UNSPECIFIED.);
#411=B_SPLINE_CURVE_WITH_KNOTS('',3,(#13515,#13516,#13517,#13518,#13519,
#13520,#13521,#13522,#13523,#13524,#13525,#13526,#13527,#13528,#13529,#13530,
#13531,#13532,#13533,#13534,#13535,#13536,#13537,#13538,#13539,#13540,#13541,
#13542,#13543,#13544,#13545,#13546,#13547,#13548,#13549,#13550,#13551,#13552,
#13553,#13554),.UNSPECIFIED.,.F.,.F.,(4,3,3,3,3,3,3,3,3,3,3,3,3,4),(0.,
0.080826365016996,0.15975466022045,0.238282174042087,0.316645830807802,
0.392145679202281,0.451150927438327,0.506701203283823,0.561963853098462,
0.663386079795717,0.672200447289833,0.727455868378004,0.75518029278889,
0.782993887761473),.UNSPECIFIED.);
#412=B_SPLINE_CURVE_WITH_KNOTS('',3,(#13557,#13558,#13559,#13560,#13561,
#13562,#13563,#13564,#13565,#13566,#13567,#13568,#13569,#13570,#13571,#13572,
#13573,#13574,#13575,#13576,#13577,#13578,#13579,#13580,#13581,#13582,#13583,
#13584,#13585,#13586,#13587,#13588,#13589,#13590,#13591,#13592,#13593,#13594,
#13595,#13596),.UNSPECIFIED.,.F.,.F.,(4,3,3,3,3,3,3,3,3,3,3,3,3,4),(0.,
0.0808168373377941,0.15974469166233,0.238272865643754,0.316637951909167,
0.392145679202253,0.451150927438289,0.506701203283775,0.561963853098404,
0.663361603296804,0.672200447289745,0.727455868377895,0.755180292788769,
0.782993887761338),.UNSPECIFIED.);
#413=B_SPLINE_CURVE_WITH_KNOTS('',3,(#13599,#13600,#13601,#13602,#13603,
#13604,#13605,#13606,#13607,#13608,#13609,#13610,#13611,#13612,#13613,#13614,
#13615,#13616,#13617,#13618,#13619,#13620,#13621,#13622,#13623,#13624,#13625,
#13626),.UNSPECIFIED.,.F.,.F.,(4,3,3,3,3,3,3,3,3,4),(0.,0.0804773681583594,
0.159381289585917,0.237932353538847,0.316356775343447,0.392145679202256,
0.495917404016704,0.598322903162837,0.699618128903555,0.782993887761399),
 .UNSPECIFIED.);
#414=B_SPLINE_CURVE_WITH_KNOTS('',3,(#13629,#13630,#13631,#13632,#13633,
#13634,#13635,#13636,#13637,#13638,#13639,#13640,#13641,#13642,#13643,#13644,
#13645,#13646,#13647,#13648,#13649,#13650,#13651,#13652,#13653,#13654,#13655,
#13656),.UNSPECIFIED.,.F.,.F.,(4,3,3,3,3,3,3,3,3,4),(0.,0.0804727531474338,
0.159375053174015,0.237925353906301,0.316349809182045,0.392145679202232,
0.495918215505487,0.598324344999523,0.699619020094104,0.78299388776127),
 .UNSPECIFIED.);
#415=B_SPLINE_CURVE_WITH_KNOTS('',3,(#13659,#13660,#13661,#13662,#13663,
#13664,#13665,#13666,#13667,#13668,#13669,#13670,#13671,#13672,#13673,#13674,
#13675,#13676,#13677,#13678,#13679,#13680,#13681,#13682,#13683,#13684,#13685,
#13686,#13687,#13688,#13689,#13690,#13691,#13692,#13693,#13694,#13695,#13696,
#13697,#13698),.UNSPECIFIED.,.F.,.F.,(4,3,3,3,3,3,3,3,3,3,3,3,3,4),(0.,
0.0808237501539957,0.159752125840905,0.23827996156287,0.316644069896139,
0.392145679202281,0.451150927438335,0.506701203283837,0.561963853098483,
0.663377487276743,0.672200447289856,0.727455868378023,0.755180292788905,
0.782993887761481),.UNSPECIFIED.);
#416=B_SPLINE_CURVE_WITH_KNOTS('',3,(#13701,#13702,#13703,#13704,#13705,
#13706,#13707,#13708,#13709,#13710,#13711,#13712,#13713,#13714,#13715,#13716,
#13717,#13718,#13719,#13720,#13721,#13722,#13723,#13724,#13725,#13726,#13727,
#13728,#13729,#13730,#13731,#13732,#13733,#13734,#13735,#13736,#13737,#13738,
#13739,#13740),.UNSPECIFIED.,.F.,.F.,(4,3,3,3,3,3,3,3,3,3,3,3,3,4),(0.,
0.0808263650166872,0.159754660220132,0.238282174041845,0.316645830807606,
0.392145679202287,0.451150927438335,0.506701203283831,0.561963853098472,
0.663386079795103,0.672200447289846,0.72745586837802,0.755180292788908,
0.782993887761494),.UNSPECIFIED.);
#417=B_SPLINE_CURVE_WITH_KNOTS('',3,(#13743,#13744,#13745,#13746,#13747,
#13748,#13749,#13750,#13751,#13752,#13753,#13754,#13755,#13756,#13757,#13758,
#13759,#13760,#13761,#13762,#13763,#13764,#13765,#13766,#13767,#13768,#13769,
#13770),.UNSPECIFIED.,.F.,.F.,(4,3,3,3,3,3,3,3,3,4),(0.,0.0804773681583258,
0.15938128958588,0.237932353538843,0.316356775343476,0.392145679202253,
0.495917404016412,0.5983229031625,0.699618128903188,0.782993887761353),
 .UNSPECIFIED.);
#418=B_SPLINE_CURVE_WITH_KNOTS('',3,(#13773,#13774,#13775,#13776,#13777,
#13778,#13779,#13780,#13781,#13782,#13783,#13784,#13785,#13786,#13787,#13788,
#13789,#13790,#13791,#13792,#13793,#13794,#13795,#13796,#13797,#13798,#13799,
#13800),.UNSPECIFIED.,.F.,.F.,(4,3,3,3,3,3,3,3,3,4),(0.,0.08047275314732,
0.15937505317391,0.237925353906137,0.316349809181831,0.392145679202234,
0.495918215505687,0.598324344999879,0.699619020095004,0.782993887761323),
 .UNSPECIFIED.);
#419=B_SPLINE_CURVE_WITH_KNOTS('',3,(#13803,#13804,#13805,#13806,#13807,
#13808,#13809,#13810,#13811,#13812,#13813,#13814,#13815,#13816,#13817,#13818,
#13819,#13820,#13821,#13822,#13823,#13824,#13825,#13826,#13827,#13828,#13829,
#13830,#13831,#13832,#13833,#13834,#13835,#13836,#13837,#13838,#13839,#13840,
#13841,#13842),.UNSPECIFIED.,.F.,.F.,(4,3,3,3,3,3,3,3,3,3,3,3,3,4),(0.,
0.0808237501538626,0.159752125840739,0.238279961562764,0.316644069896114,
0.392145679202252,0.451150927438296,0.50670120328379,0.561963853098427,
0.663377487277723,0.672200447289778,0.727455868377928,0.7551802927888,0.782993887761365),
 .UNSPECIFIED.);
#420=B_SPLINE_CURVE_WITH_KNOTS('',3,(#13845,#13846,#13847,#13848,#13849,
#13850,#13851,#13852,#13853,#13854,#13855,#13856,#13857,#13858,#13859,#13860,
#13861,#13862,#13863,#13864,#13865,#13866,#13867,#13868,#13869,#13870,#13871,
#13872,#13873,#13874,#13875,#13876,#13877,#13878,#13879,#13880,#13881,#13882,
#13883,#13884),.UNSPECIFIED.,.F.,.F.,(4,3,3,3,3,3,3,3,3,3,3,3,3,4),(0.,
0.0808263650167775,0.159754660220236,0.238282174041904,0.316645830807637,
0.39214567920233,0.451150927438407,0.506701203283934,0.561963853098602,
0.663386079793417,0.672200447290009,0.72745586837818,0.755180292789061,
0.782993887761632),.UNSPECIFIED.);
#421=B_SPLINE_CURVE_WITH_KNOTS('',3,(#13887,#13888,#13889,#13890,#13891,
#13892,#13893,#13894,#13895,#13896,#13897,#13898,#13899,#13900,#13901,#13902,
#13903,#13904,#13905,#13906,#13907,#13908,#13909,#13910,#13911,#13912,#13913,
#13914,#13915,#13916,#13917,#13918,#13919,#13920,#13921,#13922,#13923,#13924,
#13925,#13926),.UNSPECIFIED.,.F.,.F.,(4,3,3,3,3,3,3,3,3,3,3,3,3,4),(0.,
0.0808168373377771,0.159744691662314,0.238272865643762,0.316637951909151,
0.392145679202262,0.451150927438304,0.506701203283795,0.561963853098429,
0.66336160329673,0.672200447289777,0.727455868377926,0.755180292788798,
0.782993887761364),.UNSPECIFIED.);
#422=B_SPLINE_CURVE_WITH_KNOTS('',3,(#13929,#13930,#13931,#13932,#13933,
#13934,#13935,#13936,#13937,#13938,#13939,#13940,#13941,#13942,#13943,#13944,
#13945,#13946,#13947,#13948,#13949,#13950,#13951,#13952,#13953,#13954,#13955,
#13956),.UNSPECIFIED.,.F.,.F.,(4,3,3,3,3,3,3,3,3,4),(0.,0.0804773681583631,
0.15938128958592,0.237932353538891,0.316356775343511,0.392145679202255,
0.495917404016605,0.598322903162788,0.699618128903027,0.782993887761362),
 .UNSPECIFIED.);
#423=B_SPLINE_CURVE_WITH_KNOTS('',3,(#13959,#13960,#13961,#13962,#13963,
#13964,#13965,#13966,#13967,#13968,#13969,#13970,#13971,#13972,#13973,#13974,
#13975,#13976,#13977,#13978,#13979,#13980,#13981,#13982,#13983,#13984,#13985,
#13986),.UNSPECIFIED.,.F.,.F.,(4,3,3,3,3,3,3,3,3,4),(0.,0.0804727531475009,
0.159375053174066,0.237925353906258,0.316349809181868,0.392145679202247,
0.495918215505489,0.598324344999634,0.699619020094664,0.782993887761332),
 .UNSPECIFIED.);
#424=B_SPLINE_CURVE_WITH_KNOTS('',3,(#13989,#13990,#13991,#13992,#13993,
#13994,#13995,#13996,#13997,#13998,#13999,#14000,#14001,#14002,#14003,#14004,
#14005,#14006,#14007,#14008,#14009,#14010,#14011,#14012,#14013,#14014,#14015,
#14016,#14017,#14018,#14019,#14020,#14021,#14022,#14023,#14024,#14025,#14026,
#14027,#14028),.UNSPECIFIED.,.F.,.F.,(4,3,3,3,3,3,3,3,3,3,3,3,3,4),(0.,
0.0808237501538716,0.159752125840756,0.238279961562882,0.316644069896221,
0.392145679202287,0.451150927438346,0.506701203283854,0.561963853098504,
0.663377487277437,0.672200447289882,0.727455868378044,0.755180292788922,
0.782993887761492),.UNSPECIFIED.);
#425=B_SPLINE_CURVE_WITH_KNOTS('',3,(#14031,#14032,#14033,#14034,#14035,
#14036,#14037,#14038,#14039,#14040,#14041,#14042,#14043,#14044,#14045,#14046,
#14047,#14048,#14049,#14050,#14051,#14052,#14053,#14054,#14055,#14056,#14057,
#14058,#14059,#14060,#14061,#14062,#14063,#14064,#14065,#14066,#14067,#14068,
#14069,#14070),.UNSPECIFIED.,.F.,.F.,(4,3,3,3,3,3,3,3,3,3,3,3,3,4),(0.,
0.0808263650167331,0.159754660220215,0.238282174041877,0.316645830807603,
0.39214567920227,0.451150927438306,0.506701203283791,0.561963853098421,
0.663386079794874,0.672200447289781,0.727455868377954,0.755180292788844,
0.782993887761433),.UNSPECIFIED.);
#426=B_SPLINE_CURVE_WITH_KNOTS('',3,(#14073,#14074,#14075,#14076,#14077,
#14078,#14079,#14080,#14081,#14082,#14083,#14084,#14085,#14086,#14087,#14088,
#14089,#14090,#14091,#14092,#14093,#14094,#14095,#14096,#14097,#14098,#14099,
#14100,#14101,#14102,#14103,#14104,#14105,#14106,#14107,#14108,#14109,#14110,
#14111,#14112),.UNSPECIFIED.,.F.,.F.,(4,3,3,3,3,3,3,3,3,3,3,3,3,4),(0.,
0.0808168373379184,0.159744691662454,0.238272865643917,0.316637951909378,
0.39214567920226,0.451150927438305,0.506701203283801,0.561963853098441,
0.663361603296352,0.672200447289796,0.727455868377948,0.755180292788821,
0.782993887761387),.UNSPECIFIED.);
#628=SHAPE_REPRESENTATION_RELATIONSHIP('SRR','None',#23301,#638);
#638=ADVANCED_BREP_SHAPE_REPRESENTATION('',(#658),#23245);
#648=STYLED_ITEM('',(#23448),#658);
#658=MANIFOLD_SOLID_BREP('Body1',#7026);
#680=CONICAL_SURFACE('',#7280,12.1473403730037,0.739193465255218);
#681=CONICAL_SURFACE('',#7282,2.175,0.785398163397448);
#682=CONICAL_SURFACE('',#7285,2.175,0.785398163397448);
#683=CONICAL_SURFACE('',#7288,6.275,0.785398163397448);
#684=CONICAL_SURFACE('',#7315,6.275,0.785398163397451);
#685=CONICAL_SURFACE('',#7319,9.75,0.785398163397451);
#686=CONICAL_SURFACE('',#7324,14.5,0.817645045832702);
#687=CONICAL_SURFACE('',#7326,14.5,0.817645045832702);
#688=CONICAL_SURFACE('',#7328,14.5,0.817645045832702);
#689=CONICAL_SURFACE('',#7330,14.5,0.817645045832702);
#690=CONICAL_SURFACE('',#7332,14.5,0.817645045832702);
#691=CONICAL_SURFACE('',#7334,14.5,0.817645045832702);
#692=CONICAL_SURFACE('',#7336,14.5,0.817645045832702);
#693=CONICAL_SURFACE('',#7338,14.5,0.817645045832702);
#694=CONICAL_SURFACE('',#7340,14.5,0.817645045832702);
#695=CONICAL_SURFACE('',#7342,14.5,0.817645045832702);
#696=CONICAL_SURFACE('',#7344,14.5,0.817645045832702);
#697=CONICAL_SURFACE('',#7346,14.5,0.817645045832702);
#698=CONICAL_SURFACE('',#7348,14.5,0.817645045832702);
#699=CONICAL_SURFACE('',#7350,14.5,0.817645045832702);
#700=CONICAL_SURFACE('',#7352,14.5,0.817645045832702);
#701=CONICAL_SURFACE('',#7354,14.5,0.817645045832702);
#702=CONICAL_SURFACE('',#7356,14.5,0.817645045832702);
#703=CONICAL_SURFACE('',#7358,14.5,0.817645045832702);
#704=CONICAL_SURFACE('',#7360,14.5,0.817645045832702);
#705=CONICAL_SURFACE('',#7362,14.5,0.817645045832702);
#706=CONICAL_SURFACE('',#7367,14.5,0.817645045832702);
#707=CONICAL_SURFACE('',#7371,12.1473403730037,0.739193465255218);
#798=FACE_BOUND('',#1469,.T.);
#799=FACE_BOUND('',#1471,.T.);
#800=FACE_BOUND('',#1474,.T.);
#801=FACE_BOUND('',#1477,.T.);
#802=FACE_BOUND('',#1562,.T.);
#886=PLANE('',#7295);
#887=PLANE('',#7317);
#888=PLANE('',#7369);
#889=PLANE('',#7392);
#890=PLANE('',#7393);
#891=PLANE('',#7394);
#892=PLANE('',#7395);
#893=PLANE('',#7396);
#894=PLANE('',#7397);
#895=PLANE('',#7398);
#896=PLANE('',#7399);
#897=PLANE('',#7400);
#898=PLANE('',#7401);
#899=PLANE('',#7402);
#900=PLANE('',#7403);
#901=PLANE('',#7404);
#902=PLANE('',#7405);
#903=PLANE('',#7406);
#904=PLANE('',#7407);
#905=PLANE('',#7408);
#906=PLANE('',#7409);
#907=PLANE('',#7410);
#908=PLANE('',#7411);
#1049=FACE_OUTER_BOUND('',#1462,.T.);
#1050=FACE_OUTER_BOUND('',#1463,.T.);
#1051=FACE_OUTER_BOUND('',#1464,.T.);
#1052=FACE_OUTER_BOUND('',#1465,.T.);
#1053=FACE_OUTER_BOUND('',#1466,.T.);
#1054=FACE_OUTER_BOUND('',#1467,.T.);
#1055=FACE_OUTER_BOUND('',#1468,.T.);
#1056=FACE_OUTER_BOUND('',#1470,.T.);
#1057=FACE_OUTER_BOUND('',#1472,.T.);
#1058=FACE_OUTER_BOUND('',#1473,.T.);
#1059=FACE_OUTER_BOUND('',#1475,.T.);
#1060=FACE_OUTER_BOUND('',#1476,.T.);
#1061=FACE_OUTER_BOUND('',#1478,.T.);
#1062=FACE_OUTER_BOUND('',#1479,.T.);
#1063=FACE_OUTER_BOUND('',#1480,.T.);
#1064=FACE_OUTER_BOUND('',#1481,.T.);
#1065=FACE_OUTER_BOUND('',#1482,.T.);
#1066=FACE_OUTER_BOUND('',#1483,.T.);
#1067=FACE_OUTER_BOUND('',#1484,.T.);
#1068=FACE_OUTER_BOUND('',#1485,.T.);
#1069=FACE_OUTER_BOUND('',#1486,.T.);
#1070=FACE_OUTER_BOUND('',#1487,.T.);
#1071=FACE_OUTER_BOUND('',#1488,.T.);
#1072=FACE_OUTER_BOUND('',#1489,.T.);
#1073=FACE_OUTER_BOUND('',#1490,.T.);
#1074=FACE_OUTER_BOUND('',#1491,.T.);
#1075=FACE_OUTER_BOUND('',#1492,.T.);
#1076=FACE_OUTER_BOUND('',#1493,.T.);
#1077=FACE_OUTER_BOUND('',#1494,.T.);
#1078=FACE_OUTER_BOUND('',#1495,.T.);
#1079=FACE_OUTER_BOUND('',#1496,.T.);
#1080=FACE_OUTER_BOUND('',#1497,.T.);
#1081=FACE_OUTER_BOUND('',#1498,.T.);
#1082=FACE_OUTER_BOUND('',#1499,.T.);
#1083=FACE_OUTER_BOUND('',#1500,.T.);
#1084=FACE_OUTER_BOUND('',#1501,.T.);
#1085=FACE_OUTER_BOUND('',#1502,.T.);
#1086=FACE_OUTER_BOUND('',#1503,.T.);
#1087=FACE_OUTER_BOUND('',#1504,.T.);
#1088=FACE_OUTER_BOUND('',#1505,.T.);
#1089=FACE_OUTER_BOUND('',#1506,.T.);
#1090=FACE_OUTER_BOUND('',#1507,.T.);
#1091=FACE_OUTER_BOUND('',#1508,.T.);
#1092=FACE_OUTER_BOUND('',#1509,.T.);
#1093=FACE_OUTER_BOUND('',#1510,.T.);
#1094=FACE_OUTER_BOUND('',#1511,.T.);
#1095=FACE_OUTER_BOUND('',#1512,.T.);
#1096=FACE_OUTER_BOUND('',#1513,.T.);
#1097=FACE_OUTER_BOUND('',#1514,.T.);
#1098=FACE_OUTER_BOUND('',#1515,.T.);
#1099=FACE_OUTER_BOUND('',#1516,.T.);
#1100=FACE_OUTER_BOUND('',#1517,.T.);
#1101=FACE_OUTER_BOUND('',#1518,.T.);
#1102=FACE_OUTER_BOUND('',#1519,.T.);
#1103=FACE_OUTER_BOUND('',#1520,.T.);
#1104=FACE_OUTER_BOUND('',#1521,.T.);
#1105=FACE_OUTER_BOUND('',#1522,.T.);
#1106=FACE_OUTER_BOUND('',#1523,.T.);
#1107=FACE_OUTER_BOUND('',#1524,.T.);
#1108=FACE_OUTER_BOUND('',#1525,.T.);
#1109=FACE_OUTER_BOUND('',#1526,.T.);
#1110=FACE_OUTER_BOUND('',#1527,.T.);
#1111=FACE_OUTER_BOUND('',#1528,.T.);
#1112=FACE_OUTER_BOUND('',#1529,.T.);
#1113=FACE_OUTER_BOUND('',#1530,.T.);
#1114=FACE_OUTER_BOUND('',#1531,.T.);
#1115=FACE_OUTER_BOUND('',#1532,.T.);
#1116=FACE_OUTER_BOUND('',#1533,.T.);
#1117=FACE_OUTER_BOUND('',#1534,.T.);
#1118=FACE_OUTER_BOUND('',#1535,.T.);
#1119=FACE_OUTER_BOUND('',#1536,.T.);
#1120=FACE_OUTER_BOUND('',#1537,.T.);
#1121=FACE_OUTER_BOUND('',#1538,.T.);
#1122=FACE_OUTER_BOUND('',#1539,.T.);
#1123=FACE_OUTER_BOUND('',#1540,.T.);
#1124=FACE_OUTER_BOUND('',#1541,.T.);
#1125=FACE_OUTER_BOUND('',#1542,.T.);
#1126=FACE_OUTER_BOUND('',#1543,.T.);
#1127=FACE_OUTER_BOUND('',#1544,.T.);
#1128=FACE_OUTER_BOUND('',#1545,.T.);
#1129=FACE_OUTER_BOUND('',#1546,.T.);
#1130=FACE_OUTER_BOUND('',#1547,.T.);
#1131=FACE_OUTER_BOUND('',#1548,.T.);
#1132=FACE_OUTER_BOUND('',#1549,.T.);
#1133=FACE_OUTER_BOUND('',#1550,.T.);
#1134=FACE_OUTER_BOUND('',#1551,.T.);
#1135=FACE_OUTER_BOUND('',#1552,.T.);
#1136=FACE_OUTER_BOUND('',#1553,.T.);
#1137=FACE_OUTER_BOUND('',#1554,.T.);
#1138=FACE_OUTER_BOUND('',#1555,.T.);
#1139=FACE_OUTER_BOUND('',#1556,.T.);
#1140=FACE_OUTER_BOUND('',#1557,.T.);
#1141=FACE_OUTER_BOUND('',#1558,.T.);
#1142=FACE_OUTER_BOUND('',#1559,.T.);
#1143=FACE_OUTER_BOUND('',#1560,.T.);
#1144=FACE_OUTER_BOUND('',#1561,.T.);
#1462=EDGE_LOOP('',(#4747,#4748,#4749,#4750));
#1463=EDGE_LOOP('',(#4751,#4752,#4753,#4754,#4755,#4756));
#1464=EDGE_LOOP('',(#4757,#4758,#4759,#4760,#4761,#4762));
#1465=EDGE_LOOP('',(#4763,#4764,#4765,#4766,#4767));
#1466=EDGE_LOOP('',(#4768,#4769,#4770,#4771,#4772));
#1467=EDGE_LOOP('',(#4773,#4774,#4775,#4776,#4777));
#1468=EDGE_LOOP('',(#4778,#4779,#4780,#4781,#4782,#4783,#4784,#4785,#4786,
#4787,#4788));
#1469=EDGE_LOOP('',(#4789,#4790));
#1470=EDGE_LOOP('',(#4791,#4792,#4793,#4794,#4795,#4796,#4797,#4798,#4799,
#4800,#4801,#4802,#4803,#4804,#4805,#4806,#4807,#4808,#4809,#4810,#4811,
#4812,#4813,#4814,#4815,#4816,#4817,#4818,#4819,#4820,#4821,#4822,#4823,
#4824,#4825,#4826,#4827,#4828,#4829,#4830,#4831,#4832,#4833,#4834,#4835,
#4836,#4837,#4838,#4839,#4840,#4841,#4842,#4843,#4844,#4845,#4846,#4847,
#4848,#4849,#4850));
#1471=EDGE_LOOP('',(#4851));
#1472=EDGE_LOOP('',(#4852,#4853,#4854,#4855,#4856));
#1473=EDGE_LOOP('',(#4857));
#1474=EDGE_LOOP('',(#4858));
#1475=EDGE_LOOP('',(#4859,#4860,#4861,#4862,#4863));
#1476=EDGE_LOOP('',(#4864,#4865,#4866,#4867,#4868,#4869,#4870,#4871,#4872,
#4873));
#1477=EDGE_LOOP('',(#4874,#4875));
#1478=EDGE_LOOP('',(#4876,#4877,#4878));
#1479=EDGE_LOOP('',(#4879,#4880,#4881));
#1480=EDGE_LOOP('',(#4882,#4883,#4884));
#1481=EDGE_LOOP('',(#4885,#4886,#4887));
#1482=EDGE_LOOP('',(#4888,#4889,#4890));
#1483=EDGE_LOOP('',(#4891,#4892,#4893));
#1484=EDGE_LOOP('',(#4894,#4895,#4896));
#1485=EDGE_LOOP('',(#4897,#4898,#4899));
#1486=EDGE_LOOP('',(#4900,#4901,#4902));
#1487=EDGE_LOOP('',(#4903,#4904,#4905));
#1488=EDGE_LOOP('',(#4906,#4907,#4908));
#1489=EDGE_LOOP('',(#4909,#4910,#4911));
#1490=EDGE_LOOP('',(#4912,#4913,#4914));
#1491=EDGE_LOOP('',(#4915,#4916,#4917));
#1492=EDGE_LOOP('',(#4918,#4919,#4920));
#1493=EDGE_LOOP('',(#4921,#4922,#4923));
#1494=EDGE_LOOP('',(#4924,#4925,#4926));
#1495=EDGE_LOOP('',(#4927,#4928,#4929));
#1496=EDGE_LOOP('',(#4930,#4931,#4932));
#1497=EDGE_LOOP('',(#4933,#4934,#4935,#4936));
#1498=EDGE_LOOP('',(#4937,#4938,#4939,#4940));
#1499=EDGE_LOOP('',(#4941,#4942,#4943));
#1500=EDGE_LOOP('',(#4944,#4945,#4946,#4947,#4948));
#1501=EDGE_LOOP('',(#4949,#4950,#4951,#4952,#4953));
#1502=EDGE_LOOP('',(#4954,#4955,#4956,#4957,#4958));
#1503=EDGE_LOOP('',(#4959,#4960,#4961,#4962,#4963));
#1504=EDGE_LOOP('',(#4964,#4965,#4966,#4967,#4968));
#1505=EDGE_LOOP('',(#4969,#4970,#4971,#4972,#4973));
#1506=EDGE_LOOP('',(#4974,#4975,#4976,#4977,#4978));
#1507=EDGE_LOOP('',(#4979,#4980,#4981,#4982,#4983));
#1508=EDGE_LOOP('',(#4984,#4985,#4986,#4987,#4988));
#1509=EDGE_LOOP('',(#4989,#4990,#4991,#4992,#4993));
#1510=EDGE_LOOP('',(#4994,#4995,#4996,#4997,#4998,#4999));
#1511=EDGE_LOOP('',(#5000,#5001,#5002,#5003,#5004));
#1512=EDGE_LOOP('',(#5005,#5006,#5007,#5008,#5009));
#1513=EDGE_LOOP('',(#5010,#5011,#5012,#5013,#5014));
#1514=EDGE_LOOP('',(#5015,#5016,#5017,#5018,#5019));
#1515=EDGE_LOOP('',(#5020,#5021,#5022,#5023,#5024));
#1516=EDGE_LOOP('',(#5025,#5026,#5027,#5028,#5029));
#1517=EDGE_LOOP('',(#5030,#5031,#5032,#5033,#5034));
#1518=EDGE_LOOP('',(#5035,#5036,#5037,#5038,#5039));
#1519=EDGE_LOOP('',(#5040,#5041,#5042,#5043,#5044));
#1520=EDGE_LOOP('',(#5045,#5046,#5047,#5048,#5049));
#1521=EDGE_LOOP('',(#5050,#5051,#5052,#5053));
#1522=EDGE_LOOP('',(#5054,#5055,#5056,#5057,#5058,#5059,#5060,#5061,#5062,
#5063,#5064,#5065,#5066,#5067,#5068,#5069,#5070,#5071,#5072,#5073,#5074,
#5075,#5076,#5077,#5078,#5079,#5080,#5081,#5082,#5083,#5084,#5085,#5086,
#5087,#5088,#5089,#5090,#5091,#5092,#5093,#5094,#5095,#5096,#5097,#5098,
#5099,#5100,#5101,#5102,#5103,#5104,#5105,#5106,#5107,#5108,#5109,#5110,
#5111,#5112,#5113,#5114,#5115,#5116,#5117,#5118,#5119,#5120,#5121,#5122,
#5123,#5124,#5125,#5126,#5127,#5128,#5129,#5130,#5131,#5132,#5133,#5134,
#5135,#5136,#5137));
#1523=EDGE_LOOP('',(#5138,#5139,#5140,#5141,#5142));
#1524=EDGE_LOOP('',(#5143,#5144,#5145,#5146));
#1525=EDGE_LOOP('',(#5147,#5148,#5149,#5150,#5151));
#1526=EDGE_LOOP('',(#5152,#5153,#5154,#5155));
#1527=EDGE_LOOP('',(#5156,#5157,#5158,#5159,#5160));
#1528=EDGE_LOOP('',(#5161,#5162,#5163,#5164));
#1529=EDGE_LOOP('',(#5165,#5166,#5167,#5168,#5169));
#1530=EDGE_LOOP('',(#5170,#5171,#5172,#5173));
#1531=EDGE_LOOP('',(#5174,#5175,#5176,#5177,#5178));
#1532=EDGE_LOOP('',(#5179,#5180,#5181,#5182));
#1533=EDGE_LOOP('',(#5183,#5184,#5185,#5186,#5187));
#1534=EDGE_LOOP('',(#5188,#5189,#5190,#5191));
#1535=EDGE_LOOP('',(#5192,#5193,#5194,#5195,#5196));
#1536=EDGE_LOOP('',(#5197,#5198,#5199,#5200));
#1537=EDGE_LOOP('',(#5201,#5202,#5203,#5204,#5205));
#1538=EDGE_LOOP('',(#5206,#5207,#5208,#5209));
#1539=EDGE_LOOP('',(#5210,#5211,#5212,#5213,#5214,#5215));
#1540=EDGE_LOOP('',(#5216,#5217,#5218,#5219));
#1541=EDGE_LOOP('',(#5220,#5221,#5222,#5223,#5224));
#1542=EDGE_LOOP('',(#5225,#5226,#5227,#5228,#5229));
#1543=EDGE_LOOP('',(#5230,#5231,#5232,#5233,#5234));
#1544=EDGE_LOOP('',(#5235,#5236,#5237,#5238));
#1545=EDGE_LOOP('',(#5239,#5240,#5241,#5242,#5243));
#1546=EDGE_LOOP('',(#5244,#5245,#5246,#5247));
#1547=EDGE_LOOP('',(#5248,#5249,#5250,#5251,#5252));
#1548=EDGE_LOOP('',(#5253,#5254,#5255,#5256));
#1549=EDGE_LOOP('',(#5257,#5258,#5259,#5260,#5261));
#1550=EDGE_LOOP('',(#5262,#5263,#5264,#5265));
#1551=EDGE_LOOP('',(#5266,#5267,#5268,#5269,#5270));
#1552=EDGE_LOOP('',(#5271,#5272,#5273,#5274));
#1553=EDGE_LOOP('',(#5275,#5276,#5277,#5278,#5279));
#1554=EDGE_LOOP('',(#5280,#5281,#5282,#5283));
#1555=EDGE_LOOP('',(#5284,#5285,#5286,#5287,#5288));
#1556=EDGE_LOOP('',(#5289,#5290,#5291,#5292));
#1557=EDGE_LOOP('',(#5293,#5294,#5295,#5296,#5297));
#1558=EDGE_LOOP('',(#5298,#5299,#5300,#5301));
#1559=EDGE_LOOP('',(#5302,#5303,#5304,#5305,#5306));
#1560=EDGE_LOOP('',(#5307,#5308,#5309,#5310));
#1561=EDGE_LOOP('',(#5311));
#1562=EDGE_LOOP('',(#5312));
#1924=LINE('',#9768,#2183);
#1925=LINE('',#9826,#2184);
#1926=LINE('',#9830,#2185);
#1927=LINE('',#9893,#2186);
#1928=LINE('',#9916,#2187);
#1929=LINE('',#9958,#2188);
#1930=LINE('',#9967,#2189);
#1931=LINE('',#9968,#2190);
#1932=LINE('',#11449,#2191);
#1933=LINE('',#11456,#2192);
#1934=LINE('',#11461,#2193);
#1935=LINE('',#11463,#2194);
#1936=LINE('',#12058,#2195);
#1937=LINE('',#12062,#2196);
#1938=LINE('',#12119,#2197);
#1939=LINE('',#12179,#2198);
#1940=LINE('',#12239,#2199);
#1941=LINE('',#12299,#2200);
#1942=LINE('',#12359,#2201);
#1943=LINE('',#12419,#2202);
#1944=LINE('',#12479,#2203);
#1945=LINE('',#12539,#2204);
#1946=LINE('',#12599,#2205);
#1947=LINE('',#12659,#2206);
#1948=LINE('',#12719,#2207);
#1949=LINE('',#12755,#2208);
#1950=LINE('',#12815,#2209);
#1951=LINE('',#12875,#2210);
#1952=LINE('',#12935,#2211);
#1953=LINE('',#12995,#2212);
#1954=LINE('',#13055,#2213);
#1955=LINE('',#13115,#2214);
#1956=LINE('',#13175,#2215);
#1957=LINE('',#13235,#2216);
#1958=LINE('',#13432,#2217);
#2183=VECTOR('',#8184,12.1473403730037);
#2184=VECTOR('',#8189,2.175);
#2185=VECTOR('',#8194,2.05);
#2186=VECTOR('',#8197,2.175);
#2187=VECTOR('',#8202,2.05);
#2188=VECTOR('',#8207,6.275);
#2189=VECTOR('',#8218,6.025);
#2190=VECTOR('',#8219,6.025);
#2191=VECTOR('',#8262,6.275);
#2192=VECTOR('',#8271,9.75);
#2193=VECTOR('',#8278,10.);
#2194=VECTOR('',#8279,10.);
#2195=VECTOR('',#8362,14.5);
#2196=VECTOR('',#8367,10.5);
#2197=VECTOR('',#8374,8.74592262443523);
#2198=VECTOR('',#8375,8.74592262443523);
#2199=VECTOR('',#8376,8.74592262443523);
#2200=VECTOR('',#8377,8.74592262443523);
#2201=VECTOR('',#8378,8.74592262443523);
#2202=VECTOR('',#8379,8.74592262443523);
#2203=VECTOR('',#8380,8.74592262443523);
#2204=VECTOR('',#8381,8.74592262443523);
#2205=VECTOR('',#8382,8.74592262443523);
#2206=VECTOR('',#8383,8.74592262443523);
#2207=VECTOR('',#8384,8.74592262443523);
#2208=VECTOR('',#8385,8.74592262443523);
#2209=VECTOR('',#8386,8.74592262443523);
#2210=VECTOR('',#8387,8.74592262443523);
#2211=VECTOR('',#8388,8.74592262443523);
#2212=VECTOR('',#8389,8.74592262443523);
#2213=VECTOR('',#8390,8.74592262443523);
#2214=VECTOR('',#8391,8.74592262443523);
#2215=VECTOR('',#8392,8.74592262443523);
#2216=VECTOR('',#8393,8.74592262443523);
#2217=VECTOR('',#8400,12.1473403730037);
#2420=CIRCLE('',#7281,9.16192731696939);
#2421=CIRCLE('',#7283,2.05);
#2422=CIRCLE('',#7286,2.05);
#2423=CIRCLE('',#7289,6.525);
#2424=CIRCLE('',#7290,6.025);
#2425=CIRCLE('',#7291,6.025);
#2426=CIRCLE('',#7293,6.025);
#2427=CIRCLE('',#7294,6.025);
#2428=CIRCLE('',#7296,9.16192731696939);
#2429=CIRCLE('',#7297,9.16192731696939);
#2430=CIRCLE('',#7298,9.16192731696939);
#2431=CIRCLE('',#7299,9.16192731696939);
#2432=CIRCLE('',#7300,9.16192731696939);
#2433=CIRCLE('',#7301,9.16192731696939);
#2434=CIRCLE('',#7302,9.16192731696939);
#2435=CIRCLE('',#7303,9.16192731696939);
#2436=CIRCLE('',#7304,9.16192731696939);
#2437=CIRCLE('',#7305,9.16192731696939);
#2438=CIRCLE('',#7306,9.16192731696939);
#2439=CIRCLE('',#7307,9.16192731696939);
#2440=CIRCLE('',#7308,9.16192731696939);
#2441=CIRCLE('',#7309,9.16192731696939);
#2442=CIRCLE('',#7310,9.16192731696939);
#2443=CIRCLE('',#7311,9.16192731696939);
#2444=CIRCLE('',#7312,9.16192731696939);
#2445=CIRCLE('',#7313,9.16192731696939);
#2446=CIRCLE('',#7314,9.16192731696939);
#2447=CIRCLE('',#7316,6.525);
#2448=CIRCLE('',#7318,9.5);
#2449=CIRCLE('',#7320,10.);
#2450=CIRCLE('',#7321,10.);
#2451=CIRCLE('',#7323,10.);
#2452=CIRCLE('',#7325,14.4466666666667);
#2453=CIRCLE('',#7327,14.4466666666667);
#2454=CIRCLE('',#7329,14.4466666666667);
#2455=CIRCLE('',#7331,14.4466666666667);
#2456=CIRCLE('',#7333,14.4466666666667);
#2457=CIRCLE('',#7335,14.4466666666667);
#2458=CIRCLE('',#7337,14.4466666666667);
#2459=CIRCLE('',#7339,14.4466666666667);
#2460=CIRCLE('',#7341,14.4466666666667);
#2461=CIRCLE('',#7343,14.4466666666667);
#2462=CIRCLE('',#7345,14.4466666666667);
#2463=CIRCLE('',#7347,14.4466666666667);
#2464=CIRCLE('',#7349,14.4466666666667);
#2465=CIRCLE('',#7351,14.4466666666667);
#2466=CIRCLE('',#7353,14.4466666666667);
#2467=CIRCLE('',#7355,14.4466666666667);
#2468=CIRCLE('',#7357,14.4466666666667);
#2469=CIRCLE('',#7359,14.4466666666667);
#2470=CIRCLE('',#7361,14.4466666666667);
#2471=CIRCLE('',#7363,14.4233723052509);
#2472=CIRCLE('',#7364,10.5);
#2473=CIRCLE('',#7366,10.5);
#2474=CIRCLE('',#7368,14.4466666666667);
#2475=CIRCLE('',#7370,14.4034641071566);
#2476=CIRCLE('',#7372,14.4034641071566);
#2477=CIRCLE('',#7373,14.4034641071566);
#2478=CIRCLE('',#7374,14.4034641071566);
#2479=CIRCLE('',#7375,14.4034641071566);
#2480=CIRCLE('',#7376,14.4034641071566);
#2481=CIRCLE('',#7377,14.4034641071566);
#2482=CIRCLE('',#7378,14.4034641071566);
#2483=CIRCLE('',#7379,14.4034641071566);
#2484=CIRCLE('',#7380,14.4034641071566);
#2485=CIRCLE('',#7381,14.4034641071566);
#2486=CIRCLE('',#7382,14.4034641071566);
#2487=CIRCLE('',#7383,14.4034641071566);
#2488=CIRCLE('',#7384,14.4034641071566);
#2489=CIRCLE('',#7385,14.4034641071566);
#2490=CIRCLE('',#7386,14.4034641071566);
#2491=CIRCLE('',#7387,14.4034641071566);
#2492=CIRCLE('',#7388,14.4034641071566);
#2493=CIRCLE('',#7389,14.4034641071566);
#2494=CIRCLE('',#7390,14.4034641071566);
#2495=CIRCLE('',#7391,14.4034641071566);
#2790=VERTEX_POINT('',#9766);
#2791=VERTEX_POINT('',#9767);
#2792=VERTEX_POINT('',#9769);
#2793=VERTEX_POINT('',#9776);
#2794=VERTEX_POINT('',#9783);
#2795=VERTEX_POINT('',#9784);
#2796=VERTEX_POINT('',#9795);
#2797=VERTEX_POINT('',#9825);
#2798=VERTEX_POINT('',#9829);
#2799=VERTEX_POINT('',#9831);
#2800=VERTEX_POINT('',#9842);
#2801=VERTEX_POINT('',#9872);
#2802=VERTEX_POINT('',#9873);
#2803=VERTEX_POINT('',#9892);
#2804=VERTEX_POINT('',#9915);
#2805=VERTEX_POINT('',#9917);
#2806=VERTEX_POINT('',#9955);
#2807=VERTEX_POINT('',#9957);
#2808=VERTEX_POINT('',#9959);
#2809=VERTEX_POINT('',#9963);
#2810=VERTEX_POINT('',#9964);
#2811=VERTEX_POINT('',#9970);
#2812=VERTEX_POINT('',#9971);
#2813=VERTEX_POINT('',#9973);
#2814=VERTEX_POINT('',#10009);
#2815=VERTEX_POINT('',#10045);
#2816=VERTEX_POINT('',#10047);
#2817=VERTEX_POINT('',#10083);
#2818=VERTEX_POINT('',#10119);
#2819=VERTEX_POINT('',#10121);
#2820=VERTEX_POINT('',#10157);
#2821=VERTEX_POINT('',#10193);
#2822=VERTEX_POINT('',#10195);
#2823=VERTEX_POINT('',#10231);
#2824=VERTEX_POINT('',#10267);
#2825=VERTEX_POINT('',#10269);
#2826=VERTEX_POINT('',#10305);
#2827=VERTEX_POINT('',#10341);
#2828=VERTEX_POINT('',#10343);
#2829=VERTEX_POINT('',#10379);
#2830=VERTEX_POINT('',#10415);
#2831=VERTEX_POINT('',#10417);
#2832=VERTEX_POINT('',#10453);
#2833=VERTEX_POINT('',#10489);
#2834=VERTEX_POINT('',#10491);
#2835=VERTEX_POINT('',#10527);
#2836=VERTEX_POINT('',#10563);
#2837=VERTEX_POINT('',#10565);
#2838=VERTEX_POINT('',#10636);
#2839=VERTEX_POINT('',#10672);
#2840=VERTEX_POINT('',#10708);
#2841=VERTEX_POINT('',#10710);
#2842=VERTEX_POINT('',#10746);
#2843=VERTEX_POINT('',#10782);
#2844=VERTEX_POINT('',#10784);
#2845=VERTEX_POINT('',#10820);
#2846=VERTEX_POINT('',#10856);
#2847=VERTEX_POINT('',#10858);
#2848=VERTEX_POINT('',#10894);
#2849=VERTEX_POINT('',#10930);
#2850=VERTEX_POINT('',#10932);
#2851=VERTEX_POINT('',#10968);
#2852=VERTEX_POINT('',#11004);
#2853=VERTEX_POINT('',#11006);
#2854=VERTEX_POINT('',#11042);
#2855=VERTEX_POINT('',#11078);
#2856=VERTEX_POINT('',#11080);
#2857=VERTEX_POINT('',#11116);
#2858=VERTEX_POINT('',#11152);
#2859=VERTEX_POINT('',#11154);
#2860=VERTEX_POINT('',#11190);
#2861=VERTEX_POINT('',#11226);
#2862=VERTEX_POINT('',#11228);
#2863=VERTEX_POINT('',#11264);
#2864=VERTEX_POINT('',#11300);
#2865=VERTEX_POINT('',#11302);
#2866=VERTEX_POINT('',#11338);
#2867=VERTEX_POINT('',#11374);
#2868=VERTEX_POINT('',#11376);
#2869=VERTEX_POINT('',#11448);
#2870=VERTEX_POINT('',#11452);
#2871=VERTEX_POINT('',#11455);
#2872=VERTEX_POINT('',#11457);
#2873=VERTEX_POINT('',#11462);
#2874=VERTEX_POINT('',#11466);
#2875=VERTEX_POINT('',#11467);
#2876=VERTEX_POINT('',#11484);
#2877=VERTEX_POINT('',#11497);
#2878=VERTEX_POINT('',#11498);
#2879=VERTEX_POINT('',#11515);
#2880=VERTEX_POINT('',#11528);
#2881=VERTEX_POINT('',#11529);
#2882=VERTEX_POINT('',#11546);
#2883=VERTEX_POINT('',#11559);
#2884=VERTEX_POINT('',#11560);
#2885=VERTEX_POINT('',#11577);
#2886=VERTEX_POINT('',#11590);
#2887=VERTEX_POINT('',#11591);
#2888=VERTEX_POINT('',#11608);
#2889=VERTEX_POINT('',#11621);
#2890=VERTEX_POINT('',#11622);
#2891=VERTEX_POINT('',#11639);
#2892=VERTEX_POINT('',#11652);
#2893=VERTEX_POINT('',#11653);
#2894=VERTEX_POINT('',#11670);
#2895=VERTEX_POINT('',#11683);
#2896=VERTEX_POINT('',#11684);
#2897=VERTEX_POINT('',#11701);
#2898=VERTEX_POINT('',#11714);
#2899=VERTEX_POINT('',#11715);
#2900=VERTEX_POINT('',#11732);
#2901=VERTEX_POINT('',#11745);
#2902=VERTEX_POINT('',#11746);
#2903=VERTEX_POINT('',#11763);
#2904=VERTEX_POINT('',#11776);
#2905=VERTEX_POINT('',#11777);
#2906=VERTEX_POINT('',#11794);
#2907=VERTEX_POINT('',#11807);
#2908=VERTEX_POINT('',#11808);
#2909=VERTEX_POINT('',#11825);
#2910=VERTEX_POINT('',#11838);
#2911=VERTEX_POINT('',#11839);
#2912=VERTEX_POINT('',#11856);
#2913=VERTEX_POINT('',#11869);
#2914=VERTEX_POINT('',#11870);
#2915=VERTEX_POINT('',#11887);
#2916=VERTEX_POINT('',#11900);
#2917=VERTEX_POINT('',#11901);
#2918=VERTEX_POINT('',#11918);
#2919=VERTEX_POINT('',#11931);
#2920=VERTEX_POINT('',#11932);
#2921=VERTEX_POINT('',#11949);
#2922=VERTEX_POINT('',#11962);
#2923=VERTEX_POINT('',#11963);
#2924=VERTEX_POINT('',#11980);
#2925=VERTEX_POINT('',#11993);
#2926=VERTEX_POINT('',#11994);
#2927=VERTEX_POINT('',#12011);
#2928=VERTEX_POINT('',#12024);
#2929=VERTEX_POINT('',#12025);
#2930=VERTEX_POINT('',#12042);
#2931=VERTEX_POINT('',#12055);
#2932=VERTEX_POINT('',#12057);
#2933=VERTEX_POINT('',#12061);
#2934=VERTEX_POINT('',#12065);
#2935=VERTEX_POINT('',#12066);
#2936=VERTEX_POINT('',#12083);
#2937=VERTEX_POINT('',#12120);
#2938=VERTEX_POINT('',#12180);
#2939=VERTEX_POINT('',#12240);
#2940=VERTEX_POINT('',#12300);
#2941=VERTEX_POINT('',#12360);
#2942=VERTEX_POINT('',#12420);
#2943=VERTEX_POINT('',#12480);
#2944=VERTEX_POINT('',#12540);
#2945=VERTEX_POINT('',#12600);
#2946=VERTEX_POINT('',#12660);
#2947=VERTEX_POINT('',#12720);
#2948=VERTEX_POINT('',#12756);
#2949=VERTEX_POINT('',#12816);
#2950=VERTEX_POINT('',#12876);
#2951=VERTEX_POINT('',#12936);
#2952=VERTEX_POINT('',#12996);
#2953=VERTEX_POINT('',#13056);
#2954=VERTEX_POINT('',#13116);
#2955=VERTEX_POINT('',#13176);
#2956=VERTEX_POINT('',#13236);
#2957=VERTEX_POINT('',#13381);
#2958=VERTEX_POINT('',#13431);
#2959=VERTEX_POINT('',#13434);
#2960=VERTEX_POINT('',#13442);
#2961=VERTEX_POINT('',#13472);
#2962=VERTEX_POINT('',#13514);
#2963=VERTEX_POINT('',#13556);
#2964=VERTEX_POINT('',#13598);
#2965=VERTEX_POINT('',#13628);
#2966=VERTEX_POINT('',#13658);
#2967=VERTEX_POINT('',#13700);
#2968=VERTEX_POINT('',#13742);
#2969=VERTEX_POINT('',#13772);
#2970=VERTEX_POINT('',#13802);
#2971=VERTEX_POINT('',#13844);
#2972=VERTEX_POINT('',#13886);
#2973=VERTEX_POINT('',#13928);
#2974=VERTEX_POINT('',#13958);
#2975=VERTEX_POINT('',#13988);
#2976=VERTEX_POINT('',#14030);
#2977=VERTEX_POINT('',#14072);
#3549=EDGE_CURVE('',#2790,#2791,#1924,.T.);
#3550=EDGE_CURVE('',#2790,#2792,#335,.T.);
#3551=EDGE_CURVE('',#2792,#2793,#2420,.T.);
#3552=EDGE_CURVE('',#2793,#2791,#336,.T.);
#3553=EDGE_CURVE('',#2794,#2795,#337,.T.);
#3554=EDGE_CURVE('',#2796,#2794,#338,.T.);
#3555=EDGE_CURVE('',#2795,#2796,#339,.T.);
#3556=EDGE_CURVE('',#2795,#2797,#1925,.T.);
#3557=EDGE_CURVE('',#2797,#2797,#2421,.T.);
#3558=EDGE_CURVE('',#2797,#2798,#1926,.T.);
#3559=EDGE_CURVE('',#2799,#2798,#340,.T.);
#3560=EDGE_CURVE('',#2800,#2799,#341,.T.);
#3561=EDGE_CURVE('',#2798,#2800,#342,.T.);
#3562=EDGE_CURVE('',#2801,#2802,#343,.T.);
#3563=EDGE_CURVE('',#2801,#2803,#1927,.T.);
#3564=EDGE_CURVE('',#2803,#2803,#2422,.T.);
#3565=EDGE_CURVE('',#2802,#2801,#344,.T.);
#3566=EDGE_CURVE('',#2803,#2804,#1928,.T.);
#3567=EDGE_CURVE('',#2805,#2804,#345,.T.);
#3568=EDGE_CURVE('',#2804,#2805,#346,.T.);
#3569=EDGE_CURVE('',#2806,#2806,#2423,.T.);
#3570=EDGE_CURVE('',#2806,#2807,#1929,.T.);
#3571=EDGE_CURVE('',#2807,#2808,#2424,.T.);
#3572=EDGE_CURVE('',#2808,#2807,#2425,.T.);
#3573=EDGE_CURVE('',#2809,#2810,#2426,.T.);
#3574=EDGE_CURVE('',#2810,#2809,#2427,.T.);
#3575=EDGE_CURVE('',#2810,#2799,#1930,.T.);
#3576=EDGE_CURVE('',#2800,#2808,#1931,.T.);
#3577=EDGE_CURVE('',#2811,#2812,#2428,.T.);
#3578=EDGE_CURVE('',#2811,#2813,#175,.T.);
#3579=EDGE_CURVE('',#2813,#2814,#176,.T.);
#3580=EDGE_CURVE('',#2815,#2814,#2429,.T.);
#3581=EDGE_CURVE('',#2815,#2816,#177,.T.);
#3582=EDGE_CURVE('',#2816,#2817,#178,.T.);
#3583=EDGE_CURVE('',#2818,#2817,#2430,.T.);
#3584=EDGE_CURVE('',#2818,#2819,#179,.T.);
#3585=EDGE_CURVE('',#2819,#2820,#180,.T.);
#3586=EDGE_CURVE('',#2821,#2820,#2431,.T.);
#3587=EDGE_CURVE('',#2821,#2822,#181,.T.);
#3588=EDGE_CURVE('',#2822,#2823,#182,.T.);
#3589=EDGE_CURVE('',#2824,#2823,#2432,.T.);
#3590=EDGE_CURVE('',#2824,#2825,#183,.T.);
#3591=EDGE_CURVE('',#2825,#2826,#184,.T.);
#3592=EDGE_CURVE('',#2827,#2826,#2433,.T.);
#3593=EDGE_CURVE('',#2827,#2828,#185,.T.);
#3594=EDGE_CURVE('',#2828,#2829,#186,.T.);
#3595=EDGE_CURVE('',#2830,#2829,#2434,.T.);
#3596=EDGE_CURVE('',#2830,#2831,#187,.T.);
#3597=EDGE_CURVE('',#2831,#2832,#188,.T.);
#3598=EDGE_CURVE('',#2833,#2832,#2435,.T.);
#3599=EDGE_CURVE('',#2833,#2834,#189,.T.);
#3600=EDGE_CURVE('',#2834,#2835,#190,.T.);
#3601=EDGE_CURVE('',#2836,#2835,#2436,.T.);
#3602=EDGE_CURVE('',#2836,#2837,#191,.T.);
#3603=EDGE_CURVE('',#2837,#2793,#192,.T.);
#3604=EDGE_CURVE('',#2792,#2838,#193,.T.);
#3605=EDGE_CURVE('',#2838,#2839,#194,.T.);
#3606=EDGE_CURVE('',#2840,#2839,#2437,.T.);
#3607=EDGE_CURVE('',#2840,#2841,#195,.T.);
#3608=EDGE_CURVE('',#2841,#2842,#196,.T.);
#3609=EDGE_CURVE('',#2843,#2842,#2438,.T.);
#3610=EDGE_CURVE('',#2843,#2844,#197,.T.);
#3611=EDGE_CURVE('',#2844,#2845,#198,.T.);
#3612=EDGE_CURVE('',#2846,#2845,#2439,.T.);
#3613=EDGE_CURVE('',#2846,#2847,#199,.T.);
#3614=EDGE_CURVE('',#2847,#2848,#200,.T.);
#3615=EDGE_CURVE('',#2849,#2848,#2440,.T.);
#3616=EDGE_CURVE('',#2849,#2850,#201,.T.);
#3617=EDGE_CURVE('',#2850,#2851,#202,.T.);
#3618=EDGE_CURVE('',#2852,#2851,#2441,.T.);
#3619=EDGE_CURVE('',#2852,#2853,#203,.T.);
#3620=EDGE_CURVE('',#2853,#2854,#204,.T.);
#3621=EDGE_CURVE('',#2855,#2854,#2442,.T.);
#3622=EDGE_CURVE('',#2855,#2856,#205,.T.);
#3623=EDGE_CURVE('',#2856,#2857,#206,.T.);
#3624=EDGE_CURVE('',#2858,#2857,#2443,.T.);
#3625=EDGE_CURVE('',#2858,#2859,#207,.T.);
#3626=EDGE_CURVE('',#2859,#2860,#208,.T.);
#3627=EDGE_CURVE('',#2861,#2860,#2444,.T.);
#3628=EDGE_CURVE('',#2861,#2862,#209,.T.);
#3629=EDGE_CURVE('',#2862,#2863,#210,.T.);
#3630=EDGE_CURVE('',#2864,#2863,#2445,.T.);
#3631=EDGE_CURVE('',#2864,#2865,#211,.T.);
#3632=EDGE_CURVE('',#2865,#2866,#212,.T.);
#3633=EDGE_CURVE('',#2867,#2866,#2446,.T.);
#3634=EDGE_CURVE('',#2867,#2868,#213,.T.);
#3635=EDGE_CURVE('',#2868,#2812,#214,.T.);
#3636=EDGE_CURVE('',#2809,#2869,#1932,.T.);
#3637=EDGE_CURVE('',#2869,#2869,#2447,.T.);
#3638=EDGE_CURVE('',#2870,#2870,#2448,.T.);
#3639=EDGE_CURVE('',#2870,#2871,#1933,.T.);
#3640=EDGE_CURVE('',#2871,#2872,#2449,.T.);
#3641=EDGE_CURVE('',#2872,#2871,#2450,.T.);
#3642=EDGE_CURVE('',#2872,#2796,#1934,.T.);
#3643=EDGE_CURVE('',#2794,#2873,#1935,.T.);
#3644=EDGE_CURVE('',#2873,#2873,#2451,.T.);
#3645=EDGE_CURVE('',#2874,#2875,#347,.T.);
#3646=EDGE_CURVE('',#2876,#2874,#348,.T.);
#3647=EDGE_CURVE('',#2875,#2876,#2452,.T.);
#3648=EDGE_CURVE('',#2877,#2878,#349,.T.);
#3649=EDGE_CURVE('',#2879,#2877,#350,.T.);
#3650=EDGE_CURVE('',#2878,#2879,#2453,.T.);
#3651=EDGE_CURVE('',#2880,#2881,#351,.T.);
#3652=EDGE_CURVE('',#2882,#2880,#352,.T.);
#3653=EDGE_CURVE('',#2881,#2882,#2454,.T.);
#3654=EDGE_CURVE('',#2883,#2884,#353,.T.);
#3655=EDGE_CURVE('',#2885,#2883,#354,.T.);
#3656=EDGE_CURVE('',#2884,#2885,#2455,.T.);
#3657=EDGE_CURVE('',#2886,#2887,#355,.T.);
#3658=EDGE_CURVE('',#2888,#2886,#356,.T.);
#3659=EDGE_CURVE('',#2887,#2888,#2456,.T.);
#3660=EDGE_CURVE('',#2889,#2890,#357,.T.);
#3661=EDGE_CURVE('',#2891,#2889,#358,.T.);
#3662=EDGE_CURVE('',#2890,#2891,#2457,.T.);
#3663=EDGE_CURVE('',#2892,#2893,#359,.T.);
#3664=EDGE_CURVE('',#2894,#2892,#360,.T.);
#3665=EDGE_CURVE('',#2893,#2894,#2458,.T.);
#3666=EDGE_CURVE('',#2895,#2896,#361,.T.);
#3667=EDGE_CURVE('',#2897,#2895,#362,.T.);
#3668=EDGE_CURVE('',#2896,#2897,#2459,.T.);
#3669=EDGE_CURVE('',#2898,#2899,#363,.T.);
#3670=EDGE_CURVE('',#2900,#2898,#364,.T.);
#3671=EDGE_CURVE('',#2899,#2900,#2460,.T.);
#3672=EDGE_CURVE('',#2901,#2902,#365,.T.);
#3673=EDGE_CURVE('',#2903,#2901,#366,.T.);
#3674=EDGE_CURVE('',#2902,#2903,#2461,.T.);
#3675=EDGE_CURVE('',#2904,#2905,#367,.T.);
#3676=EDGE_CURVE('',#2906,#2904,#368,.T.);
#3677=EDGE_CURVE('',#2905,#2906,#2462,.T.);
#3678=EDGE_CURVE('',#2907,#2908,#369,.T.);
#3679=EDGE_CURVE('',#2909,#2907,#370,.T.);
#3680=EDGE_CURVE('',#2908,#2909,#2463,.T.);
#3681=EDGE_CURVE('',#2910,#2911,#371,.T.);
#3682=EDGE_CURVE('',#2912,#2910,#372,.T.);
#3683=EDGE_CURVE('',#2911,#2912,#2464,.T.);
#3684=EDGE_CURVE('',#2913,#2914,#373,.T.);
#3685=EDGE_CURVE('',#2915,#2913,#374,.T.);
#3686=EDGE_CURVE('',#2914,#2915,#2465,.T.);
#3687=EDGE_CURVE('',#2916,#2917,#375,.T.);
#3688=EDGE_CURVE('',#2918,#2916,#376,.T.);
#3689=EDGE_CURVE('',#2917,#2918,#2466,.T.);
#3690=EDGE_CURVE('',#2919,#2920,#377,.T.);
#3691=EDGE_CURVE('',#2921,#2919,#378,.T.);
#3692=EDGE_CURVE('',#2920,#2921,#2467,.T.);
#3693=EDGE_CURVE('',#2922,#2923,#379,.T.);
#3694=EDGE_CURVE('',#2924,#2922,#380,.T.);
#3695=EDGE_CURVE('',#2923,#2924,#2468,.T.);
#3696=EDGE_CURVE('',#2925,#2926,#381,.T.);
#3697=EDGE_CURVE('',#2927,#2925,#382,.T.);
#3698=EDGE_CURVE('',#2926,#2927,#2469,.T.);
#3699=EDGE_CURVE('',#2928,#2929,#383,.T.);
#3700=EDGE_CURVE('',#2930,#2928,#384,.T.);
#3701=EDGE_CURVE('',#2929,#2930,#2470,.T.);
#3702=EDGE_CURVE('',#2931,#2931,#2471,.T.);
#3703=EDGE_CURVE('',#2931,#2932,#1936,.T.);
#3704=EDGE_CURVE('',#2932,#2932,#2472,.T.);
#3705=EDGE_CURVE('',#2932,#2933,#1937,.T.);
#3706=EDGE_CURVE('',#2933,#2933,#2473,.T.);
#3707=EDGE_CURVE('',#2934,#2935,#385,.T.);
#3708=EDGE_CURVE('',#2936,#2934,#386,.T.);
#3709=EDGE_CURVE('',#2935,#2936,#2474,.T.);
#3710=EDGE_CURVE('',#2868,#2934,#1938,.T.);
#3711=EDGE_CURVE('',#2937,#2867,#387,.T.);
#3712=EDGE_CURVE('',#2937,#2936,#215,.T.);
#3713=EDGE_CURVE('',#2813,#2928,#1939,.T.);
#3714=EDGE_CURVE('',#2938,#2811,#388,.T.);
#3715=EDGE_CURVE('',#2938,#2930,#216,.T.);
#3716=EDGE_CURVE('',#2816,#2925,#1940,.T.);
#3717=EDGE_CURVE('',#2939,#2815,#389,.T.);
#3718=EDGE_CURVE('',#2939,#2927,#217,.T.);
#3719=EDGE_CURVE('',#2819,#2922,#1941,.T.);
#3720=EDGE_CURVE('',#2940,#2818,#390,.T.);
#3721=EDGE_CURVE('',#2940,#2924,#218,.T.);
#3722=EDGE_CURVE('',#2822,#2919,#1942,.T.);
#3723=EDGE_CURVE('',#2941,#2821,#391,.T.);
#3724=EDGE_CURVE('',#2941,#2921,#219,.T.);
#3725=EDGE_CURVE('',#2825,#2916,#1943,.T.);
#3726=EDGE_CURVE('',#2942,#2824,#392,.T.);
#3727=EDGE_CURVE('',#2942,#2918,#220,.T.);
#3728=EDGE_CURVE('',#2828,#2913,#1944,.T.);
#3729=EDGE_CURVE('',#2943,#2827,#393,.T.);
#3730=EDGE_CURVE('',#2943,#2915,#221,.T.);
#3731=EDGE_CURVE('',#2831,#2910,#1945,.T.);
#3732=EDGE_CURVE('',#2944,#2830,#394,.T.);
#3733=EDGE_CURVE('',#2944,#2912,#222,.T.);
#3734=EDGE_CURVE('',#2834,#2907,#1946,.T.);
#3735=EDGE_CURVE('',#2945,#2833,#395,.T.);
#3736=EDGE_CURVE('',#2945,#2909,#223,.T.);
#3737=EDGE_CURVE('',#2837,#2904,#1947,.T.);
#3738=EDGE_CURVE('',#2946,#2836,#396,.T.);
#3739=EDGE_CURVE('',#2946,#2906,#224,.T.);
#3740=EDGE_CURVE('',#2838,#2901,#1948,.T.);
#3741=EDGE_CURVE('',#2947,#2790,#397,.T.);
#3742=EDGE_CURVE('',#2947,#2903,#225,.T.);
#3743=EDGE_CURVE('',#2841,#2898,#1949,.T.);
#3744=EDGE_CURVE('',#2948,#2840,#398,.T.);
#3745=EDGE_CURVE('',#2948,#2900,#226,.T.);
#3746=EDGE_CURVE('',#2844,#2895,#1950,.T.);
#3747=EDGE_CURVE('',#2949,#2843,#399,.T.);
#3748=EDGE_CURVE('',#2949,#2897,#227,.T.);
#3749=EDGE_CURVE('',#2847,#2892,#1951,.T.);
#3750=EDGE_CURVE('',#2950,#2846,#400,.T.);
#3751=EDGE_CURVE('',#2950,#2894,#228,.T.);
#3752=EDGE_CURVE('',#2850,#2889,#1952,.T.);
#3753=EDGE_CURVE('',#2951,#2849,#401,.T.);
#3754=EDGE_CURVE('',#2951,#2891,#229,.T.);
#3755=EDGE_CURVE('',#2853,#2886,#1953,.T.);
#3756=EDGE_CURVE('',#2952,#2852,#402,.T.);
#3757=EDGE_CURVE('',#2952,#2888,#230,.T.);
#3758=EDGE_CURVE('',#2856,#2883,#1954,.T.);
#3759=EDGE_CURVE('',#2953,#2855,#403,.T.);
#3760=EDGE_CURVE('',#2953,#2885,#231,.T.);
#3761=EDGE_CURVE('',#2859,#2880,#1955,.T.);
#3762=EDGE_CURVE('',#2954,#2858,#404,.T.);
#3763=EDGE_CURVE('',#2954,#2882,#232,.T.);
#3764=EDGE_CURVE('',#2862,#2877,#1956,.T.);
#3765=EDGE_CURVE('',#2955,#2861,#405,.T.);
#3766=EDGE_CURVE('',#2955,#2879,#233,.T.);
#3767=EDGE_CURVE('',#2865,#2874,#1957,.T.);
#3768=EDGE_CURVE('',#2956,#2864,#406,.T.);
#3769=EDGE_CURVE('',#2956,#2876,#234,.T.);
#3770=EDGE_CURVE('',#2935,#2957,#235,.T.);
#3771=EDGE_CURVE('',#2812,#2957,#407,.T.);
#3772=EDGE_CURVE('',#2957,#2937,#2475,.T.);
#3773=EDGE_CURVE('',#2931,#2958,#1958,.T.);
#3774=EDGE_CURVE('',#2958,#2947,#2476,.T.);
#3775=EDGE_CURVE('',#2791,#2959,#408,.T.);
#3776=EDGE_CURVE('',#2959,#2946,#2477,.T.);
#3777=EDGE_CURVE('',#2835,#2960,#409,.T.);
#3778=EDGE_CURVE('',#2960,#2945,#2478,.T.);
#3779=EDGE_CURVE('',#2832,#2961,#410,.T.);
#3780=EDGE_CURVE('',#2961,#2944,#2479,.T.);
#3781=EDGE_CURVE('',#2829,#2962,#411,.T.);
#3782=EDGE_CURVE('',#2962,#2943,#2480,.T.);
#3783=EDGE_CURVE('',#2826,#2963,#412,.T.);
#3784=EDGE_CURVE('',#2963,#2942,#2481,.T.);
#3785=EDGE_CURVE('',#2823,#2964,#413,.T.);
#3786=EDGE_CURVE('',#2964,#2941,#2482,.T.);
#3787=EDGE_CURVE('',#2820,#2965,#414,.T.);
#3788=EDGE_CURVE('',#2965,#2940,#2483,.T.);
#3789=EDGE_CURVE('',#2817,#2966,#415,.T.);
#3790=EDGE_CURVE('',#2966,#2939,#2484,.T.);
#3791=EDGE_CURVE('',#2814,#2967,#416,.T.);
#3792=EDGE_CURVE('',#2967,#2938,#2485,.T.);
#3793=EDGE_CURVE('',#2866,#2968,#417,.T.);
#3794=EDGE_CURVE('',#2968,#2956,#2486,.T.);
#3795=EDGE_CURVE('',#2863,#2969,#418,.T.);
#3796=EDGE_CURVE('',#2969,#2955,#2487,.T.);
#3797=EDGE_CURVE('',#2860,#2970,#419,.T.);
#3798=EDGE_CURVE('',#2970,#2954,#2488,.T.);
#3799=EDGE_CURVE('',#2857,#2971,#420,.T.);
#3800=EDGE_CURVE('',#2971,#2953,#2489,.T.);
#3801=EDGE_CURVE('',#2854,#2972,#421,.T.);
#3802=EDGE_CURVE('',#2972,#2952,#2490,.T.);
#3803=EDGE_CURVE('',#2851,#2973,#422,.T.);
#3804=EDGE_CURVE('',#2973,#2951,#2491,.T.);
#3805=EDGE_CURVE('',#2848,#2974,#423,.T.);
#3806=EDGE_CURVE('',#2974,#2950,#2492,.T.);
#3807=EDGE_CURVE('',#2845,#2975,#424,.T.);
#3808=EDGE_CURVE('',#2975,#2949,#2493,.T.);
#3809=EDGE_CURVE('',#2842,#2976,#425,.T.);
#3810=EDGE_CURVE('',#2976,#2948,#2494,.T.);
#3811=EDGE_CURVE('',#2839,#2977,#426,.T.);
#3812=EDGE_CURVE('',#2977,#2958,#2495,.T.);
#3813=EDGE_CURVE('',#2929,#2967,#236,.T.);
#3814=EDGE_CURVE('',#2926,#2966,#237,.T.);
#3815=EDGE_CURVE('',#2923,#2965,#238,.T.);
#3816=EDGE_CURVE('',#2920,#2964,#239,.T.);
#3817=EDGE_CURVE('',#2917,#2963,#240,.T.);
#3818=EDGE_CURVE('',#2914,#2962,#241,.T.);
#3819=EDGE_CURVE('',#2911,#2961,#242,.T.);
#3820=EDGE_CURVE('',#2908,#2960,#243,.T.);
#3821=EDGE_CURVE('',#2905,#2959,#244,.T.);
#3822=EDGE_CURVE('',#2902,#2977,#245,.T.);
#3823=EDGE_CURVE('',#2899,#2976,#246,.T.);
#3824=EDGE_CURVE('',#2896,#2975,#247,.T.);
#3825=EDGE_CURVE('',#2893,#2974,#248,.T.);
#3826=EDGE_CURVE('',#2890,#2973,#249,.T.);
#3827=EDGE_CURVE('',#2887,#2972,#250,.T.);
#3828=EDGE_CURVE('',#2884,#2971,#251,.T.);
#3829=EDGE_CURVE('',#2881,#2970,#252,.T.);
#3830=EDGE_CURVE('',#2878,#2969,#253,.T.);
#3831=EDGE_CURVE('',#2875,#2968,#254,.T.);
#4747=ORIENTED_EDGE('',*,*,#3549,.F.);
#4748=ORIENTED_EDGE('',*,*,#3550,.T.);
#4749=ORIENTED_EDGE('',*,*,#3551,.T.);
#4750=ORIENTED_EDGE('',*,*,#3552,.T.);
#4751=ORIENTED_EDGE('',*,*,#3553,.F.);
#4752=ORIENTED_EDGE('',*,*,#3554,.F.);
#4753=ORIENTED_EDGE('',*,*,#3555,.F.);
#4754=ORIENTED_EDGE('',*,*,#3556,.T.);
#4755=ORIENTED_EDGE('',*,*,#3557,.T.);
#4756=ORIENTED_EDGE('',*,*,#3556,.F.);
#4757=ORIENTED_EDGE('',*,*,#3557,.F.);
#4758=ORIENTED_EDGE('',*,*,#3558,.T.);
#4759=ORIENTED_EDGE('',*,*,#3559,.F.);
#4760=ORIENTED_EDGE('',*,*,#3560,.F.);
#4761=ORIENTED_EDGE('',*,*,#3561,.F.);
#4762=ORIENTED_EDGE('',*,*,#3558,.F.);
#4763=ORIENTED_EDGE('',*,*,#3562,.F.);
#4764=ORIENTED_EDGE('',*,*,#3563,.T.);
#4765=ORIENTED_EDGE('',*,*,#3564,.T.);
#4766=ORIENTED_EDGE('',*,*,#3563,.F.);
#4767=ORIENTED_EDGE('',*,*,#3565,.F.);
#4768=ORIENTED_EDGE('',*,*,#3564,.F.);
#4769=ORIENTED_EDGE('',*,*,#3566,.T.);
#4770=ORIENTED_EDGE('',*,*,#3567,.F.);
#4771=ORIENTED_EDGE('',*,*,#3568,.F.);
#4772=ORIENTED_EDGE('',*,*,#3566,.F.);
#4773=ORIENTED_EDGE('',*,*,#3569,.T.);
#4774=ORIENTED_EDGE('',*,*,#3570,.T.);
#4775=ORIENTED_EDGE('',*,*,#3571,.T.);
#4776=ORIENTED_EDGE('',*,*,#3572,.T.);
#4777=ORIENTED_EDGE('',*,*,#3570,.F.);
#4778=ORIENTED_EDGE('',*,*,#3573,.F.);
#4779=ORIENTED_EDGE('',*,*,#3574,.F.);
#4780=ORIENTED_EDGE('',*,*,#3575,.T.);
#4781=ORIENTED_EDGE('',*,*,#3559,.T.);
#4782=ORIENTED_EDGE('',*,*,#3561,.T.);
#4783=ORIENTED_EDGE('',*,*,#3576,.T.);
#4784=ORIENTED_EDGE('',*,*,#3571,.F.);
#4785=ORIENTED_EDGE('',*,*,#3572,.F.);
#4786=ORIENTED_EDGE('',*,*,#3576,.F.);
#4787=ORIENTED_EDGE('',*,*,#3560,.T.);
#4788=ORIENTED_EDGE('',*,*,#3575,.F.);
#4789=ORIENTED_EDGE('',*,*,#3567,.T.);
#4790=ORIENTED_EDGE('',*,*,#3568,.T.);
#4791=ORIENTED_EDGE('',*,*,#3577,.F.);
#4792=ORIENTED_EDGE('',*,*,#3578,.T.);
#4793=ORIENTED_EDGE('',*,*,#3579,.T.);
#4794=ORIENTED_EDGE('',*,*,#3580,.F.);
#4795=ORIENTED_EDGE('',*,*,#3581,.T.);
#4796=ORIENTED_EDGE('',*,*,#3582,.T.);
#4797=ORIENTED_EDGE('',*,*,#3583,.F.);
#4798=ORIENTED_EDGE('',*,*,#3584,.T.);
#4799=ORIENTED_EDGE('',*,*,#3585,.T.);
#4800=ORIENTED_EDGE('',*,*,#3586,.F.);
#4801=ORIENTED_EDGE('',*,*,#3587,.T.);
#4802=ORIENTED_EDGE('',*,*,#3588,.T.);
#4803=ORIENTED_EDGE('',*,*,#3589,.F.);
#4804=ORIENTED_EDGE('',*,*,#3590,.T.);
#4805=ORIENTED_EDGE('',*,*,#3591,.T.);
#4806=ORIENTED_EDGE('',*,*,#3592,.F.);
#4807=ORIENTED_EDGE('',*,*,#3593,.T.);
#4808=ORIENTED_EDGE('',*,*,#3594,.T.);
#4809=ORIENTED_EDGE('',*,*,#3595,.F.);
#4810=ORIENTED_EDGE('',*,*,#3596,.T.);
#4811=ORIENTED_EDGE('',*,*,#3597,.T.);
#4812=ORIENTED_EDGE('',*,*,#3598,.F.);
#4813=ORIENTED_EDGE('',*,*,#3599,.T.);
#4814=ORIENTED_EDGE('',*,*,#3600,.T.);
#4815=ORIENTED_EDGE('',*,*,#3601,.F.);
#4816=ORIENTED_EDGE('',*,*,#3602,.T.);
#4817=ORIENTED_EDGE('',*,*,#3603,.T.);
#4818=ORIENTED_EDGE('',*,*,#3551,.F.);
#4819=ORIENTED_EDGE('',*,*,#3604,.T.);
#4820=ORIENTED_EDGE('',*,*,#3605,.T.);
#4821=ORIENTED_EDGE('',*,*,#3606,.F.);
#4822=ORIENTED_EDGE('',*,*,#3607,.T.);
#4823=ORIENTED_EDGE('',*,*,#3608,.T.);
#4824=ORIENTED_EDGE('',*,*,#3609,.F.);
#4825=ORIENTED_EDGE('',*,*,#3610,.T.);
#4826=ORIENTED_EDGE('',*,*,#3611,.T.);
#4827=ORIENTED_EDGE('',*,*,#3612,.F.);
#4828=ORIENTED_EDGE('',*,*,#3613,.T.);
#4829=ORIENTED_EDGE('',*,*,#3614,.T.);
#4830=ORIENTED_EDGE('',*,*,#3615,.F.);
#4831=ORIENTED_EDGE('',*,*,#3616,.T.);
#4832=ORIENTED_EDGE('',*,*,#3617,.T.);
#4833=ORIENTED_EDGE('',*,*,#3618,.F.);
#4834=ORIENTED_EDGE('',*,*,#3619,.T.);
#4835=ORIENTED_EDGE('',*,*,#3620,.T.);
#4836=ORIENTED_EDGE('',*,*,#3621,.F.);
#4837=ORIENTED_EDGE('',*,*,#3622,.T.);
#4838=ORIENTED_EDGE('',*,*,#3623,.T.);
#4839=ORIENTED_EDGE('',*,*,#3624,.F.);
#4840=ORIENTED_EDGE('',*,*,#3625,.T.);
#4841=ORIENTED_EDGE('',*,*,#3626,.T.);
#4842=ORIENTED_EDGE('',*,*,#3627,.F.);
#4843=ORIENTED_EDGE('',*,*,#3628,.T.);
#4844=ORIENTED_EDGE('',*,*,#3629,.T.);
#4845=ORIENTED_EDGE('',*,*,#3630,.F.);
#4846=ORIENTED_EDGE('',*,*,#3631,.T.);
#4847=ORIENTED_EDGE('',*,*,#3632,.T.);
#4848=ORIENTED_EDGE('',*,*,#3633,.F.);
#4849=ORIENTED_EDGE('',*,*,#3634,.T.);
#4850=ORIENTED_EDGE('',*,*,#3635,.T.);
#4851=ORIENTED_EDGE('',*,*,#3569,.F.);
#4852=ORIENTED_EDGE('',*,*,#3573,.T.);
#4853=ORIENTED_EDGE('',*,*,#3574,.T.);
#4854=ORIENTED_EDGE('',*,*,#3636,.T.);
#4855=ORIENTED_EDGE('',*,*,#3637,.T.);
#4856=ORIENTED_EDGE('',*,*,#3636,.F.);
#4857=ORIENTED_EDGE('',*,*,#3638,.F.);
#4858=ORIENTED_EDGE('',*,*,#3637,.F.);
#4859=ORIENTED_EDGE('',*,*,#3638,.T.);
#4860=ORIENTED_EDGE('',*,*,#3639,.T.);
#4861=ORIENTED_EDGE('',*,*,#3640,.T.);
#4862=ORIENTED_EDGE('',*,*,#3641,.T.);
#4863=ORIENTED_EDGE('',*,*,#3639,.F.);
#4864=ORIENTED_EDGE('',*,*,#3640,.F.);
#4865=ORIENTED_EDGE('',*,*,#3641,.F.);
#4866=ORIENTED_EDGE('',*,*,#3642,.T.);
#4867=ORIENTED_EDGE('',*,*,#3554,.T.);
#4868=ORIENTED_EDGE('',*,*,#3643,.T.);
#4869=ORIENTED_EDGE('',*,*,#3644,.T.);
#4870=ORIENTED_EDGE('',*,*,#3643,.F.);
#4871=ORIENTED_EDGE('',*,*,#3553,.T.);
#4872=ORIENTED_EDGE('',*,*,#3555,.T.);
#4873=ORIENTED_EDGE('',*,*,#3642,.F.);
#4874=ORIENTED_EDGE('',*,*,#3562,.T.);
#4875=ORIENTED_EDGE('',*,*,#3565,.T.);
#4876=ORIENTED_EDGE('',*,*,#3645,.F.);
#4877=ORIENTED_EDGE('',*,*,#3646,.F.);
#4878=ORIENTED_EDGE('',*,*,#3647,.F.);
#4879=ORIENTED_EDGE('',*,*,#3648,.F.);
#4880=ORIENTED_EDGE('',*,*,#3649,.F.);
#4881=ORIENTED_EDGE('',*,*,#3650,.F.);
#4882=ORIENTED_EDGE('',*,*,#3651,.F.);
#4883=ORIENTED_EDGE('',*,*,#3652,.F.);
#4884=ORIENTED_EDGE('',*,*,#3653,.F.);
#4885=ORIENTED_EDGE('',*,*,#3654,.F.);
#4886=ORIENTED_EDGE('',*,*,#3655,.F.);
#4887=ORIENTED_EDGE('',*,*,#3656,.F.);
#4888=ORIENTED_EDGE('',*,*,#3657,.F.);
#4889=ORIENTED_EDGE('',*,*,#3658,.F.);
#4890=ORIENTED_EDGE('',*,*,#3659,.F.);
#4891=ORIENTED_EDGE('',*,*,#3660,.F.);
#4892=ORIENTED_EDGE('',*,*,#3661,.F.);
#4893=ORIENTED_EDGE('',*,*,#3662,.F.);
#4894=ORIENTED_EDGE('',*,*,#3663,.F.);
#4895=ORIENTED_EDGE('',*,*,#3664,.F.);
#4896=ORIENTED_EDGE('',*,*,#3665,.F.);
#4897=ORIENTED_EDGE('',*,*,#3666,.F.);
#4898=ORIENTED_EDGE('',*,*,#3667,.F.);
#4899=ORIENTED_EDGE('',*,*,#3668,.F.);
#4900=ORIENTED_EDGE('',*,*,#3669,.F.);
#4901=ORIENTED_EDGE('',*,*,#3670,.F.);
#4902=ORIENTED_EDGE('',*,*,#3671,.F.);
#4903=ORIENTED_EDGE('',*,*,#3672,.F.);
#4904=ORIENTED_EDGE('',*,*,#3673,.F.);
#4905=ORIENTED_EDGE('',*,*,#3674,.F.);
#4906=ORIENTED_EDGE('',*,*,#3675,.F.);
#4907=ORIENTED_EDGE('',*,*,#3676,.F.);
#4908=ORIENTED_EDGE('',*,*,#3677,.F.);
#4909=ORIENTED_EDGE('',*,*,#3678,.F.);
#4910=ORIENTED_EDGE('',*,*,#3679,.F.);
#4911=ORIENTED_EDGE('',*,*,#3680,.F.);
#4912=ORIENTED_EDGE('',*,*,#3681,.F.);
#4913=ORIENTED_EDGE('',*,*,#3682,.F.);
#4914=ORIENTED_EDGE('',*,*,#3683,.F.);
#4915=ORIENTED_EDGE('',*,*,#3684,.F.);
#4916=ORIENTED_EDGE('',*,*,#3685,.F.);
#4917=ORIENTED_EDGE('',*,*,#3686,.F.);
#4918=ORIENTED_EDGE('',*,*,#3687,.F.);
#4919=ORIENTED_EDGE('',*,*,#3688,.F.);
#4920=ORIENTED_EDGE('',*,*,#3689,.F.);
#4921=ORIENTED_EDGE('',*,*,#3690,.F.);
#4922=ORIENTED_EDGE('',*,*,#3691,.F.);
#4923=ORIENTED_EDGE('',*,*,#3692,.F.);
#4924=ORIENTED_EDGE('',*,*,#3693,.F.);
#4925=ORIENTED_EDGE('',*,*,#3694,.F.);
#4926=ORIENTED_EDGE('',*,*,#3695,.F.);
#4927=ORIENTED_EDGE('',*,*,#3696,.F.);
#4928=ORIENTED_EDGE('',*,*,#3697,.F.);
#4929=ORIENTED_EDGE('',*,*,#3698,.F.);
#4930=ORIENTED_EDGE('',*,*,#3699,.F.);
#4931=ORIENTED_EDGE('',*,*,#3700,.F.);
#4932=ORIENTED_EDGE('',*,*,#3701,.F.);
#4933=ORIENTED_EDGE('',*,*,#3702,.F.);
#4934=ORIENTED_EDGE('',*,*,#3703,.T.);
#4935=ORIENTED_EDGE('',*,*,#3704,.F.);
#4936=ORIENTED_EDGE('',*,*,#3703,.F.);
#4937=ORIENTED_EDGE('',*,*,#3704,.T.);
#4938=ORIENTED_EDGE('',*,*,#3705,.T.);
#4939=ORIENTED_EDGE('',*,*,#3706,.F.);
#4940=ORIENTED_EDGE('',*,*,#3705,.F.);
#4941=ORIENTED_EDGE('',*,*,#3707,.F.);
#4942=ORIENTED_EDGE('',*,*,#3708,.F.);
#4943=ORIENTED_EDGE('',*,*,#3709,.F.);
#4944=ORIENTED_EDGE('',*,*,#3708,.T.);
#4945=ORIENTED_EDGE('',*,*,#3710,.F.);
#4946=ORIENTED_EDGE('',*,*,#3634,.F.);
#4947=ORIENTED_EDGE('',*,*,#3711,.F.);
#4948=ORIENTED_EDGE('',*,*,#3712,.T.);
#4949=ORIENTED_EDGE('',*,*,#3700,.T.);
#4950=ORIENTED_EDGE('',*,*,#3713,.F.);
#4951=ORIENTED_EDGE('',*,*,#3578,.F.);
#4952=ORIENTED_EDGE('',*,*,#3714,.F.);
#4953=ORIENTED_EDGE('',*,*,#3715,.T.);
#4954=ORIENTED_EDGE('',*,*,#3697,.T.);
#4955=ORIENTED_EDGE('',*,*,#3716,.F.);
#4956=ORIENTED_EDGE('',*,*,#3581,.F.);
#4957=ORIENTED_EDGE('',*,*,#3717,.F.);
#4958=ORIENTED_EDGE('',*,*,#3718,.T.);
#4959=ORIENTED_EDGE('',*,*,#3694,.T.);
#4960=ORIENTED_EDGE('',*,*,#3719,.F.);
#4961=ORIENTED_EDGE('',*,*,#3584,.F.);
#4962=ORIENTED_EDGE('',*,*,#3720,.F.);
#4963=ORIENTED_EDGE('',*,*,#3721,.T.);
#4964=ORIENTED_EDGE('',*,*,#3691,.T.);
#4965=ORIENTED_EDGE('',*,*,#3722,.F.);
#4966=ORIENTED_EDGE('',*,*,#3587,.F.);
#4967=ORIENTED_EDGE('',*,*,#3723,.F.);
#4968=ORIENTED_EDGE('',*,*,#3724,.T.);
#4969=ORIENTED_EDGE('',*,*,#3688,.T.);
#4970=ORIENTED_EDGE('',*,*,#3725,.F.);
#4971=ORIENTED_EDGE('',*,*,#3590,.F.);
#4972=ORIENTED_EDGE('',*,*,#3726,.F.);
#4973=ORIENTED_EDGE('',*,*,#3727,.T.);
#4974=ORIENTED_EDGE('',*,*,#3685,.T.);
#4975=ORIENTED_EDGE('',*,*,#3728,.F.);
#4976=ORIENTED_EDGE('',*,*,#3593,.F.);
#4977=ORIENTED_EDGE('',*,*,#3729,.F.);
#4978=ORIENTED_EDGE('',*,*,#3730,.T.);
#4979=ORIENTED_EDGE('',*,*,#3682,.T.);
#4980=ORIENTED_EDGE('',*,*,#3731,.F.);
#4981=ORIENTED_EDGE('',*,*,#3596,.F.);
#4982=ORIENTED_EDGE('',*,*,#3732,.F.);
#4983=ORIENTED_EDGE('',*,*,#3733,.T.);
#4984=ORIENTED_EDGE('',*,*,#3679,.T.);
#4985=ORIENTED_EDGE('',*,*,#3734,.F.);
#4986=ORIENTED_EDGE('',*,*,#3599,.F.);
#4987=ORIENTED_EDGE('',*,*,#3735,.F.);
#4988=ORIENTED_EDGE('',*,*,#3736,.T.);
#4989=ORIENTED_EDGE('',*,*,#3676,.T.);
#4990=ORIENTED_EDGE('',*,*,#3737,.F.);
#4991=ORIENTED_EDGE('',*,*,#3602,.F.);
#4992=ORIENTED_EDGE('',*,*,#3738,.F.);
#4993=ORIENTED_EDGE('',*,*,#3739,.T.);
#4994=ORIENTED_EDGE('',*,*,#3673,.T.);
#4995=ORIENTED_EDGE('',*,*,#3740,.F.);
#4996=ORIENTED_EDGE('',*,*,#3604,.F.);
#4997=ORIENTED_EDGE('',*,*,#3550,.F.);
#4998=ORIENTED_EDGE('',*,*,#3741,.F.);
#4999=ORIENTED_EDGE('',*,*,#3742,.T.);
#5000=ORIENTED_EDGE('',*,*,#3670,.T.);
#5001=ORIENTED_EDGE('',*,*,#3743,.F.);
#5002=ORIENTED_EDGE('',*,*,#3607,.F.);
#5003=ORIENTED_EDGE('',*,*,#3744,.F.);
#5004=ORIENTED_EDGE('',*,*,#3745,.T.);
#5005=ORIENTED_EDGE('',*,*,#3667,.T.);
#5006=ORIENTED_EDGE('',*,*,#3746,.F.);
#5007=ORIENTED_EDGE('',*,*,#3610,.F.);
#5008=ORIENTED_EDGE('',*,*,#3747,.F.);
#5009=ORIENTED_EDGE('',*,*,#3748,.T.);
#5010=ORIENTED_EDGE('',*,*,#3664,.T.);
#5011=ORIENTED_EDGE('',*,*,#3749,.F.);
#5012=ORIENTED_EDGE('',*,*,#3613,.F.);
#5013=ORIENTED_EDGE('',*,*,#3750,.F.);
#5014=ORIENTED_EDGE('',*,*,#3751,.T.);
#5015=ORIENTED_EDGE('',*,*,#3661,.T.);
#5016=ORIENTED_EDGE('',*,*,#3752,.F.);
#5017=ORIENTED_EDGE('',*,*,#3616,.F.);
#5018=ORIENTED_EDGE('',*,*,#3753,.F.);
#5019=ORIENTED_EDGE('',*,*,#3754,.T.);
#5020=ORIENTED_EDGE('',*,*,#3658,.T.);
#5021=ORIENTED_EDGE('',*,*,#3755,.F.);
#5022=ORIENTED_EDGE('',*,*,#3619,.F.);
#5023=ORIENTED_EDGE('',*,*,#3756,.F.);
#5024=ORIENTED_EDGE('',*,*,#3757,.T.);
#5025=ORIENTED_EDGE('',*,*,#3655,.T.);
#5026=ORIENTED_EDGE('',*,*,#3758,.F.);
#5027=ORIENTED_EDGE('',*,*,#3622,.F.);
#5028=ORIENTED_EDGE('',*,*,#3759,.F.);
#5029=ORIENTED_EDGE('',*,*,#3760,.T.);
#5030=ORIENTED_EDGE('',*,*,#3652,.T.);
#5031=ORIENTED_EDGE('',*,*,#3761,.F.);
#5032=ORIENTED_EDGE('',*,*,#3625,.F.);
#5033=ORIENTED_EDGE('',*,*,#3762,.F.);
#5034=ORIENTED_EDGE('',*,*,#3763,.T.);
#5035=ORIENTED_EDGE('',*,*,#3649,.T.);
#5036=ORIENTED_EDGE('',*,*,#3764,.F.);
#5037=ORIENTED_EDGE('',*,*,#3628,.F.);
#5038=ORIENTED_EDGE('',*,*,#3765,.F.);
#5039=ORIENTED_EDGE('',*,*,#3766,.T.);
#5040=ORIENTED_EDGE('',*,*,#3646,.T.);
#5041=ORIENTED_EDGE('',*,*,#3767,.F.);
#5042=ORIENTED_EDGE('',*,*,#3631,.F.);
#5043=ORIENTED_EDGE('',*,*,#3768,.F.);
#5044=ORIENTED_EDGE('',*,*,#3769,.T.);
#5045=ORIENTED_EDGE('',*,*,#3707,.T.);
#5046=ORIENTED_EDGE('',*,*,#3770,.T.);
#5047=ORIENTED_EDGE('',*,*,#3771,.F.);
#5048=ORIENTED_EDGE('',*,*,#3635,.F.);
#5049=ORIENTED_EDGE('',*,*,#3710,.T.);
#5050=ORIENTED_EDGE('',*,*,#3709,.T.);
#5051=ORIENTED_EDGE('',*,*,#3712,.F.);
#5052=ORIENTED_EDGE('',*,*,#3772,.F.);
#5053=ORIENTED_EDGE('',*,*,#3770,.F.);
#5054=ORIENTED_EDGE('',*,*,#3702,.T.);
#5055=ORIENTED_EDGE('',*,*,#3773,.T.);
#5056=ORIENTED_EDGE('',*,*,#3774,.T.);
#5057=ORIENTED_EDGE('',*,*,#3741,.T.);
#5058=ORIENTED_EDGE('',*,*,#3549,.T.);
#5059=ORIENTED_EDGE('',*,*,#3775,.T.);
#5060=ORIENTED_EDGE('',*,*,#3776,.T.);
#5061=ORIENTED_EDGE('',*,*,#3738,.T.);
#5062=ORIENTED_EDGE('',*,*,#3601,.T.);
#5063=ORIENTED_EDGE('',*,*,#3777,.T.);
#5064=ORIENTED_EDGE('',*,*,#3778,.T.);
#5065=ORIENTED_EDGE('',*,*,#3735,.T.);
#5066=ORIENTED_EDGE('',*,*,#3598,.T.);
#5067=ORIENTED_EDGE('',*,*,#3779,.T.);
#5068=ORIENTED_EDGE('',*,*,#3780,.T.);
#5069=ORIENTED_EDGE('',*,*,#3732,.T.);
#5070=ORIENTED_EDGE('',*,*,#3595,.T.);
#5071=ORIENTED_EDGE('',*,*,#3781,.T.);
#5072=ORIENTED_EDGE('',*,*,#3782,.T.);
#5073=ORIENTED_EDGE('',*,*,#3729,.T.);
#5074=ORIENTED_EDGE('',*,*,#3592,.T.);
#5075=ORIENTED_EDGE('',*,*,#3783,.T.);
#5076=ORIENTED_EDGE('',*,*,#3784,.T.);
#5077=ORIENTED_EDGE('',*,*,#3726,.T.);
#5078=ORIENTED_EDGE('',*,*,#3589,.T.);
#5079=ORIENTED_EDGE('',*,*,#3785,.T.);
#5080=ORIENTED_EDGE('',*,*,#3786,.T.);
#5081=ORIENTED_EDGE('',*,*,#3723,.T.);
#5082=ORIENTED_EDGE('',*,*,#3586,.T.);
#5083=ORIENTED_EDGE('',*,*,#3787,.T.);
#5084=ORIENTED_EDGE('',*,*,#3788,.T.);
#5085=ORIENTED_EDGE('',*,*,#3720,.T.);
#5086=ORIENTED_EDGE('',*,*,#3583,.T.);
#5087=ORIENTED_EDGE('',*,*,#3789,.T.);
#5088=ORIENTED_EDGE('',*,*,#3790,.T.);
#5089=ORIENTED_EDGE('',*,*,#3717,.T.);
#5090=ORIENTED_EDGE('',*,*,#3580,.T.);
#5091=ORIENTED_EDGE('',*,*,#3791,.T.);
#5092=ORIENTED_EDGE('',*,*,#3792,.T.);
#5093=ORIENTED_EDGE('',*,*,#3714,.T.);
#5094=ORIENTED_EDGE('',*,*,#3577,.T.);
#5095=ORIENTED_EDGE('',*,*,#3771,.T.);
#5096=ORIENTED_EDGE('',*,*,#3772,.T.);
#5097=ORIENTED_EDGE('',*,*,#3711,.T.);
#5098=ORIENTED_EDGE('',*,*,#3633,.T.);
#5099=ORIENTED_EDGE('',*,*,#3793,.T.);
#5100=ORIENTED_EDGE('',*,*,#3794,.T.);
#5101=ORIENTED_EDGE('',*,*,#3768,.T.);
#5102=ORIENTED_EDGE('',*,*,#3630,.T.);
#5103=ORIENTED_EDGE('',*,*,#3795,.T.);
#5104=ORIENTED_EDGE('',*,*,#3796,.T.);
#5105=ORIENTED_EDGE('',*,*,#3765,.T.);
#5106=ORIENTED_EDGE('',*,*,#3627,.T.);
#5107=ORIENTED_EDGE('',*,*,#3797,.T.);
#5108=ORIENTED_EDGE('',*,*,#3798,.T.);
#5109=ORIENTED_EDGE('',*,*,#3762,.T.);
#5110=ORIENTED_EDGE('',*,*,#3624,.T.);
#5111=ORIENTED_EDGE('',*,*,#3799,.T.);
#5112=ORIENTED_EDGE('',*,*,#3800,.T.);
#5113=ORIENTED_EDGE('',*,*,#3759,.T.);
#5114=ORIENTED_EDGE('',*,*,#3621,.T.);
#5115=ORIENTED_EDGE('',*,*,#3801,.T.);
#5116=ORIENTED_EDGE('',*,*,#3802,.T.);
#5117=ORIENTED_EDGE('',*,*,#3756,.T.);
#5118=ORIENTED_EDGE('',*,*,#3618,.T.);
#5119=ORIENTED_EDGE('',*,*,#3803,.T.);
#5120=ORIENTED_EDGE('',*,*,#3804,.T.);
#5121=ORIENTED_EDGE('',*,*,#3753,.T.);
#5122=ORIENTED_EDGE('',*,*,#3615,.T.);
#5123=ORIENTED_EDGE('',*,*,#3805,.T.);
#5124=ORIENTED_EDGE('',*,*,#3806,.T.);
#5125=ORIENTED_EDGE('',*,*,#3750,.T.);
#5126=ORIENTED_EDGE('',*,*,#3612,.T.);
#5127=ORIENTED_EDGE('',*,*,#3807,.T.);
#5128=ORIENTED_EDGE('',*,*,#3808,.T.);
#5129=ORIENTED_EDGE('',*,*,#3747,.T.);
#5130=ORIENTED_EDGE('',*,*,#3609,.T.);
#5131=ORIENTED_EDGE('',*,*,#3809,.T.);
#5132=ORIENTED_EDGE('',*,*,#3810,.T.);
#5133=ORIENTED_EDGE('',*,*,#3744,.T.);
#5134=ORIENTED_EDGE('',*,*,#3606,.T.);
#5135=ORIENTED_EDGE('',*,*,#3811,.T.);
#5136=ORIENTED_EDGE('',*,*,#3812,.T.);
#5137=ORIENTED_EDGE('',*,*,#3773,.F.);
#5138=ORIENTED_EDGE('',*,*,#3699,.T.);
#5139=ORIENTED_EDGE('',*,*,#3813,.T.);
#5140=ORIENTED_EDGE('',*,*,#3791,.F.);
#5141=ORIENTED_EDGE('',*,*,#3579,.F.);
#5142=ORIENTED_EDGE('',*,*,#3713,.T.);
#5143=ORIENTED_EDGE('',*,*,#3701,.T.);
#5144=ORIENTED_EDGE('',*,*,#3715,.F.);
#5145=ORIENTED_EDGE('',*,*,#3792,.F.);
#5146=ORIENTED_EDGE('',*,*,#3813,.F.);
#5147=ORIENTED_EDGE('',*,*,#3696,.T.);
#5148=ORIENTED_EDGE('',*,*,#3814,.T.);
#5149=ORIENTED_EDGE('',*,*,#3789,.F.);
#5150=ORIENTED_EDGE('',*,*,#3582,.F.);
#5151=ORIENTED_EDGE('',*,*,#3716,.T.);
#5152=ORIENTED_EDGE('',*,*,#3698,.T.);
#5153=ORIENTED_EDGE('',*,*,#3718,.F.);
#5154=ORIENTED_EDGE('',*,*,#3790,.F.);
#5155=ORIENTED_EDGE('',*,*,#3814,.F.);
#5156=ORIENTED_EDGE('',*,*,#3693,.T.);
#5157=ORIENTED_EDGE('',*,*,#3815,.T.);
#5158=ORIENTED_EDGE('',*,*,#3787,.F.);
#5159=ORIENTED_EDGE('',*,*,#3585,.F.);
#5160=ORIENTED_EDGE('',*,*,#3719,.T.);
#5161=ORIENTED_EDGE('',*,*,#3695,.T.);
#5162=ORIENTED_EDGE('',*,*,#3721,.F.);
#5163=ORIENTED_EDGE('',*,*,#3788,.F.);
#5164=ORIENTED_EDGE('',*,*,#3815,.F.);
#5165=ORIENTED_EDGE('',*,*,#3690,.T.);
#5166=ORIENTED_EDGE('',*,*,#3816,.T.);
#5167=ORIENTED_EDGE('',*,*,#3785,.F.);
#5168=ORIENTED_EDGE('',*,*,#3588,.F.);
#5169=ORIENTED_EDGE('',*,*,#3722,.T.);
#5170=ORIENTED_EDGE('',*,*,#3692,.T.);
#5171=ORIENTED_EDGE('',*,*,#3724,.F.);
#5172=ORIENTED_EDGE('',*,*,#3786,.F.);
#5173=ORIENTED_EDGE('',*,*,#3816,.F.);
#5174=ORIENTED_EDGE('',*,*,#3687,.T.);
#5175=ORIENTED_EDGE('',*,*,#3817,.T.);
#5176=ORIENTED_EDGE('',*,*,#3783,.F.);
#5177=ORIENTED_EDGE('',*,*,#3591,.F.);
#5178=ORIENTED_EDGE('',*,*,#3725,.T.);
#5179=ORIENTED_EDGE('',*,*,#3689,.T.);
#5180=ORIENTED_EDGE('',*,*,#3727,.F.);
#5181=ORIENTED_EDGE('',*,*,#3784,.F.);
#5182=ORIENTED_EDGE('',*,*,#3817,.F.);
#5183=ORIENTED_EDGE('',*,*,#3684,.T.);
#5184=ORIENTED_EDGE('',*,*,#3818,.T.);
#5185=ORIENTED_EDGE('',*,*,#3781,.F.);
#5186=ORIENTED_EDGE('',*,*,#3594,.F.);
#5187=ORIENTED_EDGE('',*,*,#3728,.T.);
#5188=ORIENTED_EDGE('',*,*,#3686,.T.);
#5189=ORIENTED_EDGE('',*,*,#3730,.F.);
#5190=ORIENTED_EDGE('',*,*,#3782,.F.);
#5191=ORIENTED_EDGE('',*,*,#3818,.F.);
#5192=ORIENTED_EDGE('',*,*,#3681,.T.);
#5193=ORIENTED_EDGE('',*,*,#3819,.T.);
#5194=ORIENTED_EDGE('',*,*,#3779,.F.);
#5195=ORIENTED_EDGE('',*,*,#3597,.F.);
#5196=ORIENTED_EDGE('',*,*,#3731,.T.);
#5197=ORIENTED_EDGE('',*,*,#3683,.T.);
#5198=ORIENTED_EDGE('',*,*,#3733,.F.);
#5199=ORIENTED_EDGE('',*,*,#3780,.F.);
#5200=ORIENTED_EDGE('',*,*,#3819,.F.);
#5201=ORIENTED_EDGE('',*,*,#3678,.T.);
#5202=ORIENTED_EDGE('',*,*,#3820,.T.);
#5203=ORIENTED_EDGE('',*,*,#3777,.F.);
#5204=ORIENTED_EDGE('',*,*,#3600,.F.);
#5205=ORIENTED_EDGE('',*,*,#3734,.T.);
#5206=ORIENTED_EDGE('',*,*,#3680,.T.);
#5207=ORIENTED_EDGE('',*,*,#3736,.F.);
#5208=ORIENTED_EDGE('',*,*,#3778,.F.);
#5209=ORIENTED_EDGE('',*,*,#3820,.F.);
#5210=ORIENTED_EDGE('',*,*,#3675,.T.);
#5211=ORIENTED_EDGE('',*,*,#3821,.T.);
#5212=ORIENTED_EDGE('',*,*,#3775,.F.);
#5213=ORIENTED_EDGE('',*,*,#3552,.F.);
#5214=ORIENTED_EDGE('',*,*,#3603,.F.);
#5215=ORIENTED_EDGE('',*,*,#3737,.T.);
#5216=ORIENTED_EDGE('',*,*,#3677,.T.);
#5217=ORIENTED_EDGE('',*,*,#3739,.F.);
#5218=ORIENTED_EDGE('',*,*,#3776,.F.);
#5219=ORIENTED_EDGE('',*,*,#3821,.F.);
#5220=ORIENTED_EDGE('',*,*,#3672,.T.);
#5221=ORIENTED_EDGE('',*,*,#3822,.T.);
#5222=ORIENTED_EDGE('',*,*,#3811,.F.);
#5223=ORIENTED_EDGE('',*,*,#3605,.F.);
#5224=ORIENTED_EDGE('',*,*,#3740,.T.);
#5225=ORIENTED_EDGE('',*,*,#3674,.T.);
#5226=ORIENTED_EDGE('',*,*,#3742,.F.);
#5227=ORIENTED_EDGE('',*,*,#3774,.F.);
#5228=ORIENTED_EDGE('',*,*,#3812,.F.);
#5229=ORIENTED_EDGE('',*,*,#3822,.F.);
#5230=ORIENTED_EDGE('',*,*,#3669,.T.);
#5231=ORIENTED_EDGE('',*,*,#3823,.T.);
#5232=ORIENTED_EDGE('',*,*,#3809,.F.);
#5233=ORIENTED_EDGE('',*,*,#3608,.F.);
#5234=ORIENTED_EDGE('',*,*,#3743,.T.);
#5235=ORIENTED_EDGE('',*,*,#3671,.T.);
#5236=ORIENTED_EDGE('',*,*,#3745,.F.);
#5237=ORIENTED_EDGE('',*,*,#3810,.F.);
#5238=ORIENTED_EDGE('',*,*,#3823,.F.);
#5239=ORIENTED_EDGE('',*,*,#3666,.T.);
#5240=ORIENTED_EDGE('',*,*,#3824,.T.);
#5241=ORIENTED_EDGE('',*,*,#3807,.F.);
#5242=ORIENTED_EDGE('',*,*,#3611,.F.);
#5243=ORIENTED_EDGE('',*,*,#3746,.T.);
#5244=ORIENTED_EDGE('',*,*,#3668,.T.);
#5245=ORIENTED_EDGE('',*,*,#3748,.F.);
#5246=ORIENTED_EDGE('',*,*,#3808,.F.);
#5247=ORIENTED_EDGE('',*,*,#3824,.F.);
#5248=ORIENTED_EDGE('',*,*,#3663,.T.);
#5249=ORIENTED_EDGE('',*,*,#3825,.T.);
#5250=ORIENTED_EDGE('',*,*,#3805,.F.);
#5251=ORIENTED_EDGE('',*,*,#3614,.F.);
#5252=ORIENTED_EDGE('',*,*,#3749,.T.);
#5253=ORIENTED_EDGE('',*,*,#3665,.T.);
#5254=ORIENTED_EDGE('',*,*,#3751,.F.);
#5255=ORIENTED_EDGE('',*,*,#3806,.F.);
#5256=ORIENTED_EDGE('',*,*,#3825,.F.);
#5257=ORIENTED_EDGE('',*,*,#3660,.T.);
#5258=ORIENTED_EDGE('',*,*,#3826,.T.);
#5259=ORIENTED_EDGE('',*,*,#3803,.F.);
#5260=ORIENTED_EDGE('',*,*,#3617,.F.);
#5261=ORIENTED_EDGE('',*,*,#3752,.T.);
#5262=ORIENTED_EDGE('',*,*,#3662,.T.);
#5263=ORIENTED_EDGE('',*,*,#3754,.F.);
#5264=ORIENTED_EDGE('',*,*,#3804,.F.);
#5265=ORIENTED_EDGE('',*,*,#3826,.F.);
#5266=ORIENTED_EDGE('',*,*,#3657,.T.);
#5267=ORIENTED_EDGE('',*,*,#3827,.T.);
#5268=ORIENTED_EDGE('',*,*,#3801,.F.);
#5269=ORIENTED_EDGE('',*,*,#3620,.F.);
#5270=ORIENTED_EDGE('',*,*,#3755,.T.);
#5271=ORIENTED_EDGE('',*,*,#3659,.T.);
#5272=ORIENTED_EDGE('',*,*,#3757,.F.);
#5273=ORIENTED_EDGE('',*,*,#3802,.F.);
#5274=ORIENTED_EDGE('',*,*,#3827,.F.);
#5275=ORIENTED_EDGE('',*,*,#3654,.T.);
#5276=ORIENTED_EDGE('',*,*,#3828,.T.);
#5277=ORIENTED_EDGE('',*,*,#3799,.F.);
#5278=ORIENTED_EDGE('',*,*,#3623,.F.);
#5279=ORIENTED_EDGE('',*,*,#3758,.T.);
#5280=ORIENTED_EDGE('',*,*,#3656,.T.);
#5281=ORIENTED_EDGE('',*,*,#3760,.F.);
#5282=ORIENTED_EDGE('',*,*,#3800,.F.);
#5283=ORIENTED_EDGE('',*,*,#3828,.F.);
#5284=ORIENTED_EDGE('',*,*,#3651,.T.);
#5285=ORIENTED_EDGE('',*,*,#3829,.T.);
#5286=ORIENTED_EDGE('',*,*,#3797,.F.);
#5287=ORIENTED_EDGE('',*,*,#3626,.F.);
#5288=ORIENTED_EDGE('',*,*,#3761,.T.);
#5289=ORIENTED_EDGE('',*,*,#3653,.T.);
#5290=ORIENTED_EDGE('',*,*,#3763,.F.);
#5291=ORIENTED_EDGE('',*,*,#3798,.F.);
#5292=ORIENTED_EDGE('',*,*,#3829,.F.);
#5293=ORIENTED_EDGE('',*,*,#3648,.T.);
#5294=ORIENTED_EDGE('',*,*,#3830,.T.);
#5295=ORIENTED_EDGE('',*,*,#3795,.F.);
#5296=ORIENTED_EDGE('',*,*,#3629,.F.);
#5297=ORIENTED_EDGE('',*,*,#3764,.T.);
#5298=ORIENTED_EDGE('',*,*,#3650,.T.);
#5299=ORIENTED_EDGE('',*,*,#3766,.F.);
#5300=ORIENTED_EDGE('',*,*,#3796,.F.);
#5301=ORIENTED_EDGE('',*,*,#3830,.F.);
#5302=ORIENTED_EDGE('',*,*,#3645,.T.);
#5303=ORIENTED_EDGE('',*,*,#3831,.T.);
#5304=ORIENTED_EDGE('',*,*,#3793,.F.);
#5305=ORIENTED_EDGE('',*,*,#3632,.F.);
#5306=ORIENTED_EDGE('',*,*,#3767,.T.);
#5307=ORIENTED_EDGE('',*,*,#3647,.T.);
#5308=ORIENTED_EDGE('',*,*,#3769,.F.);
#5309=ORIENTED_EDGE('',*,*,#3794,.F.);
#5310=ORIENTED_EDGE('',*,*,#3831,.F.);
#5311=ORIENTED_EDGE('',*,*,#3706,.T.);
#5312=ORIENTED_EDGE('',*,*,#3644,.F.);
#6589=CYLINDRICAL_SURFACE('',#7284,2.05);
#6590=CYLINDRICAL_SURFACE('',#7287,2.05);
#6591=CYLINDRICAL_SURFACE('',#7292,6.025);
#6592=CYLINDRICAL_SURFACE('',#7322,10.);
#6593=CYLINDRICAL_SURFACE('',#7365,10.5);
#6700=ADVANCED_FACE('',(#1049),#680,.T.);
#6701=ADVANCED_FACE('',(#1050),#681,.F.);
#6702=ADVANCED_FACE('',(#1051),#6589,.F.);
#6703=ADVANCED_FACE('',(#1052),#682,.F.);
#6704=ADVANCED_FACE('',(#1053),#6590,.F.);
#6705=ADVANCED_FACE('',(#1054),#683,.F.);
#6706=ADVANCED_FACE('',(#1055,#798),#6591,.F.);
#6707=ADVANCED_FACE('',(#1056,#799),#886,.T.);
#6708=ADVANCED_FACE('',(#1057),#684,.F.);
#6709=ADVANCED_FACE('',(#1058,#800),#887,.T.);
#6710=ADVANCED_FACE('',(#1059),#685,.T.);
#6711=ADVANCED_FACE('',(#1060,#801),#6592,.T.);
#6712=ADVANCED_FACE('',(#1061),#686,.T.);
#6713=ADVANCED_FACE('',(#1062),#687,.T.);
#6714=ADVANCED_FACE('',(#1063),#688,.T.);
#6715=ADVANCED_FACE('',(#1064),#689,.T.);
#6716=ADVANCED_FACE('',(#1065),#690,.T.);
#6717=ADVANCED_FACE('',(#1066),#691,.T.);
#6718=ADVANCED_FACE('',(#1067),#692,.T.);
#6719=ADVANCED_FACE('',(#1068),#693,.T.);
#6720=ADVANCED_FACE('',(#1069),#694,.T.);
#6721=ADVANCED_FACE('',(#1070),#695,.T.);
#6722=ADVANCED_FACE('',(#1071),#696,.T.);
#6723=ADVANCED_FACE('',(#1072),#697,.T.);
#6724=ADVANCED_FACE('',(#1073),#698,.T.);
#6725=ADVANCED_FACE('',(#1074),#699,.T.);
#6726=ADVANCED_FACE('',(#1075),#700,.T.);
#6727=ADVANCED_FACE('',(#1076),#701,.T.);
#6728=ADVANCED_FACE('',(#1077),#702,.T.);
#6729=ADVANCED_FACE('',(#1078),#703,.T.);
#6730=ADVANCED_FACE('',(#1079),#704,.T.);
#6731=ADVANCED_FACE('',(#1080),#705,.T.);
#6732=ADVANCED_FACE('',(#1081),#6593,.T.);
#6733=ADVANCED_FACE('',(#1082),#706,.T.);
#6734=ADVANCED_FACE('',(#1083),#93,.F.);
#6735=ADVANCED_FACE('',(#1084),#94,.F.);
#6736=ADVANCED_FACE('',(#1085),#95,.F.);
#6737=ADVANCED_FACE('',(#1086),#96,.F.);
#6738=ADVANCED_FACE('',(#1087),#97,.F.);
#6739=ADVANCED_FACE('',(#1088),#98,.F.);
#6740=ADVANCED_FACE('',(#1089),#99,.F.);
#6741=ADVANCED_FACE('',(#1090),#100,.F.);
#6742=ADVANCED_FACE('',(#1091),#101,.F.);
#6743=ADVANCED_FACE('',(#1092),#102,.F.);
#6744=ADVANCED_FACE('',(#1093),#103,.F.);
#6745=ADVANCED_FACE('',(#1094),#104,.F.);
#6746=ADVANCED_FACE('',(#1095),#105,.F.);
#6747=ADVANCED_FACE('',(#1096),#106,.F.);
#6748=ADVANCED_FACE('',(#1097),#107,.F.);
#6749=ADVANCED_FACE('',(#1098),#108,.F.);
#6750=ADVANCED_FACE('',(#1099),#109,.F.);
#6751=ADVANCED_FACE('',(#1100),#110,.F.);
#6752=ADVANCED_FACE('',(#1101),#111,.F.);
#6753=ADVANCED_FACE('',(#1102),#112,.F.);
#6754=ADVANCED_FACE('',(#1103),#113,.F.);
#6755=ADVANCED_FACE('',(#1104),#888,.T.);
#6756=ADVANCED_FACE('',(#1105),#707,.T.);
#6757=ADVANCED_FACE('',(#1106),#114,.F.);
#6758=ADVANCED_FACE('',(#1107),#889,.T.);
#6759=ADVANCED_FACE('',(#1108),#115,.F.);
#6760=ADVANCED_FACE('',(#1109),#890,.T.);
#6761=ADVANCED_FACE('',(#1110),#116,.F.);
#6762=ADVANCED_FACE('',(#1111),#891,.T.);
#6763=ADVANCED_FACE('',(#1112),#117,.F.);
#6764=ADVANCED_FACE('',(#1113),#892,.T.);
#6765=ADVANCED_FACE('',(#1114),#118,.F.);
#6766=ADVANCED_FACE('',(#1115),#893,.T.);
#6767=ADVANCED_FACE('',(#1116),#119,.F.);
#6768=ADVANCED_FACE('',(#1117),#894,.T.);
#6769=ADVANCED_FACE('',(#1118),#120,.F.);
#6770=ADVANCED_FACE('',(#1119),#895,.T.);
#6771=ADVANCED_FACE('',(#1120),#121,.F.);
#6772=ADVANCED_FACE('',(#1121),#896,.T.);
#6773=ADVANCED_FACE('',(#1122),#122,.F.);
#6774=ADVANCED_FACE('',(#1123),#897,.T.);
#6775=ADVANCED_FACE('',(#1124),#123,.F.);
#6776=ADVANCED_FACE('',(#1125),#898,.T.);
#6777=ADVANCED_FACE('',(#1126),#124,.F.);
#6778=ADVANCED_FACE('',(#1127),#899,.T.);
#6779=ADVANCED_FACE('',(#1128),#125,.F.);
#6780=ADVANCED_FACE('',(#1129),#900,.T.);
#6781=ADVANCED_FACE('',(#1130),#126,.F.);
#6782=ADVANCED_FACE('',(#1131),#901,.T.);
#6783=ADVANCED_FACE('',(#1132),#127,.F.);
#6784=ADVANCED_FACE('',(#1133),#902,.T.);
#6785=ADVANCED_FACE('',(#1134),#128,.F.);
#6786=ADVANCED_FACE('',(#1135),#903,.T.);
#6787=ADVANCED_FACE('',(#1136),#129,.F.);
#6788=ADVANCED_FACE('',(#1137),#904,.T.);
#6789=ADVANCED_FACE('',(#1138),#130,.F.);
#6790=ADVANCED_FACE('',(#1139),#905,.T.);
#6791=ADVANCED_FACE('',(#1140),#131,.F.);
#6792=ADVANCED_FACE('',(#1141),#906,.T.);
#6793=ADVANCED_FACE('',(#1142),#132,.F.);
#6794=ADVANCED_FACE('',(#1143),#907,.T.);
#6795=ADVANCED_FACE('',(#1144,#802),#908,.T.);
#7026=CLOSED_SHELL('',(#6700,#6701,#6702,#6703,#6704,#6705,#6706,#6707,
#6708,#6709,#6710,#6711,#6712,#6713,#6714,#6715,#6716,#6717,#6718,#6719,
#6720,#6721,#6722,#6723,#6724,#6725,#6726,#6727,#6728,#6729,#6730,#6731,
#6732,#6733,#6734,#6735,#6736,#6737,#6738,#6739,#6740,#6741,#6742,#6743,
#6744,#6745,#6746,#6747,#6748,#6749,#6750,#6751,#6752,#6753,#6754,#6755,
#6756,#6757,#6758,#6759,#6760,#6761,#6762,#6763,#6764,#6765,#6766,#6767,
#6768,#6769,#6770,#6771,#6772,#6773,#6774,#6775,#6776,#6777,#6778,#6779,
#6780,#6781,#6782,#6783,#6784,#6785,#6786,#6787,#6788,#6789,#6790,#6791,
#6792,#6793,#6794,#6795));
#7279=AXIS2_PLACEMENT_3D('',#9764,#8180,#8181);
#7280=AXIS2_PLACEMENT_3D('',#9765,#8182,#8183);
#7281=AXIS2_PLACEMENT_3D('',#9777,#8185,#8186);
#7282=AXIS2_PLACEMENT_3D('',#9782,#8187,#8188);
#7283=AXIS2_PLACEMENT_3D('',#9827,#8190,#8191);
#7284=AXIS2_PLACEMENT_3D('',#9828,#8192,#8193);
#7285=AXIS2_PLACEMENT_3D('',#9871,#8195,#8196);
#7286=AXIS2_PLACEMENT_3D('',#9894,#8198,#8199);
#7287=AXIS2_PLACEMENT_3D('',#9914,#8200,#8201);
#7288=AXIS2_PLACEMENT_3D('',#9954,#8203,#8204);
#7289=AXIS2_PLACEMENT_3D('',#9956,#8205,#8206);
#7290=AXIS2_PLACEMENT_3D('',#9960,#8208,#8209);
#7291=AXIS2_PLACEMENT_3D('',#9961,#8210,#8211);
#7292=AXIS2_PLACEMENT_3D('',#9962,#8212,#8213);
#7293=AXIS2_PLACEMENT_3D('',#9965,#8214,#8215);
#7294=AXIS2_PLACEMENT_3D('',#9966,#8216,#8217);
#7295=AXIS2_PLACEMENT_3D('',#9969,#8220,#8221);
#7296=AXIS2_PLACEMENT_3D('',#9972,#8222,#8223);
#7297=AXIS2_PLACEMENT_3D('',#10046,#8224,#8225);
#7298=AXIS2_PLACEMENT_3D('',#10120,#8226,#8227);
#7299=AXIS2_PLACEMENT_3D('',#10194,#8228,#8229);
#7300=AXIS2_PLACEMENT_3D('',#10268,#8230,#8231);
#7301=AXIS2_PLACEMENT_3D('',#10342,#8232,#8233);
#7302=AXIS2_PLACEMENT_3D('',#10416,#8234,#8235);
#7303=AXIS2_PLACEMENT_3D('',#10490,#8236,#8237);
#7304=AXIS2_PLACEMENT_3D('',#10564,#8238,#8239);
#7305=AXIS2_PLACEMENT_3D('',#10709,#8240,#8241);
#7306=AXIS2_PLACEMENT_3D('',#10783,#8242,#8243);
#7307=AXIS2_PLACEMENT_3D('',#10857,#8244,#8245);
#7308=AXIS2_PLACEMENT_3D('',#10931,#8246,#8247);
#7309=AXIS2_PLACEMENT_3D('',#11005,#8248,#8249);
#7310=AXIS2_PLACEMENT_3D('',#11079,#8250,#8251);
#7311=AXIS2_PLACEMENT_3D('',#11153,#8252,#8253);
#7312=AXIS2_PLACEMENT_3D('',#11227,#8254,#8255);
#7313=AXIS2_PLACEMENT_3D('',#11301,#8256,#8257);
#7314=AXIS2_PLACEMENT_3D('',#11375,#8258,#8259);
#7315=AXIS2_PLACEMENT_3D('',#11447,#8260,#8261);
#7316=AXIS2_PLACEMENT_3D('',#11450,#8263,#8264);
#7317=AXIS2_PLACEMENT_3D('',#11451,#8265,#8266);
#7318=AXIS2_PLACEMENT_3D('',#11453,#8267,#8268);
#7319=AXIS2_PLACEMENT_3D('',#11454,#8269,#8270);
#7320=AXIS2_PLACEMENT_3D('',#11458,#8272,#8273);
#7321=AXIS2_PLACEMENT_3D('',#11459,#8274,#8275);
#7322=AXIS2_PLACEMENT_3D('',#11460,#8276,#8277);
#7323=AXIS2_PLACEMENT_3D('',#11464,#8280,#8281);
#7324=AXIS2_PLACEMENT_3D('',#11465,#8282,#8283);
#7325=AXIS2_PLACEMENT_3D('',#11495,#8284,#8285);
#7326=AXIS2_PLACEMENT_3D('',#11496,#8286,#8287);
#7327=AXIS2_PLACEMENT_3D('',#11526,#8288,#8289);
#7328=AXIS2_PLACEMENT_3D('',#11527,#8290,#8291);
#7329=AXIS2_PLACEMENT_3D('',#11557,#8292,#8293);
#7330=AXIS2_PLACEMENT_3D('',#11558,#8294,#8295);
#7331=AXIS2_PLACEMENT_3D('',#11588,#8296,#8297);
#7332=AXIS2_PLACEMENT_3D('',#11589,#8298,#8299);
#7333=AXIS2_PLACEMENT_3D('',#11619,#8300,#8301);
#7334=AXIS2_PLACEMENT_3D('',#11620,#8302,#8303);
#7335=AXIS2_PLACEMENT_3D('',#11650,#8304,#8305);
#7336=AXIS2_PLACEMENT_3D('',#11651,#8306,#8307);
#7337=AXIS2_PLACEMENT_3D('',#11681,#8308,#8309);
#7338=AXIS2_PLACEMENT_3D('',#11682,#8310,#8311);
#7339=AXIS2_PLACEMENT_3D('',#11712,#8312,#8313);
#7340=AXIS2_PLACEMENT_3D('',#11713,#8314,#8315);
#7341=AXIS2_PLACEMENT_3D('',#11743,#8316,#8317);
#7342=AXIS2_PLACEMENT_3D('',#11744,#8318,#8319);
#7343=AXIS2_PLACEMENT_3D('',#11774,#8320,#8321);
#7344=AXIS2_PLACEMENT_3D('',#11775,#8322,#8323);
#7345=AXIS2_PLACEMENT_3D('',#11805,#8324,#8325);
#7346=AXIS2_PLACEMENT_3D('',#11806,#8326,#8327);
#7347=AXIS2_PLACEMENT_3D('',#11836,#8328,#8329);
#7348=AXIS2_PLACEMENT_3D('',#11837,#8330,#8331);
#7349=AXIS2_PLACEMENT_3D('',#11867,#8332,#8333);
#7350=AXIS2_PLACEMENT_3D('',#11868,#8334,#8335);
#7351=AXIS2_PLACEMENT_3D('',#11898,#8336,#8337);
#7352=AXIS2_PLACEMENT_3D('',#11899,#8338,#8339);
#7353=AXIS2_PLACEMENT_3D('',#11929,#8340,#8341);
#7354=AXIS2_PLACEMENT_3D('',#11930,#8342,#8343);
#7355=AXIS2_PLACEMENT_3D('',#11960,#8344,#8345);
#7356=AXIS2_PLACEMENT_3D('',#11961,#8346,#8347);
#7357=AXIS2_PLACEMENT_3D('',#11991,#8348,#8349);
#7358=AXIS2_PLACEMENT_3D('',#11992,#8350,#8351);
#7359=AXIS2_PLACEMENT_3D('',#12022,#8352,#8353);
#7360=AXIS2_PLACEMENT_3D('',#12023,#8354,#8355);
#7361=AXIS2_PLACEMENT_3D('',#12053,#8356,#8357);
#7362=AXIS2_PLACEMENT_3D('',#12054,#8358,#8359);
#7363=AXIS2_PLACEMENT_3D('',#12056,#8360,#8361);
#7364=AXIS2_PLACEMENT_3D('',#12059,#8363,#8364);
#7365=AXIS2_PLACEMENT_3D('',#12060,#8365,#8366);
#7366=AXIS2_PLACEMENT_3D('',#12063,#8368,#8369);
#7367=AXIS2_PLACEMENT_3D('',#12064,#8370,#8371);
#7368=AXIS2_PLACEMENT_3D('',#12094,#8372,#8373);
#7369=AXIS2_PLACEMENT_3D('',#13428,#8394,#8395);
#7370=AXIS2_PLACEMENT_3D('',#13429,#8396,#8397);
#7371=AXIS2_PLACEMENT_3D('',#13430,#8398,#8399);
#7372=AXIS2_PLACEMENT_3D('',#13433,#8401,#8402);
#7373=AXIS2_PLACEMENT_3D('',#13441,#8403,#8404);
#7374=AXIS2_PLACEMENT_3D('',#13471,#8405,#8406);
#7375=AXIS2_PLACEMENT_3D('',#13513,#8407,#8408);
#7376=AXIS2_PLACEMENT_3D('',#13555,#8409,#8410);
#7377=AXIS2_PLACEMENT_3D('',#13597,#8411,#8412);
#7378=AXIS2_PLACEMENT_3D('',#13627,#8413,#8414);
#7379=AXIS2_PLACEMENT_3D('',#13657,#8415,#8416);
#7380=AXIS2_PLACEMENT_3D('',#13699,#8417,#8418);
#7381=AXIS2_PLACEMENT_3D('',#13741,#8419,#8420);
#7382=AXIS2_PLACEMENT_3D('',#13771,#8421,#8422);
#7383=AXIS2_PLACEMENT_3D('',#13801,#8423,#8424);
#7384=AXIS2_PLACEMENT_3D('',#13843,#8425,#8426);
#7385=AXIS2_PLACEMENT_3D('',#13885,#8427,#8428);
#7386=AXIS2_PLACEMENT_3D('',#13927,#8429,#8430);
#7387=AXIS2_PLACEMENT_3D('',#13957,#8431,#8432);
#7388=AXIS2_PLACEMENT_3D('',#13987,#8433,#8434);
#7389=AXIS2_PLACEMENT_3D('',#14029,#8435,#8436);
#7390=AXIS2_PLACEMENT_3D('',#14071,#8437,#8438);
#7391=AXIS2_PLACEMENT_3D('',#14113,#8439,#8440);
#7392=AXIS2_PLACEMENT_3D('',#14230,#8441,#8442);
#7393=AXIS2_PLACEMENT_3D('',#14347,#8443,#8444);
#7394=AXIS2_PLACEMENT_3D('',#14402,#8445,#8446);
#7395=AXIS2_PLACEMENT_3D('',#14457,#8447,#8448);
#7396=AXIS2_PLACEMENT_3D('',#14574,#8449,#8450);
#7397=AXIS2_PLACEMENT_3D('',#14691,#8451,#8452);
#7398=AXIS2_PLACEMENT_3D('',#14808,#8453,#8454);
#7399=AXIS2_PLACEMENT_3D('',#14863,#8455,#8456);
#7400=AXIS2_PLACEMENT_3D('',#14918,#8457,#8458);
#7401=AXIS2_PLACEMENT_3D('',#15035,#8459,#8460);
#7402=AXIS2_PLACEMENT_3D('',#15152,#8461,#8462);
#7403=AXIS2_PLACEMENT_3D('',#15269,#8463,#8464);
#7404=AXIS2_PLACEMENT_3D('',#15324,#8465,#8466);
#7405=AXIS2_PLACEMENT_3D('',#15379,#8467,#8468);
#7406=AXIS2_PLACEMENT_3D('',#15496,#8469,#8470);
#7407=AXIS2_PLACEMENT_3D('',#15613,#8471,#8472);
#7408=AXIS2_PLACEMENT_3D('',#15730,#8473,#8474);
#7409=AXIS2_PLACEMENT_3D('',#15785,#8475,#8476);
#7410=AXIS2_PLACEMENT_3D('',#15840,#8477,#8478);
#7411=AXIS2_PLACEMENT_3D('',#15841,#8479,#8480);
#8180=DIRECTION('axis',(0.,0.,1.));
#8181=DIRECTION('refdir',(1.,0.,0.));
#8182=DIRECTION('center_axis',(1.,0.,0.));
#8183=DIRECTION('ref_axis',(0.,1.,0.));
#8184=DIRECTION('',(-0.739012155113086,0.673692091830617,8.2503486387125E-17));
#8185=DIRECTION('center_axis',(1.,0.,0.));
#8186=DIRECTION('ref_axis',(0.,0.,-1.));
#8187=DIRECTION('center_axis',(0.,-1.,0.));
#8188=DIRECTION('ref_axis',(0.,0.,-1.));
#8189=DIRECTION('',(-8.65956056235493E-17,0.707106781186548,-0.707106781186547));
#8190=DIRECTION('center_axis',(0.,1.,0.));
#8191=DIRECTION('ref_axis',(0.,0.,-1.));
#8192=DIRECTION('center_axis',(0.,1.,0.));
#8193=DIRECTION('ref_axis',(0.,0.,-1.));
#8194=DIRECTION('',(0.,1.,0.));
#8195=DIRECTION('center_axis',(0.,0.,1.));
#8196=DIRECTION('ref_axis',(1.,0.,0.));
#8197=DIRECTION('',(0.707106781186547,-8.65956056235493E-17,-0.707106781186548));
#8198=DIRECTION('center_axis',(0.,0.,-1.));
#8199=DIRECTION('ref_axis',(1.,0.,0.));
#8200=DIRECTION('center_axis',(0.,0.,-1.));
#8201=DIRECTION('ref_axis',(1.,0.,0.));
#8202=DIRECTION('',(0.,0.,-1.));
#8203=DIRECTION('center_axis',(-1.,0.,0.));
#8204=DIRECTION('ref_axis',(0.,-1.,0.));
#8205=DIRECTION('center_axis',(-1.,0.,0.));
#8206=DIRECTION('ref_axis',(0.,-1.,0.));
#8207=DIRECTION('',(0.707106781186547,-0.707106781186547,8.65956056235493E-17));
#8208=DIRECTION('center_axis',(1.,0.,0.));
#8209=DIRECTION('ref_axis',(0.,-1.,0.));
#8210=DIRECTION('center_axis',(1.,0.,0.));
#8211=DIRECTION('ref_axis',(0.,-1.,0.));
#8212=DIRECTION('center_axis',(1.,0.,0.));
#8213=DIRECTION('ref_axis',(0.,1.,0.));
#8214=DIRECTION('center_axis',(-1.,0.,0.));
#8215=DIRECTION('ref_axis',(0.,-1.,0.));
#8216=DIRECTION('center_axis',(-1.,0.,0.));
#8217=DIRECTION('ref_axis',(0.,-1.,0.));
#8218=DIRECTION('',(-1.,0.,0.));
#8219=DIRECTION('',(-1.,0.,0.));
#8220=DIRECTION('center_axis',(-1.,0.,0.));
#8221=DIRECTION('ref_axis',(0.,0.,1.));
#8222=DIRECTION('center_axis',(1.,0.,0.));
#8223=DIRECTION('ref_axis',(0.,0.,-1.));
#8224=DIRECTION('center_axis',(1.,0.,0.));
#8225=DIRECTION('ref_axis',(0.,0.,-1.));
#8226=DIRECTION('center_axis',(1.,0.,0.));
#8227=DIRECTION('ref_axis',(0.,0.,-1.));
#8228=DIRECTION('center_axis',(1.,0.,0.));
#8229=DIRECTION('ref_axis',(0.,0.,-1.));
#8230=DIRECTION('center_axis',(1.,0.,0.));
#8231=DIRECTION('ref_axis',(0.,0.,-1.));
#8232=DIRECTION('center_axis',(1.,0.,0.));
#8233=DIRECTION('ref_axis',(0.,0.,-1.));
#8234=DIRECTION('center_axis',(1.,0.,0.));
#8235=DIRECTION('ref_axis',(0.,0.,-1.));
#8236=DIRECTION('center_axis',(1.,0.,0.));
#8237=DIRECTION('ref_axis',(0.,0.,-1.));
#8238=DIRECTION('center_axis',(1.,0.,0.));
#8239=DIRECTION('ref_axis',(0.,0.,-1.));
#8240=DIRECTION('center_axis',(1.,0.,0.));
#8241=DIRECTION('ref_axis',(0.,0.,-1.));
#8242=DIRECTION('center_axis',(1.,0.,0.));
#8243=DIRECTION('ref_axis',(0.,0.,-1.));
#8244=DIRECTION('center_axis',(1.,0.,0.));
#8245=DIRECTION('ref_axis',(0.,0.,-1.));
#8246=DIRECTION('center_axis',(1.,0.,0.));
#8247=DIRECTION('ref_axis',(0.,0.,-1.));
#8248=DIRECTION('center_axis',(1.,0.,0.));
#8249=DIRECTION('ref_axis',(0.,0.,-1.));
#8250=DIRECTION('center_axis',(1.,0.,0.));
#8251=DIRECTION('ref_axis',(0.,0.,-1.));
#8252=DIRECTION('center_axis',(1.,0.,0.));
#8253=DIRECTION('ref_axis',(0.,0.,-1.));
#8254=DIRECTION('center_axis',(1.,0.,0.));
#8255=DIRECTION('ref_axis',(0.,0.,-1.));
#8256=DIRECTION('center_axis',(1.,0.,0.));
#8257=DIRECTION('ref_axis',(0.,0.,-1.));
#8258=DIRECTION('center_axis',(1.,0.,0.));
#8259=DIRECTION('ref_axis',(0.,0.,-1.));
#8260=DIRECTION('center_axis',(1.,0.,0.));
#8261=DIRECTION('ref_axis',(0.,-1.,0.));
#8262=DIRECTION('',(0.707106781186546,0.707106781186549,-8.65956056235495E-17));
#8263=DIRECTION('center_axis',(1.,0.,0.));
#8264=DIRECTION('ref_axis',(0.,-1.,0.));
#8265=DIRECTION('center_axis',(1.,0.,0.));
#8266=DIRECTION('ref_axis',(0.,0.,-1.));
#8267=DIRECTION('center_axis',(-1.,0.,0.));
#8268=DIRECTION('ref_axis',(0.,-1.,0.));
#8269=DIRECTION('center_axis',(-1.,0.,0.));
#8270=DIRECTION('ref_axis',(0.,-1.,0.));
#8271=DIRECTION('',(-0.707106781186546,0.707106781186549,8.65956056235495E-17));
#8272=DIRECTION('center_axis',(1.,0.,0.));
#8273=DIRECTION('ref_axis',(0.,-1.,0.));
#8274=DIRECTION('center_axis',(1.,0.,0.));
#8275=DIRECTION('ref_axis',(0.,-1.,0.));
#8276=DIRECTION('center_axis',(1.,0.,0.));
#8277=DIRECTION('ref_axis',(0.,1.,0.));
#8278=DIRECTION('',(-1.,0.,0.));
#8279=DIRECTION('',(-1.,0.,0.));
#8280=DIRECTION('center_axis',(1.,0.,0.));
#8281=DIRECTION('ref_axis',(0.,0.,-1.));
#8282=DIRECTION('center_axis',(-1.,0.,0.));
#8283=DIRECTION('ref_axis',(0.,1.,0.));
#8284=DIRECTION('center_axis',(1.,-9.71851396181453E-17,-2.16484527094502E-17));
#8285=DIRECTION('ref_axis',(0.,1.,0.));
#8286=DIRECTION('center_axis',(-1.,0.,0.));
#8287=DIRECTION('ref_axis',(0.,1.,0.));
#8288=DIRECTION('center_axis',(1.,-8.57388205317489E-17,-5.0620761759739E-17));
#8289=DIRECTION('ref_axis',(0.,1.,0.));
#8290=DIRECTION('center_axis',(-1.,0.,0.));
#8291=DIRECTION('ref_axis',(0.,1.,0.));
#8292=DIRECTION('center_axis',(1.,-6.58997883142157E-17,-7.46379579533984E-17));
#8293=DIRECTION('ref_axis',(0.,1.,0.));
#8294=DIRECTION('center_axis',(-1.,0.,0.));
#8295=DIRECTION('ref_axis',(0.,1.,0.));
#8296=DIRECTION('center_axis',(1.,-3.96100256656632E-17,-9.13490707893474E-17));
#8297=DIRECTION('ref_axis',(0.,1.,0.));
#8298=DIRECTION('center_axis',(-1.,0.,0.));
#8299=DIRECTION('ref_axis',(0.,1.,0.));
#8300=DIRECTION('center_axis',(1.,-9.44295772567882E-18,-9.91183001100339E-17));
#8301=DIRECTION('ref_axis',(0.,1.,0.));
#8302=DIRECTION('center_axis',(-1.,0.,0.));
#8303=DIRECTION('ref_axis',(0.,1.,0.));
#8304=DIRECTION('center_axis',(1.,2.16484527094502E-17,-9.71851396181453E-17));
#8305=DIRECTION('ref_axis',(0.,1.,0.));
#8306=DIRECTION('center_axis',(-1.,0.,0.));
#8307=DIRECTION('ref_axis',(0.,1.,0.));
#8308=DIRECTION('center_axis',(1.,5.0620761759739E-17,-8.57388205317489E-17));
#8309=DIRECTION('ref_axis',(0.,1.,0.));
#8310=DIRECTION('center_axis',(-1.,0.,0.));
#8311=DIRECTION('ref_axis',(0.,1.,0.));
#8312=DIRECTION('center_axis',(1.,7.46379579533984E-17,-6.58997883142157E-17));
#8313=DIRECTION('ref_axis',(0.,1.,0.));
#8314=DIRECTION('center_axis',(-1.,0.,0.));
#8315=DIRECTION('ref_axis',(0.,1.,0.));
#8316=DIRECTION('center_axis',(1.,9.13490707893474E-17,-3.96100256656632E-17));
#8317=DIRECTION('ref_axis',(0.,1.,0.));
#8318=DIRECTION('center_axis',(-1.,0.,0.));
#8319=DIRECTION('ref_axis',(0.,-0.997421223023649,0.0717697977007645));
#8320=DIRECTION('center_axis',(1.,9.91183001100339E-17,-9.44295772567882E-18));
#8321=DIRECTION('ref_axis',(0.,1.,0.));
#8322=DIRECTION('center_axis',(-1.,0.,0.));
#8323=DIRECTION('ref_axis',(0.,1.,0.));
#8324=DIRECTION('center_axis',(1.,9.71851396181453E-17,2.16484527094502E-17));
#8325=DIRECTION('ref_axis',(0.,1.,0.));
#8326=DIRECTION('center_axis',(-1.,0.,0.));
#8327=DIRECTION('ref_axis',(0.,1.,0.));
#8328=DIRECTION('center_axis',(1.,8.57388205317489E-17,5.0620761759739E-17));
#8329=DIRECTION('ref_axis',(0.,1.,0.));
#8330=DIRECTION('center_axis',(-1.,0.,0.));
#8331=DIRECTION('ref_axis',(0.,1.,0.));
#8332=DIRECTION('center_axis',(1.,6.58997883142157E-17,7.46379579533984E-17));
#8333=DIRECTION('ref_axis',(0.,1.,0.));
#8334=DIRECTION('center_axis',(-1.,0.,0.));
#8335=DIRECTION('ref_axis',(0.,1.,0.));
#8336=DIRECTION('center_axis',(1.,3.96100256656632E-17,9.13490707893474E-17));
#8337=DIRECTION('ref_axis',(0.,1.,0.));
#8338=DIRECTION('center_axis',(-1.,0.,0.));
#8339=DIRECTION('ref_axis',(0.,1.,0.));
#8340=DIRECTION('center_axis',(1.,9.44295772567883E-18,9.91183001100339E-17));
#8341=DIRECTION('ref_axis',(0.,1.,0.));
#8342=DIRECTION('center_axis',(-1.,0.,0.));
#8343=DIRECTION('ref_axis',(0.,1.,0.));
#8344=DIRECTION('center_axis',(1.,-2.16484527094502E-17,9.71851396181453E-17));
#8345=DIRECTION('ref_axis',(0.,1.,0.));
#8346=DIRECTION('center_axis',(-1.,0.,0.));
#8347=DIRECTION('ref_axis',(0.,1.,0.));
#8348=DIRECTION('center_axis',(1.,-5.0620761759739E-17,8.57388205317489E-17));
#8349=DIRECTION('ref_axis',(0.,1.,0.));
#8350=DIRECTION('center_axis',(-1.,0.,0.));
#8351=DIRECTION('ref_axis',(0.,1.,0.));
#8352=DIRECTION('center_axis',(1.,-7.46379579533983E-17,6.58997883142157E-17));
#8353=DIRECTION('ref_axis',(0.,1.,0.));
#8354=DIRECTION('center_axis',(-1.,0.,0.));
#8355=DIRECTION('ref_axis',(0.,1.,0.));
#8356=DIRECTION('center_axis',(1.,-9.13490707893474E-17,3.96100256656632E-17));
#8357=DIRECTION('ref_axis',(0.,1.,0.));
#8358=DIRECTION('center_axis',(-1.,0.,0.));
#8359=DIRECTION('ref_axis',(0.,1.,0.));
#8360=DIRECTION('center_axis',(-1.,0.,0.));
#8361=DIRECTION('ref_axis',(0.,1.,0.));
#8362=DIRECTION('',(0.68394112888133,0.729537204140085,8.93425401909064E-17));
#8363=DIRECTION('center_axis',(1.,0.,0.));
#8364=DIRECTION('ref_axis',(0.,0.,-1.));
#8365=DIRECTION('center_axis',(1.,0.,0.));
#8366=DIRECTION('ref_axis',(0.,1.,0.));
#8367=DIRECTION('',(1.,0.,0.));
#8368=DIRECTION('center_axis',(1.,0.,0.));
#8369=DIRECTION('ref_axis',(0.,1.,0.));
#8370=DIRECTION('center_axis',(-1.,0.,0.));
#8371=DIRECTION('ref_axis',(0.,1.,0.));
#8372=DIRECTION('center_axis',(1.,-9.91183001100339E-17,9.44295772567884E-18));
#8373=DIRECTION('ref_axis',(0.,1.,0.));
#8374=DIRECTION('',(0.657420344909251,0.731109352828835,0.182421501763368));
#8375=DIRECTION('',(0.657420344909251,0.751697658316477,-0.0524320568061806));
#8376=DIRECTION('',(0.657420344909251,0.698704559622551,-0.28215320033992));
#8377=DIRECTION('',(0.657420344909251,0.577317390471848,-0.484255222747444));
#8378=DIRECTION('',(0.657420344909251,0.399418372734979,-0.638954969947916));
#8379=DIRECTION('',(0.657420344909251,0.182421501763368,-0.731109352828835));
#8380=DIRECTION('',(0.657420344909251,-0.0524320568061806,-0.751697658316477));
#8381=DIRECTION('',(0.657420344909251,-0.282153200339919,-0.698704559622551));
#8382=DIRECTION('',(0.657420344909251,-0.484255222747444,-0.577317390471848));
#8383=DIRECTION('',(0.657420344909251,-0.638954969947916,-0.399418372734979));
#8384=DIRECTION('',(0.657420344909251,-0.731109352828835,-0.182421501763368));
#8385=DIRECTION('',(0.657420344909251,-0.751697658316477,0.0524320568061806));
#8386=DIRECTION('',(0.657420344909251,-0.698704559622551,0.282153200339919));
#8387=DIRECTION('',(0.657420344909251,-0.577317390471848,0.484255222747444));
#8388=DIRECTION('',(0.657420344909251,-0.399418372734979,0.638954969947916));
#8389=DIRECTION('',(0.657420344909251,-0.182421501763368,0.731109352828835));
#8390=DIRECTION('',(0.657420344909251,0.0524320568061804,0.751697658316477));
#8391=DIRECTION('',(0.657420344909251,0.282153200339919,0.698704559622551));
#8392=DIRECTION('',(0.657420344909251,0.484255222747444,0.577317390471848));
#8393=DIRECTION('',(0.657420344909251,0.638954969947916,0.399418372734979));
#8394=DIRECTION('center_axis',(1.,-9.91183001100339E-17,9.44295772567884E-18));
#8395=DIRECTION('ref_axis',(-2.16484527094502E-17,-0.309016994374948,-0.951056516295153));
#8396=DIRECTION('center_axis',(1.,-9.91183001100339E-17,9.44295772567884E-18));
#8397=DIRECTION('ref_axis',(0.,1.,0.));
#8398=DIRECTION('center_axis',(1.,0.,0.));
#8399=DIRECTION('ref_axis',(0.,1.,0.));
#8400=DIRECTION('',(-0.739012155113086,0.673692091830617,8.2503486387125E-17));
#8401=DIRECTION('center_axis',(1.,9.91183001100339E-17,-9.44295772567882E-18));
#8402=DIRECTION('ref_axis',(0.,1.,0.));
#8403=DIRECTION('center_axis',(1.,9.71851396181453E-17,2.16484527094502E-17));
#8404=DIRECTION('ref_axis',(0.,1.,0.));
#8405=DIRECTION('center_axis',(1.,8.57388205317489E-17,5.0620761759739E-17));
#8406=DIRECTION('ref_axis',(0.,1.,0.));
#8407=DIRECTION('center_axis',(1.,6.58997883142157E-17,7.46379579533984E-17));
#8408=DIRECTION('ref_axis',(0.,1.,0.));
#8409=DIRECTION('center_axis',(1.,3.96100256656632E-17,9.13490707893474E-17));
#8410=DIRECTION('ref_axis',(0.,1.,0.));
#8411=DIRECTION('center_axis',(1.,9.44295772567883E-18,9.91183001100339E-17));
#8412=DIRECTION('ref_axis',(0.,1.,0.));
#8413=DIRECTION('center_axis',(1.,-2.16484527094502E-17,9.71851396181453E-17));
#8414=DIRECTION('ref_axis',(0.,1.,0.));
#8415=DIRECTION('center_axis',(1.,-5.0620761759739E-17,8.57388205317489E-17));
#8416=DIRECTION('ref_axis',(0.,1.,0.));
#8417=DIRECTION('center_axis',(1.,-7.46379579533983E-17,6.58997883142157E-17));
#8418=DIRECTION('ref_axis',(0.,1.,0.));
#8419=DIRECTION('center_axis',(1.,-9.13490707893474E-17,3.96100256656632E-17));
#8420=DIRECTION('ref_axis',(0.,1.,0.));
#8421=DIRECTION('center_axis',(1.,-9.71851396181453E-17,-2.16484527094502E-17));
#8422=DIRECTION('ref_axis',(0.,1.,0.));
#8423=DIRECTION('center_axis',(1.,-8.57388205317489E-17,-5.0620761759739E-17));
#8424=DIRECTION('ref_axis',(0.,1.,0.));
#8425=DIRECTION('center_axis',(1.,-6.58997883142157E-17,-7.46379579533984E-17));
#8426=DIRECTION('ref_axis',(0.,1.,0.));
#8427=DIRECTION('center_axis',(1.,-3.96100256656632E-17,-9.13490707893474E-17));
#8428=DIRECTION('ref_axis',(0.,1.,0.));
#8429=DIRECTION('center_axis',(1.,-9.44295772567882E-18,-9.91183001100339E-17));
#8430=DIRECTION('ref_axis',(0.,1.,0.));
#8431=DIRECTION('center_axis',(1.,2.16484527094502E-17,-9.71851396181453E-17));
#8432=DIRECTION('ref_axis',(0.,1.,0.));
#8433=DIRECTION('center_axis',(1.,5.0620761759739E-17,-8.57388205317489E-17));
#8434=DIRECTION('ref_axis',(0.,1.,0.));
#8435=DIRECTION('center_axis',(1.,7.46379579533984E-17,-6.58997883142157E-17));
#8436=DIRECTION('ref_axis',(0.,1.,0.));
#8437=DIRECTION('center_axis',(1.,9.13490707893474E-17,-3.96100256656632E-17));
#8438=DIRECTION('ref_axis',(0.,1.,0.));
#8439=DIRECTION('center_axis',(1.,9.91183001100339E-17,-9.44295772567882E-18));
#8440=DIRECTION('ref_axis',(0.,1.,0.));
#8441=DIRECTION('center_axis',(1.,-9.13490707893474E-17,3.96100256656632E-17));
#8442=DIRECTION('ref_axis',(-2.16484527094502E-17,-0.587785252292473,-0.809016994374947));
#8443=DIRECTION('center_axis',(1.,-7.46379579533983E-17,6.58997883142157E-17));
#8444=DIRECTION('ref_axis',(-2.16484527094502E-17,-0.809016994374948,-0.587785252292473));
#8445=DIRECTION('center_axis',(1.,-5.0620761759739E-17,8.57388205317489E-17));
#8446=DIRECTION('ref_axis',(-2.16484527094502E-17,-0.951056516295154,-0.309016994374947));
#8447=DIRECTION('center_axis',(1.,-2.16484527094502E-17,9.71851396181453E-17));
#8448=DIRECTION('ref_axis',(-2.16484527094502E-17,-1.,1.83697019872103E-16));
#8449=DIRECTION('center_axis',(1.,9.44295772567883E-18,9.91183001100339E-17));
#8450=DIRECTION('ref_axis',(-2.16484527094502E-17,-0.951056516295153,0.309016994374948));
#8451=DIRECTION('center_axis',(1.,3.96100256656632E-17,9.13490707893474E-17));
#8452=DIRECTION('ref_axis',(-2.16484527094502E-17,-0.809016994374947,0.587785252292473));
#8453=DIRECTION('center_axis',(1.,6.58997883142157E-17,7.46379579533984E-17));
#8454=DIRECTION('ref_axis',(-2.16484527094502E-17,-0.587785252292473,0.809016994374947));
#8455=DIRECTION('center_axis',(1.,8.57388205317489E-17,5.0620761759739E-17));
#8456=DIRECTION('ref_axis',(-2.16484527094502E-17,-0.309016994374947,0.951056516295154));
#8457=DIRECTION('center_axis',(1.,9.71851396181453E-17,2.16484527094502E-17));
#8458=DIRECTION('ref_axis',(-2.16484527094502E-17,1.22464679914735E-16,
1.));
#8459=DIRECTION('center_axis',(1.,9.91183001100339E-17,-9.44295772567882E-18));
#8460=DIRECTION('ref_axis',(-2.16484527094502E-17,0.309016994374948,0.951056516295153));
#8461=DIRECTION('center_axis',(1.,9.13490707893474E-17,-3.96100256656632E-17));
#8462=DIRECTION('ref_axis',(-2.16484527094502E-17,0.587785252292473,0.809016994374947));
#8463=DIRECTION('center_axis',(1.,7.46379579533984E-17,-6.58997883142157E-17));
#8464=DIRECTION('ref_axis',(-2.16484527094502E-17,0.809016994374947,0.587785252292473));
#8465=DIRECTION('center_axis',(1.,5.0620761759739E-17,-8.57388205317489E-17));
#8466=DIRECTION('ref_axis',(-2.16484527094502E-17,0.951056516295154,0.309016994374947));
#8467=DIRECTION('center_axis',(1.,2.16484527094502E-17,-9.71851396181453E-17));
#8468=DIRECTION('ref_axis',(-2.16484527094502E-17,1.,-6.12323399573677E-17));
#8469=DIRECTION('center_axis',(1.,-9.44295772567882E-18,-9.91183001100339E-17));
#8470=DIRECTION('ref_axis',(-2.16484527094502E-17,0.951056516295154,-0.309016994374948));
#8471=DIRECTION('center_axis',(1.,-3.96100256656632E-17,-9.13490707893474E-17));
#8472=DIRECTION('ref_axis',(-2.16484527094502E-17,0.809016994374947,-0.587785252292473));
#8473=DIRECTION('center_axis',(1.,-6.58997883142157E-17,-7.46379579533984E-17));
#8474=DIRECTION('ref_axis',(-2.16484527094502E-17,0.587785252292473,-0.809016994374947));
#8475=DIRECTION('center_axis',(1.,-8.57388205317489E-17,-5.0620761759739E-17));
#8476=DIRECTION('ref_axis',(-2.16484527094502E-17,0.309016994374947,-0.951056516295154));
#8477=DIRECTION('center_axis',(1.,-9.71851396181453E-17,-2.16484527094502E-17));
#8478=DIRECTION('ref_axis',(-2.16484527094502E-17,0.,-1.));
#8479=DIRECTION('center_axis',(1.,0.,0.));
#8480=DIRECTION('ref_axis',(0.,0.,-1.));
#9764=CARTESIAN_POINT('',(0.,0.,0.));
#9765=CARTESIAN_POINT('Origin',(13.3251262658471,0.,0.));
#9766=CARTESIAN_POINT('',(14.7056733117529,-13.405863146671,4.41802289075134E-12));
#9767=CARTESIAN_POINT('',(10.5501326772895,-9.61762388247333,-2.19193273745671E-10));
#9768=CARTESIAN_POINT('',(13.3251262658471,-12.1473403730037,-1.48762015059523E-15));
#9769=CARTESIAN_POINT('',(10.0502525316942,-9.05620683581208,1.38781479615277));
#9770=CARTESIAN_POINT('Ctrl Pts',(14.7056733117529,-13.405863146671,8.83775691518096E-12));
#9771=CARTESIAN_POINT('Ctrl Pts',(14.1100932095804,-12.8629253856219,0.176689529340777));
#9772=CARTESIAN_POINT('Ctrl Pts',(13.5158390354049,-12.3177128141581,0.353880322328605));
#9773=CARTESIAN_POINT('Ctrl Pts',(11.9766359241915,-10.8925118431821,0.813848738908495));
#9774=CARTESIAN_POINT('Ctrl Pts',(10.9888514793465,-9.96433939118444,1.11043953280469));
#9775=CARTESIAN_POINT('Ctrl Pts',(10.0502525316942,-9.05620683581207,1.38781479615277));
#9776=CARTESIAN_POINT('',(10.0502525316942,-9.15961421508102,0.205863042617261));
#9777=CARTESIAN_POINT('Origin',(10.0502525316942,0.,0.));
#9778=CARTESIAN_POINT('Ctrl Pts',(10.0502525316942,-9.15961421508102,0.20586304261726));
#9779=CARTESIAN_POINT('Ctrl Pts',(10.215181575916,-9.311523886516,0.138211917211072));
#9780=CARTESIAN_POINT('Ctrl Pts',(10.3819612210757,-9.46431682339903,0.0694917893468868));
#9781=CARTESIAN_POINT('Ctrl Pts',(10.5501326772895,-9.61762388247333,-4.38387486034753E-10));
#9782=CARTESIAN_POINT('Origin',(24.5,-9.875,0.));
#9783=CARTESIAN_POINT('',(22.2,-10.,0.));
#9784=CARTESIAN_POINT('',(24.5,-9.78106229945361,2.08106229945361));
#9785=CARTESIAN_POINT('Ctrl Pts',(22.2,-10.,-3.46944695195361E-17));
#9786=CARTESIAN_POINT('Ctrl Pts',(22.2,-10.,0.279281663145492));
#9787=CARTESIAN_POINT('Ctrl Pts',(22.2664319537276,-9.98711221417022,0.57235161892421));
#9788=CARTESIAN_POINT('Ctrl Pts',(22.5234308581959,-9.94287664809831,1.09963640431428));
#9789=CARTESIAN_POINT('Ctrl Pts',(22.7136761128309,-9.91228969341567,1.33407151029786));
#9790=CARTESIAN_POINT('Ctrl Pts',(23.1318392128932,-9.8577299734025,1.69022028358443));
#9791=CARTESIAN_POINT('Ctrl Pts',(23.3865793433932,-9.82998540360157,1.83883276387722));
#9792=CARTESIAN_POINT('Ctrl Pts',(23.9342975404997,-9.79141246827269,2.03424683169264));
#9793=CARTESIAN_POINT('Ctrl Pts',(24.2273042269987,-9.78106229945361,2.08106229945361));
#9794=CARTESIAN_POINT('Ctrl Pts',(24.5,-9.78106229945361,2.08106229945361));
#9795=CARTESIAN_POINT('',(26.8,-10.,0.));
#9796=CARTESIAN_POINT('Ctrl Pts',(26.8,-10.,1.04083408558608E-15));
#9797=CARTESIAN_POINT('Ctrl Pts',(26.8,-10.,-0.279281663145491));
#9798=CARTESIAN_POINT('Ctrl Pts',(26.7335680462724,-9.98711221417022,-0.57235161892421));
#9799=CARTESIAN_POINT('Ctrl Pts',(26.4765691418041,-9.94287664809831,-1.09963640431428));
#9800=CARTESIAN_POINT('Ctrl Pts',(26.2863238871692,-9.91228969341567,-1.33407151029786));
#9801=CARTESIAN_POINT('Ctrl Pts',(25.8681607871068,-9.8577299734025,-1.69022028358443));
#9802=CARTESIAN_POINT('Ctrl Pts',(25.6134206566068,-9.82998540360157,-1.83883276387722));
#9803=CARTESIAN_POINT('Ctrl Pts',(25.0657024595003,-9.79141246827269,-2.03424683169264));
#9804=CARTESIAN_POINT('Ctrl Pts',(24.7726957730013,-9.78106229945362,-2.08106229945361));
#9805=CARTESIAN_POINT('Ctrl Pts',(24.5,-9.78106229945362,-2.08106229945361));
#9806=CARTESIAN_POINT('Ctrl Pts',(24.2273042269987,-9.78106229945362,-2.08106229945361));
#9807=CARTESIAN_POINT('Ctrl Pts',(23.9342975404997,-9.79141246827269,-2.03424683169264));
#9808=CARTESIAN_POINT('Ctrl Pts',(23.3865793433932,-9.82998540360157,-1.83883276387722));
#9809=CARTESIAN_POINT('Ctrl Pts',(23.1318392128932,-9.8577299734025,-1.69022028358443));
#9810=CARTESIAN_POINT('Ctrl Pts',(22.7136761128309,-9.91228969341567,-1.33407151029786));
#9811=CARTESIAN_POINT('Ctrl Pts',(22.5234308581959,-9.94287664809831,-1.09963640431428));
#9812=CARTESIAN_POINT('Ctrl Pts',(22.2664319537276,-9.98711221417022,-0.572351618924211));
#9813=CARTESIAN_POINT('Ctrl Pts',(22.2,-10.,-0.279281663145492));
#9814=CARTESIAN_POINT('Ctrl Pts',(22.2,-10.,4.85722573273506E-16));
#9815=CARTESIAN_POINT('Ctrl Pts',(24.5,-9.78106229945361,2.08106229945361));
#9816=CARTESIAN_POINT('Ctrl Pts',(24.7726957730013,-9.78106229945361,2.08106229945361));
#9817=CARTESIAN_POINT('Ctrl Pts',(25.0657024595003,-9.79141246827269,2.03424683169264));
#9818=CARTESIAN_POINT('Ctrl Pts',(25.6134206566068,-9.82998540360157,1.83883276387722));
#9819=CARTESIAN_POINT('Ctrl Pts',(25.8681607871068,-9.8577299734025,1.69022028358443));
#9820=CARTESIAN_POINT('Ctrl Pts',(26.2863238871692,-9.91228969341567,1.33407151029786));
#9821=CARTESIAN_POINT('Ctrl Pts',(26.4765691418041,-9.94287664809831,1.09963640431428));
#9822=CARTESIAN_POINT('Ctrl Pts',(26.7335680462724,-9.98711221417022,0.572351618924211));
#9823=CARTESIAN_POINT('Ctrl Pts',(26.8,-10.,0.279281663145492));
#9824=CARTESIAN_POINT('Ctrl Pts',(26.8,-10.,-2.08166817117217E-16));
#9825=CARTESIAN_POINT('',(24.5,-9.75,2.05));
#9826=CARTESIAN_POINT('',(24.5,-9.875,2.175));
#9827=CARTESIAN_POINT('Origin',(24.5,-9.75,0.));
#9828=CARTESIAN_POINT('Origin',(24.5,-7.75,0.));
#9829=CARTESIAN_POINT('',(24.5,-5.66552071746278,2.05));
#9830=CARTESIAN_POINT('',(24.5,-7.75,2.05));
#9831=CARTESIAN_POINT('',(26.55,-6.025,-3.34230378723604E-16));
#9832=CARTESIAN_POINT('Ctrl Pts',(26.55,-6.025,1.38777878078145E-16));
#9833=CARTESIAN_POINT('Ctrl Pts',(26.55,-6.025,0.259594733817565));
#9834=CARTESIAN_POINT('Ctrl Pts',(26.4976983668916,-6.00658123724956,0.535111320788412));
#9835=CARTESIAN_POINT('Ctrl Pts',(26.287830413716,-5.94008056213222,1.03961781502895));
#9836=CARTESIAN_POINT('Ctrl Pts',(26.13037388806,-5.8928399020443,1.26876391480488));
#9837=CARTESIAN_POINT('Ctrl Pts',(25.7686724003374,-5.80318375449856,1.63046540252745));
#9838=CARTESIAN_POINT('Ctrl Pts',(25.5395625840329,-5.75468697285078,1.78785157007388));
#9839=CARTESIAN_POINT('Ctrl Pts',(25.035191264494,-5.68525838031662,1.99766693028397));
#9840=CARTESIAN_POINT('Ctrl Pts',(24.7597261277258,-5.66552071746278,2.05));
#9841=CARTESIAN_POINT('Ctrl Pts',(24.5,-5.66552071746278,2.05));
#9842=CARTESIAN_POINT('',(22.45,-6.025,-6.81175073918965E-16));
#9843=CARTESIAN_POINT('Ctrl Pts',(22.45,-6.025,-6.24500451351651E-16));
#9844=CARTESIAN_POINT('Ctrl Pts',(22.45,-6.025,-0.259594733817566));
#9845=CARTESIAN_POINT('Ctrl Pts',(22.5023016331084,-6.00658123724956,-0.535111320788414));
#9846=CARTESIAN_POINT('Ctrl Pts',(22.712169586284,-5.94008056213222,-1.03961781502895));
#9847=CARTESIAN_POINT('Ctrl Pts',(22.86962611194,-5.8928399020443,-1.26876391480488));
#9848=CARTESIAN_POINT('Ctrl Pts',(23.2313275996626,-5.80318375449856,-1.63046540252745));
#9849=CARTESIAN_POINT('Ctrl Pts',(23.4604374159671,-5.75468697285078,-1.78785157007388));
#9850=CARTESIAN_POINT('Ctrl Pts',(23.964808735506,-5.68525838031662,-1.99766693028397));
#9851=CARTESIAN_POINT('Ctrl Pts',(24.2402738722742,-5.66552071746278,-2.05));
#9852=CARTESIAN_POINT('Ctrl Pts',(24.7597261277258,-5.66552071746278,-2.05));
#9853=CARTESIAN_POINT('Ctrl Pts',(25.035191264494,-5.68525838031662,-1.99766693028397));
#9854=CARTESIAN_POINT('Ctrl Pts',(25.5395625840329,-5.75468697285078,-1.78785157007388));
#9855=CARTESIAN_POINT('Ctrl Pts',(25.7686724003374,-5.80318375449856,-1.63046540252745));
#9856=CARTESIAN_POINT('Ctrl Pts',(26.13037388806,-5.8928399020443,-1.26876391480488));
#9857=CARTESIAN_POINT('Ctrl Pts',(26.287830413716,-5.94008056213222,-1.03961781502895));
#9858=CARTESIAN_POINT('Ctrl Pts',(26.4976983668916,-6.00658123724956,-0.535111320788414));
#9859=CARTESIAN_POINT('Ctrl Pts',(26.55,-6.025,-0.259594733817566));
#9860=CARTESIAN_POINT('Ctrl Pts',(26.55,-6.025,-6.24500451351651E-16));
#9861=CARTESIAN_POINT('Ctrl Pts',(24.5,-5.66552071746278,2.05));
#9862=CARTESIAN_POINT('Ctrl Pts',(24.2402738722742,-5.66552071746278,2.05));
#9863=CARTESIAN_POINT('Ctrl Pts',(23.964808735506,-5.68525838031662,1.99766693028397));
#9864=CARTESIAN_POINT('Ctrl Pts',(23.4604374159671,-5.75468697285078,1.78785157007388));
#9865=CARTESIAN_POINT('Ctrl Pts',(23.2313275996626,-5.80318375449856,1.63046540252745));
#9866=CARTESIAN_POINT('Ctrl Pts',(22.86962611194,-5.8928399020443,1.26876391480488));
#9867=CARTESIAN_POINT('Ctrl Pts',(22.712169586284,-5.94008056213222,1.03961781502895));
#9868=CARTESIAN_POINT('Ctrl Pts',(22.5023016331084,-6.00658123724956,0.535111320788414));
#9869=CARTESIAN_POINT('Ctrl Pts',(22.45,-6.025,0.259594733817566));
#9870=CARTESIAN_POINT('Ctrl Pts',(22.45,-6.025,0.));
#9871=CARTESIAN_POINT('Origin',(24.5,0.,9.875));
#9872=CARTESIAN_POINT('',(22.2,0.,10.));
#9873=CARTESIAN_POINT('',(26.8,0.,10.));
#9874=CARTESIAN_POINT('Ctrl Pts',(22.2,-2.77555756156289E-16,10.));
#9875=CARTESIAN_POINT('Ctrl Pts',(22.2,0.279281663145492,10.));
#9876=CARTESIAN_POINT('Ctrl Pts',(22.2664319537276,0.57235161892421,9.98711221417022));
#9877=CARTESIAN_POINT('Ctrl Pts',(22.5234308581959,1.09963640431428,9.94287664809831));
#9878=CARTESIAN_POINT('Ctrl Pts',(22.7136761128309,1.33407151029786,9.91228969341567));
#9879=CARTESIAN_POINT('Ctrl Pts',(23.1318392128932,1.69022028358443,9.8577299734025));
#9880=CARTESIAN_POINT('Ctrl Pts',(23.3865793433932,1.83883276387722,9.82998540360157));
#9881=CARTESIAN_POINT('Ctrl Pts',(23.9342975404997,2.03424683169264,9.79141246827269));
#9882=CARTESIAN_POINT('Ctrl Pts',(24.2273042269987,2.08106229945361,9.78106229945362));
#9883=CARTESIAN_POINT('Ctrl Pts',(24.7726957730013,2.08106229945361,9.78106229945362));
#9884=CARTESIAN_POINT('Ctrl Pts',(25.0657024595003,2.03424683169264,9.79141246827269));
#9885=CARTESIAN_POINT('Ctrl Pts',(25.6134206566068,1.83883276387722,9.82998540360157));
#9886=CARTESIAN_POINT('Ctrl Pts',(25.8681607871068,1.69022028358443,9.8577299734025));
#9887=CARTESIAN_POINT('Ctrl Pts',(26.2863238871692,1.33407151029786,9.91228969341567));
#9888=CARTESIAN_POINT('Ctrl Pts',(26.4765691418041,1.09963640431428,9.94287664809831));
#9889=CARTESIAN_POINT('Ctrl Pts',(26.7335680462724,0.572351618924211,9.98711221417022));
#9890=CARTESIAN_POINT('Ctrl Pts',(26.8,0.279281663145492,10.));
#9891=CARTESIAN_POINT('Ctrl Pts',(26.8,0.,10.));
#9892=CARTESIAN_POINT('',(22.45,2.51052593825207E-16,9.75));
#9893=CARTESIAN_POINT('',(22.325,2.66360678814549E-16,9.875));
#9894=CARTESIAN_POINT('Origin',(24.5,0.,9.75));
#9895=CARTESIAN_POINT('Ctrl Pts',(26.8,1.31838984174237E-15,10.));
#9896=CARTESIAN_POINT('Ctrl Pts',(26.8,-0.279281663145491,10.));
#9897=CARTESIAN_POINT('Ctrl Pts',(26.7335680462724,-0.572351618924209,9.98711221417022));
#9898=CARTESIAN_POINT('Ctrl Pts',(26.4765691418041,-1.09963640431428,9.94287664809831));
#9899=CARTESIAN_POINT('Ctrl Pts',(26.2863238871692,-1.33407151029786,9.91228969341567));
#9900=CARTESIAN_POINT('Ctrl Pts',(25.8681607871068,-1.69022028358443,9.8577299734025));
#9901=CARTESIAN_POINT('Ctrl Pts',(25.6134206566068,-1.83883276387722,9.82998540360157));
#9902=CARTESIAN_POINT('Ctrl Pts',(25.0657024595003,-2.03424683169264,9.79141246827269));
#9903=CARTESIAN_POINT('Ctrl Pts',(24.7726957730013,-2.08106229945361,9.78106229945362));
#9904=CARTESIAN_POINT('Ctrl Pts',(24.5,-2.08106229945361,9.78106229945362));
#9905=CARTESIAN_POINT('Ctrl Pts',(24.2273042269987,-2.08106229945361,9.78106229945362));
#9906=CARTESIAN_POINT('Ctrl Pts',(23.9342975404997,-2.03424683169264,9.79141246827269));
#9907=CARTESIAN_POINT('Ctrl Pts',(23.3865793433932,-1.83883276387722,9.82998540360157));
#9908=CARTESIAN_POINT('Ctrl Pts',(23.1318392128932,-1.69022028358443,9.8577299734025));
#9909=CARTESIAN_POINT('Ctrl Pts',(22.7136761128309,-1.33407151029786,9.91228969341567));
#9910=CARTESIAN_POINT('Ctrl Pts',(22.5234308581959,-1.09963640431428,9.94287664809831));
#9911=CARTESIAN_POINT('Ctrl Pts',(22.2664319537276,-0.572351618924211,9.98711221417022));
#9912=CARTESIAN_POINT('Ctrl Pts',(22.2,-0.279281663145492,10.));
#9913=CARTESIAN_POINT('Ctrl Pts',(22.2,3.46944695195361E-16,10.));
#9914=CARTESIAN_POINT('Origin',(24.5,0.,7.75));
#9915=CARTESIAN_POINT('',(22.45,1.94915235951676E-16,6.025));
#9916=CARTESIAN_POINT('',(22.45,2.51052593825207E-16,7.75));
#9917=CARTESIAN_POINT('',(24.5,2.05,5.66552071746278));
#9918=CARTESIAN_POINT('Ctrl Pts',(24.5,2.05,5.66552071746278));
#9919=CARTESIAN_POINT('Ctrl Pts',(24.2402738722742,2.05,5.66552071746278));
#9920=CARTESIAN_POINT('Ctrl Pts',(23.964808735506,1.99766693028397,5.68525838031662));
#9921=CARTESIAN_POINT('Ctrl Pts',(23.4604374159671,1.78785157007388,5.75468697285078));
#9922=CARTESIAN_POINT('Ctrl Pts',(23.2313275996626,1.63046540252745,5.80318375449856));
#9923=CARTESIAN_POINT('Ctrl Pts',(22.86962611194,1.26876391480488,5.8928399020443));
#9924=CARTESIAN_POINT('Ctrl Pts',(22.712169586284,1.03961781502895,5.94008056213222));
#9925=CARTESIAN_POINT('Ctrl Pts',(22.5023016331084,0.535111320788414,6.00658123724956));
#9926=CARTESIAN_POINT('Ctrl Pts',(22.45,0.259594733817566,6.025));
#9927=CARTESIAN_POINT('Ctrl Pts',(22.45,2.77555756156289E-16,6.025));
#9928=CARTESIAN_POINT('Ctrl Pts',(22.45,2.08166817117217E-16,6.025));
#9929=CARTESIAN_POINT('Ctrl Pts',(22.45,-0.259594733817565,6.025));
#9930=CARTESIAN_POINT('Ctrl Pts',(22.5023016331084,-0.535111320788413,6.00658123724956));
#9931=CARTESIAN_POINT('Ctrl Pts',(22.712169586284,-1.03961781502895,5.94008056213222));
#9932=CARTESIAN_POINT('Ctrl Pts',(22.86962611194,-1.26876391480488,5.8928399020443));
#9933=CARTESIAN_POINT('Ctrl Pts',(23.2313275996626,-1.63046540252745,5.80318375449856));
#9934=CARTESIAN_POINT('Ctrl Pts',(23.4604374159671,-1.78785157007388,5.75468697285078));
#9935=CARTESIAN_POINT('Ctrl Pts',(23.964808735506,-1.99766693028397,5.68525838031662));
#9936=CARTESIAN_POINT('Ctrl Pts',(24.2402738722742,-2.05,5.66552071746278));
#9937=CARTESIAN_POINT('Ctrl Pts',(24.7597261277258,-2.05,5.66552071746278));
#9938=CARTESIAN_POINT('Ctrl Pts',(25.035191264494,-1.99766693028397,5.68525838031662));
#9939=CARTESIAN_POINT('Ctrl Pts',(25.5395625840329,-1.78785157007388,5.75468697285078));
#9940=CARTESIAN_POINT('Ctrl Pts',(25.7686724003374,-1.63046540252745,5.80318375449856));
#9941=CARTESIAN_POINT('Ctrl Pts',(26.13037388806,-1.26876391480488,5.8928399020443));
#9942=CARTESIAN_POINT('Ctrl Pts',(26.287830413716,-1.03961781502895,5.94008056213222));
#9943=CARTESIAN_POINT('Ctrl Pts',(26.4976983668916,-0.535111320788413,6.00658123724956));
#9944=CARTESIAN_POINT('Ctrl Pts',(26.55,-0.259594733817566,6.025));
#9945=CARTESIAN_POINT('Ctrl Pts',(26.55,0.259594733817565,6.025));
#9946=CARTESIAN_POINT('Ctrl Pts',(26.4976983668916,0.535111320788412,6.00658123724956));
#9947=CARTESIAN_POINT('Ctrl Pts',(26.287830413716,1.03961781502895,5.94008056213222));
#9948=CARTESIAN_POINT('Ctrl Pts',(26.13037388806,1.26876391480488,5.8928399020443));
#9949=CARTESIAN_POINT('Ctrl Pts',(25.7686724003374,1.63046540252745,5.80318375449856));
#9950=CARTESIAN_POINT('Ctrl Pts',(25.5395625840329,1.78785157007388,5.75468697285078));
#9951=CARTESIAN_POINT('Ctrl Pts',(25.035191264494,1.99766693028397,5.68525838031662));
#9952=CARTESIAN_POINT('Ctrl Pts',(24.7597261277258,2.05,5.66552071746278));
#9953=CARTESIAN_POINT('Ctrl Pts',(24.5,2.05,5.66552071746278));
#9954=CARTESIAN_POINT('Origin',(10.3002525316942,0.,0.));
#9955=CARTESIAN_POINT('',(10.0502525316942,6.525,-7.99082036443648E-16));
#9956=CARTESIAN_POINT('Origin',(10.0502525316942,0.,0.));
#9957=CARTESIAN_POINT('',(10.5502525316942,6.025,7.3784969648628E-16));
#9958=CARTESIAN_POINT('',(10.3002525316942,6.275,-7.68465866464964E-16));
#9959=CARTESIAN_POINT('',(10.5502525316942,-6.025,-7.3784969648628E-16));
#9960=CARTESIAN_POINT('Origin',(10.5502525316942,0.,0.));
#9961=CARTESIAN_POINT('Origin',(10.5502525316942,0.,0.));
#9962=CARTESIAN_POINT('Origin',(19.7001262658471,0.,0.));
#9963=CARTESIAN_POINT('',(28.85,6.025,-7.3784969648628E-16));
#9964=CARTESIAN_POINT('',(28.85,-6.025,-7.3784969648628E-16));
#9965=CARTESIAN_POINT('Origin',(28.85,0.,0.));
#9966=CARTESIAN_POINT('Origin',(28.85,0.,0.));
#9967=CARTESIAN_POINT('',(19.7001262658471,-6.025,-7.3784969648628E-16));
#9968=CARTESIAN_POINT('',(19.7001262658471,-6.025,-7.3784969648628E-16));
#9969=CARTESIAN_POINT('Origin',(10.0502525316942,9.16192731696939,0.));
#9970=CARTESIAN_POINT('',(10.0502525316942,8.18410616705958,-4.11841212213243));
#9971=CARTESIAN_POINT('',(10.0502525316942,8.64769560732005,-3.02626384252387));
#9972=CARTESIAN_POINT('Origin',(10.0502525316942,0.,0.));
#9973=CARTESIAN_POINT('',(10.0502525316942,9.2755658561365,-5.45537535466284));
#9974=CARTESIAN_POINT('Ctrl Pts',(10.0502525316942,8.18410616705958,-4.11841212213243));
#9975=CARTESIAN_POINT('Ctrl Pts',(10.0502525316942,8.19431842617809,-4.12237383820348));
#9976=CARTESIAN_POINT('Ctrl Pts',(10.0502525316942,8.21464735012275,-4.1304870856583));
#9977=CARTESIAN_POINT('Ctrl Pts',(10.0502525316942,8.24485395393399,-4.14322640185693));
#9978=CARTESIAN_POINT('Ctrl Pts',(10.0502525316942,8.28455481633258,-4.16135311687778));
#9979=CARTESIAN_POINT('Ctrl Pts',(10.0502525316942,8.33321297157003,-4.18592891379899));
#9980=CARTESIAN_POINT('Ctrl Pts',(10.0502525316942,8.38088287416164,-4.21244876582417));
#9981=CARTESIAN_POINT('Ctrl Pts',(10.0502525316942,8.42753204825146,-4.24094982636281));
#9982=CARTESIAN_POINT('Ctrl Pts',(10.0502525316942,8.47311320506822,-4.27147990109806));
#9983=CARTESIAN_POINT('Ctrl Pts',(10.0502525316942,8.51756357237276,-4.3040953182409));
#9984=CARTESIAN_POINT('Ctrl Pts',(10.0502525316942,8.56081999110915,-4.33884232599626));
#9985=CARTESIAN_POINT('Ctrl Pts',(10.0502525316942,8.60283329387128,-4.37573883085758));
#9986=CARTESIAN_POINT('Ctrl Pts',(10.0502525316942,8.6435823082099,-4.41475679767577));
#9987=CARTESIAN_POINT('Ctrl Pts',(10.0502525316942,8.68309075792173,-4.45580026211617));
#9988=CARTESIAN_POINT('Ctrl Pts',(10.0502525316942,8.72143659100306,-4.4986943294444));
#9989=CARTESIAN_POINT('Ctrl Pts',(10.0502525316942,8.75872782924178,-4.54322265243728));
#9990=CARTESIAN_POINT('Ctrl Pts',(10.0502525316942,8.79508318101477,-4.58915808705618));
#9991=CARTESIAN_POINT('Ctrl Pts',(10.0502525316942,8.83061212429863,-4.63629390238203));
#9992=CARTESIAN_POINT('Ctrl Pts',(10.0502525316942,8.86539310688376,-4.68447828052063));
#9993=CARTESIAN_POINT('Ctrl Pts',(10.0502525316942,8.89945965089929,-4.73363584056076));
#9994=CARTESIAN_POINT('Ctrl Pts',(10.0502525316942,8.93281562325407,-4.78374147310216));
#9995=CARTESIAN_POINT('Ctrl Pts',(10.0502525316942,8.96544592744964,-4.83480166455838));
#9996=CARTESIAN_POINT('Ctrl Pts',(10.0502525316942,8.99732855257362,-4.88683372770265));
#9997=CARTESIAN_POINT('Ctrl Pts',(10.0502525316942,9.02844713284016,-4.9398440174493));
#9998=CARTESIAN_POINT('Ctrl Pts',(10.0502525316942,9.05880038387882,-4.99381190670161));
#9999=CARTESIAN_POINT('Ctrl Pts',(10.0502525316942,9.08839676934597,-5.04870046735128));
#10000=CARTESIAN_POINT('Ctrl Pts',(10.0502525316942,9.11725155657582,-5.10446294828982));
#10001=CARTESIAN_POINT('Ctrl Pts',(10.0502525316942,9.14538320175401,-5.16105047473192));
#10002=CARTESIAN_POINT('Ctrl Pts',(10.0502525316942,9.17281011362288,-5.21841931731543));
#10003=CARTESIAN_POINT('Ctrl Pts',(10.0502525316942,9.19954772791879,-5.27653724822262));
#10004=CARTESIAN_POINT('Ctrl Pts',(10.0502525316942,9.2256083913841,-5.33538160688598));
#10005=CARTESIAN_POINT('Ctrl Pts',(10.0502525316942,9.24592251158686,-5.38302685274804));
#10006=CARTESIAN_POINT('Ctrl Pts',(10.0502525316942,9.26085993003723,-5.41907797515233));
#10007=CARTESIAN_POINT('Ctrl Pts',(10.0502525316942,9.27068592765741,-5.44325277512453));
#10008=CARTESIAN_POINT('Ctrl Pts',(10.0502525316942,9.2755658561365,-5.45537535466284));
#10009=CARTESIAN_POINT('',(10.0502525316942,7.28928030147641,-5.55043285230422));
#10010=CARTESIAN_POINT('Ctrl Pts',(10.0502525316942,9.2755658561365,-5.45537535466284));
#10011=CARTESIAN_POINT('Ctrl Pts',(10.0502525316942,9.25004353985722,-5.48408843121132));
#10012=CARTESIAN_POINT('Ctrl Pts',(10.0502525316942,9.19987743117415,-5.53944326709657));
#10013=CARTESIAN_POINT('Ctrl Pts',(10.0502525316942,9.12726384869626,-5.61626154813455));
#10014=CARTESIAN_POINT('Ctrl Pts',(10.0502525316942,9.03572636773682,-5.70623565557996));
#10015=CARTESIAN_POINT('Ctrl Pts',(10.0502525316942,8.93010252395574,-5.79796105654696));
#10016=CARTESIAN_POINT('Ctrl Pts',(10.0502525316942,8.83316895299322,-5.86920138549131));
#10017=CARTESIAN_POINT('Ctrl Pts',(10.0502525316942,8.74463793548674,-5.92064129305387));
#10018=CARTESIAN_POINT('Ctrl Pts',(10.0502525316942,8.6639539190358,-5.95360120899604));
#10019=CARTESIAN_POINT('Ctrl Pts',(10.0502525316942,8.59022668922188,-5.97019580138365));
#10020=CARTESIAN_POINT('Ctrl Pts',(10.0502525316942,8.52210226517413,-5.97364002234323));
#10021=CARTESIAN_POINT('Ctrl Pts',(10.0502525316942,8.45790665865659,-5.96790845784416));
#10022=CARTESIAN_POINT('Ctrl Pts',(10.0502525316942,8.39592031140414,-5.95708504467347));
#10023=CARTESIAN_POINT('Ctrl Pts',(10.0502525316942,8.33461788057945,-5.94479472837688));
#10024=CARTESIAN_POINT('Ctrl Pts',(10.0502525316942,8.27290485770376,-5.93364300051867));
#10025=CARTESIAN_POINT('Ctrl Pts',(10.0502525316942,8.2104048870761,-5.92453426026728));
#10026=CARTESIAN_POINT('Ctrl Pts',(10.0502525316942,8.14730848207823,-5.91703766966772));
#10027=CARTESIAN_POINT('Ctrl Pts',(10.0502525316942,8.08413710664289,-5.90995523970614));
#10028=CARTESIAN_POINT('Ctrl Pts',(10.0502525316942,8.02154163982398,-5.90180775582857));
#10029=CARTESIAN_POINT('Ctrl Pts',(10.0502525316942,7.96008352176745,-5.89136254542228));
#10030=CARTESIAN_POINT('Ctrl Pts',(10.0502525316942,7.90003527315714,-5.87811409765682));
#10031=CARTESIAN_POINT('Ctrl Pts',(10.0502525316942,7.84146798659238,-5.86206014174823));
#10032=CARTESIAN_POINT('Ctrl Pts',(10.0502525316942,7.78432826524869,-5.84350339850201));
#10033=CARTESIAN_POINT('Ctrl Pts',(10.0502525316942,7.72851334381364,-5.82285820956226));
#10034=CARTESIAN_POINT('Ctrl Pts',(10.0502525316942,7.67395636265026,-5.80043066085533));
#10035=CARTESIAN_POINT('Ctrl Pts',(10.0502525316942,7.62067331151744,-5.77629688888814));
#10036=CARTESIAN_POINT('Ctrl Pts',(10.0502525316942,7.56872566186653,-5.75039773581461));
#10037=CARTESIAN_POINT('Ctrl Pts',(10.0502525316942,7.51819950516883,-5.72259034420254));
#10038=CARTESIAN_POINT('Ctrl Pts',(10.0502525316942,7.46918012077942,-5.69271190798352));
#10039=CARTESIAN_POINT('Ctrl Pts',(10.0502525316942,7.42172307293681,-5.66064997807339));
#10040=CARTESIAN_POINT('Ctrl Pts',(10.0502525316942,7.37585243997691,-5.62635178473812));
#10041=CARTESIAN_POINT('Ctrl Pts',(10.0502525316942,7.34042983445952,-5.59710957827922));
#10042=CARTESIAN_POINT('Ctrl Pts',(10.0502525316942,7.31457760934185,-5.5741645986968));
#10043=CARTESIAN_POINT('Ctrl Pts',(10.0502525316942,7.2976598885924,-5.55841836363355));
#10044=CARTESIAN_POINT('Ctrl Pts',(10.0502525316942,7.28928030147641,-5.55043285230422));
#10045=CARTESIAN_POINT('',(10.0502525316942,6.51088816465465,-6.44587057493322));
#10046=CARTESIAN_POINT('Origin',(10.0502525316942,0.,0.));
#10047=CARTESIAN_POINT('',(10.0502525316942,7.13578365451837,-8.05467776187827));
#10048=CARTESIAN_POINT('Ctrl Pts',(10.0502525316942,6.51088816465465,-6.44587057493322));
#10049=CARTESIAN_POINT('Ctrl Pts',(10.0502525316942,6.51937636264256,-6.45279415243689));
#10050=CARTESIAN_POINT('Ctrl Pts',(10.0502525316942,6.5362031868863,-6.46679229227336));
#10051=CARTESIAN_POINT('Ctrl Pts',(10.0502525316942,6.56099470907402,-6.48824245587723));
#10052=CARTESIAN_POINT('Ctrl Pts',(10.0502525316942,6.59315100996711,-6.51775022748935));
#10053=CARTESIAN_POINT('Ctrl Pts',(10.0502525316942,6.63183332667763,-6.55615939617772));
#10054=CARTESIAN_POINT('Ctrl Pts',(10.0502525316942,6.66897501320444,-6.59611208427845));
#10055=CARTESIAN_POINT('Ctrl Pts',(10.0502525316942,6.7045337021382,-6.63763359119236));
#10056=CARTESIAN_POINT('Ctrl Pts',(10.0502525316942,6.73844964641633,-6.68075476979194));
#10057=CARTESIAN_POINT('Ctrl Pts',(10.0502525316942,6.77064573971725,-6.72550979370064));
#10058=CARTESIAN_POINT('Ctrl Pts',(10.0502525316942,6.801047622728,-6.77192313035348));
#10059=CARTESIAN_POINT('Ctrl Pts',(10.0502525316942,6.82960300105582,-6.81999661627367));
#10060=CARTESIAN_POINT('Ctrl Pts',(10.0502525316942,6.8563004018424,-6.86969704580336));
#10061=CARTESIAN_POINT('Ctrl Pts',(10.0502525316942,6.88119204236944,-6.92094048249309));
#10062=CARTESIAN_POINT('Ctrl Pts',(10.0502525316942,6.90440610103192,-6.97358467882161));
#10063=CARTESIAN_POINT('Ctrl Pts',(10.0502525316942,6.92611216762375,-7.02745725692073));
#10064=CARTESIAN_POINT('Ctrl Pts',(10.0502525316942,6.94649333188842,-7.08237887287822));
#10065=CARTESIAN_POINT('Ctrl Pts',(10.0502525316942,6.96571759693621,-7.13818674446165));
#10066=CARTESIAN_POINT('Ctrl Pts',(10.0502525316942,6.98390648535873,-7.19476072597386));
#10067=CARTESIAN_POINT('Ctrl Pts',(10.0502525316942,7.00111517257794,-7.25203948481561));
#10068=CARTESIAN_POINT('Ctrl Pts',(10.0502525316942,7.01735509547412,-7.31000033546873));
#10069=CARTESIAN_POINT('Ctrl Pts',(10.0502525316942,7.032609892012,-7.36864478180451));
#10070=CARTESIAN_POINT('Ctrl Pts',(10.0502525316942,7.04685327862879,-7.42798248750274));
#10071=CARTESIAN_POINT('Ctrl Pts',(10.0502525316942,7.06006772676068,-7.48801443914016));
#10072=CARTESIAN_POINT('Ctrl Pts',(10.0502525316942,7.07225838902223,-7.54872062228975));
#10073=CARTESIAN_POINT('Ctrl Pts',(10.0502525316942,7.08344472624202,-7.6100685316471));
#10074=CARTESIAN_POINT('Ctrl Pts',(10.0502525316942,7.09365570540476,-7.67201842213158));
#10075=CARTESIAN_POINT('Ctrl Pts',(10.0502525316942,7.10292398252533,-7.73452951433515));
#10076=CARTESIAN_POINT('Ctrl Pts',(10.0502525316942,7.11128057847415,-7.79756590777721));
#10077=CARTESIAN_POINT('Ctrl Pts',(10.0502525316942,7.11875013245223,-7.86110172188657));
#10078=CARTESIAN_POINT('Ctrl Pts',(10.0502525316942,7.12535138940982,-7.92511922053603));
#10079=CARTESIAN_POINT('Ctrl Pts',(10.0502525316942,7.1299480751289,-7.97670995045205));
#10080=CARTESIAN_POINT('Ctrl Pts',(10.0502525316942,7.13301399479354,-8.01561252148766));
#10081=CARTESIAN_POINT('Ctrl Pts',(10.0502525316942,7.13488864983229,-8.04164052278268));
#10082=CARTESIAN_POINT('Ctrl Pts',(10.0502525316942,7.13578365451837,-8.05467776187827));
#10083=CARTESIAN_POINT('',(10.0502525316942,5.21733945232202,-7.53128682236137));
#10084=CARTESIAN_POINT('Ctrl Pts',(10.0502525316942,7.13578365451837,-8.05467776187827));
#10085=CARTESIAN_POINT('Ctrl Pts',(10.0502525316942,7.10263766069576,-8.07409869096647));
#10086=CARTESIAN_POINT('Ctrl Pts',(10.0502525316942,7.03782127112617,-8.11124208821886));
#10087=CARTESIAN_POINT('Ctrl Pts',(10.0502525316942,6.94502349601963,-8.16186178396251));
#10088=CARTESIAN_POINT('Ctrl Pts',(10.0502525316942,6.83016265001357,-8.21914560790757));
#10089=CARTESIAN_POINT('Ctrl Pts',(10.0502525316942,6.70136369739476,-8.27374208546745));
#10090=CARTESIAN_POINT('Ctrl Pts',(10.0502525316942,6.58715992075444,-8.31154154378012));
#10091=CARTESIAN_POINT('Ctrl Pts',(10.0502525316942,6.48706611403475,-8.33310621412631));
#10092=CARTESIAN_POINT('Ctrl Pts',(10.0502525316942,6.40014588026892,-8.33952022470187));
#10093=CARTESIAN_POINT('Ctrl Pts',(10.0502525316942,6.32489910686351,-8.33251965296669));
#10094=CARTESIAN_POINT('Ctrl Pts',(10.0502525316942,6.25904460664514,-8.31474369699109));
#10095=CARTESIAN_POINT('Ctrl Pts',(10.0502525316942,6.19976210758369,-8.28945512184757));
#10096=CARTESIAN_POINT('Ctrl Pts',(10.0502525316942,6.14415420671479,-8.26000660950279));
#10097=CARTESIAN_POINT('Ctrl Pts',(10.0502525316942,6.08965004701613,-8.22937433118026));
#10098=CARTESIAN_POINT('Ctrl Pts',(10.0502525316942,6.03440354789477,-8.19969803488993));
#10099=CARTESIAN_POINT('Ctrl Pts',(10.0502525316942,5.9777772990961,-8.17172155504672));
#10100=CARTESIAN_POINT('Ctrl Pts',(10.0502525316942,5.92008562586321,-8.1450940122787));
#10101=CARTESIAN_POINT('Ctrl Pts',(10.0502525316942,5.86219466883171,-8.11883719254497));
#10102=CARTESIAN_POINT('Ctrl Pts',(10.0502525316942,5.80518055320261,-8.09174541189394));
#10103=CARTESIAN_POINT('Ctrl Pts',(10.0502525316942,5.74995815707107,-8.06281982355119));
#10104=CARTESIAN_POINT('Ctrl Pts',(10.0502525316942,5.69694287444674,-8.03166387167001));
#10105=CARTESIAN_POINT('Ctrl Pts',(10.0502525316942,5.6462030201203,-7.99829736542789));
#10106=CARTESIAN_POINT('Ctrl Pts',(10.0502525316942,5.59759426482043,-7.96299170889331));
#10107=CARTESIAN_POINT('Ctrl Pts',(10.0502525316942,5.5508908343176,-7.92610920815888));
#10108=CARTESIAN_POINT('Ctrl Pts',(10.0502525316942,5.50593455556538,-7.88792030747535));
#10109=CARTESIAN_POINT('Ctrl Pts',(10.0502525316942,5.46271710825365,-7.84850235807098));
#10110=CARTESIAN_POINT('Ctrl Pts',(10.0502525316942,5.42131523598658,-7.80781809321391));
#10111=CARTESIAN_POINT('Ctrl Pts',(10.0502525316942,5.38185496199325,-7.76575825114004));
#10112=CARTESIAN_POINT('Ctrl Pts',(10.0502525316942,5.34446770160195,-7.72219434684711));
#10113=CARTESIAN_POINT('Ctrl Pts',(10.0502525316942,5.3092410482218,-7.67703660519485));
#10114=CARTESIAN_POINT('Ctrl Pts',(10.0502525316942,5.27621420845565,-7.63024227979884));
#10115=CARTESIAN_POINT('Ctrl Pts',(10.0502525316942,5.251561647403,-7.59148510170534));
#10116=CARTESIAN_POINT('Ctrl Pts',(10.0502525316942,5.23406510887067,-7.56167435245346));
#10117=CARTESIAN_POINT('Ctrl Pts',(10.0502525316942,5.22284125454301,-7.54147092977177));
#10118=CARTESIAN_POINT('Ctrl Pts',(10.0502525316942,5.21733945232202,-7.53128682236137));
#10119=CARTESIAN_POINT('',(10.0502525316942,4.20033906466803,-8.14236230483842));
#10120=CARTESIAN_POINT('Origin',(10.0502525316942,0.,0.));
#10121=CARTESIAN_POINT('',(10.0502525316942,4.29750123086779,-9.86553218952114));
#10122=CARTESIAN_POINT('Ctrl Pts',(10.0502525316942,4.20033906466803,-8.14236230483842));
#10123=CARTESIAN_POINT('Ctrl Pts',(10.0502525316942,4.20627231756552,-8.15157001576925));
#10124=CARTESIAN_POINT('Ctrl Pts',(10.0502525316942,4.21794991531197,-8.17008281252941));
#10125=CARTESIAN_POINT('Ctrl Pts',(10.0502525316942,4.23489958895176,-8.1981441320729));
#10126=CARTESIAN_POINT('Ctrl Pts',(10.0502525316942,4.2563636455618,-8.23614453399815));
#10127=CARTESIAN_POINT('Ctrl Pts',(10.0502525316942,4.28128362907021,-8.28462731741005));
#10128=CARTESIAN_POINT('Ctrl Pts',(10.0502525316942,4.30426141247364,-8.33410199410829));
#10129=CARTESIAN_POINT('Ctrl Pts',(10.0502525316942,4.32524888402656,-8.38457953300338));
#10130=CARTESIAN_POINT('Ctrl Pts',(10.0502525316942,4.34417968683382,-8.43607081406306));
#10131=CARTESIAN_POINT('Ctrl Pts',(10.0502525316942,4.36096992819547,-8.48858451117083));
#10132=CARTESIAN_POINT('Ctrl Pts',(10.0502525316942,4.37554132734911,-8.54212091594884));
#10133=CARTESIAN_POINT('Ctrl Pts',(10.0502525316942,4.38784358185488,-8.59666561517837));
#10134=CARTESIAN_POINT('Ctrl Pts',(10.0502525316942,4.39787604148868,-8.65218348309394));
#10135=CARTESIAN_POINT('Ctrl Pts',(10.0502525316942,4.4057143056259,-8.70861082741579));
#10136=CARTESIAN_POINT('Ctrl Pts',(10.0502525316942,4.41152423606579,-8.76585197201427));
#10137=CARTESIAN_POINT('Ctrl Pts',(10.0502525316942,4.41552038997766,-8.82379538192297));
#10138=CARTESIAN_POINT('Ctrl Pts',(10.0502525316942,4.41793231637186,-8.88232706878773));
#10139=CARTESIAN_POINT('Ctrl Pts',(10.0502525316942,4.41897009817737,-8.94134413332185));
#10140=CARTESIAN_POINT('Ctrl Pts',(10.0502525316942,4.41878643730905,-9.00076986272314));
#10141=CARTESIAN_POINT('Ctrl Pts',(10.0502525316942,4.41745276152696,-9.06056297636652));
#10142=CARTESIAN_POINT('Ctrl Pts',(10.0502525316942,4.41498695816126,-9.12070543323243));
#10143=CARTESIAN_POINT('Ctrl Pts',(10.0502525316942,4.4113730012699,-9.18119360744053));
#10144=CARTESIAN_POINT('Ctrl Pts',(10.0502525316942,4.40658290745794,-9.24202856762888));
#10145=CARTESIAN_POINT('Ctrl Pts',(10.0502525316942,4.40059970120156,-9.3032058354636));
#10146=CARTESIAN_POINT('Ctrl Pts',(10.0502525316942,4.3934344677265,-9.36470796833893));
#10147=CARTESIAN_POINT('Ctrl Pts',(10.0502525316942,4.38511576007206,-9.42651006560004));
#10148=CARTESIAN_POINT('Ctrl Pts',(10.0502525316942,4.37568340938316,-9.48858327871958));
#10149=CARTESIAN_POINT('Ctrl Pts',(10.0502525316942,4.36518107490567,-9.55089891543934));
#10150=CARTESIAN_POINT('Ctrl Pts',(10.0502525316942,4.35364935309914,-9.61343241834946));
#10151=CARTESIAN_POINT('Ctrl Pts',(10.0502525316942,4.34111967477257,-9.67616678749592));
#10152=CARTESIAN_POINT('Ctrl Pts',(10.0502525316942,4.32761534819776,-9.73909094732754));
#10153=CARTESIAN_POINT('Ctrl Pts',(10.0502525316942,4.316044643808,-9.78957710119959));
#10154=CARTESIAN_POINT('Ctrl Pts',(10.0502525316942,4.30693895110861,-9.8275230661634));
#10155=CARTESIAN_POINT('Ctrl Pts',(10.0502525316942,4.30067875926925,-9.85285646666673));
#10156=CARTESIAN_POINT('Ctrl Pts',(10.0502525316942,4.29750123086779,-9.86553218952114));
#10157=CARTESIAN_POINT('',(10.0502525316942,2.63468906623289,-8.77492596468499));
#10158=CARTESIAN_POINT('Ctrl Pts',(10.0502525316942,4.29750123086779,-9.86553218952114));
#10159=CARTESIAN_POINT('Ctrl Pts',(10.0502525316942,4.25997612031891,-9.87375991529634));
#10160=CARTESIAN_POINT('Ctrl Pts',(10.0502525316942,4.18685412967622,-9.88905601939953));
#10161=CARTESIAN_POINT('Ctrl Pts',(10.0502525316942,4.08295585472858,-9.9085221213413));
#10162=CARTESIAN_POINT('Ctrl Pts',(10.0502525316942,3.95601502356553,-9.9275083219784));
#10163=CARTESIAN_POINT('Ctrl Pts',(10.0502525316942,3.81664870098641,-9.93963159251159));
#10164=CARTESIAN_POINT('Ctrl Pts',(10.0502525316942,3.69635378003033,-9.94029010584861));
#10165=CARTESIAN_POINT('Ctrl Pts',(10.0502525316942,3.59449506329372,-9.92986863879505));
#10166=CARTESIAN_POINT('Ctrl Pts',(10.0502525316942,3.50984697030288,-9.90910889595984));
#10167=CARTESIAN_POINT('Ctrl Pts',(10.0502525316942,3.44044633176199,-9.87919842483915));
#10168=CARTESIAN_POINT('Ctrl Pts',(10.0502525316942,3.38330805268968,-9.84194232635164));
#10169=CARTESIAN_POINT('Ctrl Pts',(10.0502525316942,3.3347416451379,-9.79957216249457));
#10170=CARTESIAN_POINT('Ctrl Pts',(10.0502525316942,3.29095547943263,-9.75438117654386));
#10171=CARTESIAN_POINT('Ctrl Pts',(10.0502525316942,3.24858483776411,-9.70840543702524));
#10172=CARTESIAN_POINT('Ctrl Pts',(10.0502525316942,3.20521277465607,-9.66310949495059));
#10173=CARTESIAN_POINT('Ctrl Pts',(10.0502525316942,3.16000321945708,-9.61900380828622));
#10174=CARTESIAN_POINT('Ctrl Pts',(10.0502525316942,3.11336354092674,-9.57585180276088));
#10175=CARTESIAN_POINT('Ctrl Pts',(10.0502525316942,3.06641977252332,-9.53299079371256));
#10176=CARTESIAN_POINT('Ctrl Pts',(10.0502525316942,3.02056794696251,-9.4896066485377));
#10177=CARTESIAN_POINT('Ctrl Pts',(10.0502525316942,2.97698682564639,-9.44503212038191));
#10178=CARTESIAN_POINT('Ctrl Pts',(10.0502525316942,2.9361940142505,-9.39901842603143));
#10179=CARTESIAN_POINT('Ctrl Pts',(10.0502525316942,2.8982483626292,-9.35160551556488));
#10180=CARTESIAN_POINT('Ctrl Pts',(10.0502525316942,2.86292873701901,-9.30300690939252));
#10181=CARTESIAN_POINT('Ctrl Pts',(10.0502525316942,2.82990845462794,-9.25349741301079));
#10182=CARTESIAN_POINT('Ctrl Pts',(10.0502525316942,2.79895351207997,-9.20328535602728));
#10183=CARTESIAN_POINT('Ctrl Pts',(10.0502525316942,2.77003209344587,-9.15244173271444));
#10184=CARTESIAN_POINT('Ctrl Pts',(10.0502525316942,2.74322870228394,-9.10095481538197));
#10185=CARTESIAN_POINT('Ctrl Pts',(10.0502525316942,2.71869695754934,-9.04875963323664));
#10186=CARTESIAN_POINT('Ctrl Pts',(10.0502525316942,2.69660154669561,-8.99577459934956));
#10187=CARTESIAN_POINT('Ctrl Pts',(10.0502525316942,2.67705351804929,-8.94194140034058));
#10188=CARTESIAN_POINT('Ctrl Pts',(10.0502525316942,2.66010336866474,-8.88723149748883));
#10189=CARTESIAN_POINT('Ctrl Pts',(10.0502525316942,2.64863401651716,-8.84275317038967));
#10190=CARTESIAN_POINT('Ctrl Pts',(10.0502525316942,2.64120584766726,-8.8089947353088));
#10191=CARTESIAN_POINT('Ctrl Pts',(10.0502525316942,2.63677452882417,-8.78631177678628));
#10192=CARTESIAN_POINT('Ctrl Pts',(10.0502525316942,2.63468906623289,-8.77492596468499));
#10193=CARTESIAN_POINT('',(10.0502525316942,1.47863151154858,-9.041822881172));
#10194=CARTESIAN_POINT('Origin',(10.0502525316942,0.,0.));
#10195=CARTESIAN_POINT('',(10.0502525316942,1.03854944428814,-10.7106795892491));
#10196=CARTESIAN_POINT('Ctrl Pts',(10.0502525316942,1.47863151154858,-9.041822881172));
#10197=CARTESIAN_POINT('Ctrl Pts',(10.0502525316942,1.48142903122265,-9.05241341063017));
#10198=CARTESIAN_POINT('Ctrl Pts',(10.0502525316942,1.48681431784179,-9.0736287027809));
#10199=CARTESIAN_POINT('Ctrl Pts',(10.0502525316942,1.49426299078246,-9.10555434079238));
#10200=CARTESIAN_POINT('Ctrl Pts',(10.0502525316942,1.50293375169959,-9.14832762892595));
#10201=CARTESIAN_POINT('Ctrl Pts',(10.0502525316942,1.51165206039235,-9.20213819442161));
#10202=CARTESIAN_POINT('Ctrl Pts',(10.0502525316942,1.51821671513724,-9.25629193365179));
#10203=CARTESIAN_POINT('Ctrl Pts',(10.0502525316942,1.52257856936539,-9.31078441132333));
#10204=CARTESIAN_POINT('Ctrl Pts',(10.0502525316942,1.52467115182437,-9.36560546949212));
#10205=CARTESIAN_POINT('Ctrl Pts',(10.0502525316942,1.52441199543777,-9.42073743324162));
#10206=CARTESIAN_POINT('Ctrl Pts',(10.0502525316942,1.52172656066024,-9.47615638983506));
#10207=CARTESIAN_POINT('Ctrl Pts',(10.0502525316942,1.51657146095807,-9.53183308717807));
#10208=CARTESIAN_POINT('Ctrl Pts',(10.0502525316942,1.50895693238989,-9.58773391775221));
#10209=CARTESIAN_POINT('Ctrl Pts',(10.0502525316942,1.49897455623114,-9.64382166809154));
#10210=CARTESIAN_POINT('Ctrl Pts',(10.0502525316942,1.48681164197681,-9.70005659890418));
#10211=CARTESIAN_POINT('Ctrl Pts',(10.0502525316942,1.472706711821,-9.75639893594512));
#10212=CARTESIAN_POINT('Ctrl Pts',(10.0502525316942,1.45691330418438,-9.81281120439258));
#10213=CARTESIAN_POINT('Ctrl Pts',(10.0502525316942,1.43966301743384,-9.86926046040473));
#10214=CARTESIAN_POINT('Ctrl Pts',(10.0502525316942,1.4211247852801,-9.9257209332579));
#10215=CARTESIAN_POINT('Ctrl Pts',(10.0502525316942,1.40137929597453,-9.98217543513636));
#10216=CARTESIAN_POINT('Ctrl Pts',(10.0502525316942,1.38044913636064,-10.0386123354999));
#10217=CARTESIAN_POINT('Ctrl Pts',(10.0502525316942,1.3583201853205,-10.0950232336429));
#10218=CARTESIAN_POINT('Ctrl Pts',(10.0502525316942,1.33496549883664,-10.1514004985561));
#10219=CARTESIAN_POINT('Ctrl Pts',(10.0502525316942,1.31037031610781,-10.2077346253654));
#10220=CARTESIAN_POINT('Ctrl Pts',(10.0502525316942,1.2845505698718,-10.26401245069));
#10221=CARTESIAN_POINT('Ctrl Pts',(10.0502525316942,1.2575411104082,-10.3202191159745));
#10222=CARTESIAN_POINT('Ctrl Pts',(10.0502525316942,1.22938873407214,-10.3763394931394));
#10223=CARTESIAN_POINT('Ctrl Pts',(10.0502525316942,1.20014382966931,-10.4323597856746));
#10224=CARTESIAN_POINT('Ctrl Pts',(10.0502525316942,1.16985259538408,-10.4882691830915));
#10225=CARTESIAN_POINT('Ctrl Pts',(10.0502525316942,1.13855017696687,-10.5440612301269));
#10226=CARTESIAN_POINT('Ctrl Pts',(10.0502525316942,1.10626216443499,-10.599732595958));
#10227=CARTESIAN_POINT('Ctrl Pts',(10.0502525316942,1.07965669109989,-10.6441722372873));
#10228=CARTESIAN_POINT('Ctrl Pts',(10.0502525316942,1.05927071468098,-10.6774471807436));
#10229=CARTESIAN_POINT('Ctrl Pts',(10.0502525316942,1.04548846715806,-10.6996061707058));
#10230=CARTESIAN_POINT('Ctrl Pts',(10.0502525316942,1.03854944428814,-10.7106795892491));
#10231=CARTESIAN_POINT('',(10.0502525316942,-0.205863042617262,-9.15961421508102));
#10232=CARTESIAN_POINT('Ctrl Pts',(10.0502525316942,1.03854944428814,-10.7106795892491));
#10233=CARTESIAN_POINT('Ctrl Pts',(10.0502525316942,1.00031843628634,-10.7069087245865));
#10234=CARTESIAN_POINT('Ctrl Pts',(10.0502525316942,0.926048534485517,-10.6988602462966));
#10235=CARTESIAN_POINT('Ctrl Pts',(10.0502525316942,0.821220046750494,-10.6852672767501));
#10236=CARTESIAN_POINT('Ctrl Pts',(10.0502525316942,0.694625083433483,-10.6640973524763));
#10237=CARTESIAN_POINT('Ctrl Pts',(10.0502525316942,0.558333537570359,-10.6325607057952));
#10238=CARTESIAN_POINT('Ctrl Pts',(10.0502525316942,0.443722777305704,-10.596013814283));
#10239=CARTESIAN_POINT('Ctrl Pts',(10.0502525316942,0.35006979143776,-10.5546263356355));
#10240=CARTESIAN_POINT('Ctrl Pts',(10.0502525316942,0.275979784341795,-10.5087249476599));
#10241=CARTESIAN_POINT('Ctrl Pts',(10.0502525316942,0.219218698708486,-10.4588324224655));
#10242=CARTESIAN_POINT('Ctrl Pts',(10.0502525316942,0.176389733643621,-10.4057430679645));
#10243=CARTESIAN_POINT('Ctrl Pts',(10.0502525316942,0.143293435954743,-10.3504388022425));
#10244=CARTESIAN_POINT('Ctrl Pts',(10.0502525316942,0.1156151003885,-10.2939289512549));
#10245=CARTESIAN_POINT('Ctrl Pts',(10.0502525316942,0.0895255103702553,
-10.237110176256));
#10246=CARTESIAN_POINT('Ctrl Pts',(10.0502525316942,0.0622734430034751,
-10.1806284708027));
#10247=CARTESIAN_POINT('Ctrl Pts',(10.0502525316942,0.0329060076605428,
-10.1247109492303));
#10248=CARTESIAN_POINT('Ctrl Pts',(10.0502525316942,0.00188374052503669,
-10.0692584999061));
#10249=CARTESIAN_POINT('Ctrl Pts',(10.0502525316942,-0.0295176561224928,
-10.0139888357391));
#10250=CARTESIAN_POINT('Ctrl Pts',(10.0502525316942,-0.05971889546067,-9.95855906844526));
#10251=CARTESIAN_POINT('Ctrl Pts',(10.0502525316942,-0.0873927181594365,
-9.90269886586131));
#10252=CARTESIAN_POINT('Ctrl Pts',(10.0502525316942,-0.111969973727219,
-9.84633157004081));
#10253=CARTESIAN_POINT('Ctrl Pts',(10.0502525316942,-0.133407037879776,
-9.78951336137147));
#10254=CARTESIAN_POINT('Ctrl Pts',(10.0502525316942,-0.151980202759258,
-9.73237897573987));
#10255=CARTESIAN_POINT('Ctrl Pts',(10.0502525316942,-0.168085081732297,
-9.67508881816964));
#10256=CARTESIAN_POINT('Ctrl Pts',(10.0502525316942,-0.182008602623654,
-9.61776871087166));
#10257=CARTESIAN_POINT('Ctrl Pts',(10.0502525316942,-0.193802962616849,
-9.56047634174856));
#10258=CARTESIAN_POINT('Ctrl Pts',(10.0502525316942,-0.203384169996506,
-9.50322667013965));
#10259=CARTESIAN_POINT('Ctrl Pts',(10.0502525316942,-0.210586047375027,
-9.44600537601646));
#10260=CARTESIAN_POINT('Ctrl Pts',(10.0502525316942,-0.215226755929045,
-9.38878575682053));
#10261=CARTESIAN_POINT('Ctrl Pts',(10.0502525316942,-0.21718266259851,-9.33154666905179));
#10262=CARTESIAN_POINT('Ctrl Pts',(10.0502525316942,-0.216396922881075,
-9.27427657522174));
#10263=CARTESIAN_POINT('Ctrl Pts',(10.0502525316942,-0.2135603660237,-9.2284309476721));
#10264=CARTESIAN_POINT('Ctrl Pts',(10.0502525316942,-0.210193044269049,
-9.1940293375968));
#10265=CARTESIAN_POINT('Ctrl Pts',(10.0502525316942,-0.207398059264384,
-9.1710872092551));
#10266=CARTESIAN_POINT('Ctrl Pts',(10.0502525316942,-0.205863042617262,
-9.15961421508102));
#10267=CARTESIAN_POINT('',(10.0502525316942,-1.38781479615277,-9.05620683581208));
#10268=CARTESIAN_POINT('Origin',(10.0502525316942,0.,0.));
#10269=CARTESIAN_POINT('',(10.0502525316942,-2.32206279789789,-10.5073910450885));
#10270=CARTESIAN_POINT('Ctrl Pts',(10.0502525316942,-1.38781479615277,-9.05620683581208));
#10271=CARTESIAN_POINT('Ctrl Pts',(10.0502525316942,-1.38842685041928,-9.06714350898568));
#10272=CARTESIAN_POINT('Ctrl Pts',(10.0502525316942,-1.38986102430324,-9.08898459591562));
#10273=CARTESIAN_POINT('Ctrl Pts',(10.0502525316942,-1.39264248006707,-9.12164944850753));
#10274=CARTESIAN_POINT('Ctrl Pts',(10.0502525316942,-1.39761376933417,-9.16500867538789));
#10275=CARTESIAN_POINT('Ctrl Pts',(10.0502525316942,-1.40595054425593,-9.21887966989633));
#10276=CARTESIAN_POINT('Ctrl Pts',(10.0502525316942,-1.41644161231465,-9.27241152635132));
#10277=CARTESIAN_POINT('Ctrl Pts',(10.0502525316942,-1.42913234409394,-9.32558483941339));
#10278=CARTESIAN_POINT('Ctrl Pts',(10.0502525316942,-1.44408281853422,-9.37836940755697));
#10279=CARTESIAN_POINT('Ctrl Pts',(10.0502525316942,-1.4613660046363,-9.43072293720942));
#10280=CARTESIAN_POINT('Ctrl Pts',(10.0502525316942,-1.48104540427845,-9.48259965202034));
#10281=CARTESIAN_POINT('Ctrl Pts',(10.0502525316942,-1.50315324111201,-9.53395832441854));
#10282=CARTESIAN_POINT('Ctrl Pts',(10.0502525316942,-1.52766939477237,-9.58477015487067));
#10283=CARTESIAN_POINT('Ctrl Pts',(10.0502525316942,-1.55449526669738,-9.63502805143792));
#10284=CARTESIAN_POINT('Ctrl Pts',(10.0502525316942,-1.5834404348547,-9.68475210162498));
#10285=CARTESIAN_POINT('Ctrl Pts',(10.0502525316942,-1.61426576023972,-9.73397818528844));
#10286=CARTESIAN_POINT('Ctrl Pts',(10.0502525316942,-1.64671853312854,-9.78274900943559));
#10287=CARTESIAN_POINT('Ctrl Pts',(10.0502525316942,-1.68056831017818,-9.8311048104422));
#10288=CARTESIAN_POINT('Ctrl Pts',(10.0502525316942,-1.71564646229066,-9.87907328228114));
#10289=CARTESIAN_POINT('Ctrl Pts',(10.0502525316942,-1.75187093905158,-9.92666301240917));
#10290=CARTESIAN_POINT('Ctrl Pts',(10.0502525316942,-1.78921666506164,-9.97386991924375));
#10291=CARTESIAN_POINT('Ctrl Pts',(10.0502525316942,-1.8276944743413,-10.0206816495736));
#10292=CARTESIAN_POINT('Ctrl Pts',(10.0502525316942,-1.86732763406234,-10.0670826197184));
#10293=CARTESIAN_POINT('Ctrl Pts',(10.0502525316942,-1.9081272454134,-10.1130592286672));
#10294=CARTESIAN_POINT('Ctrl Pts',(10.0502525316942,-1.95007408775204,-10.1586038807877));
#10295=CARTESIAN_POINT('Ctrl Pts',(10.0502525316942,-1.99313042494654,-10.2037132140826));
#10296=CARTESIAN_POINT('Ctrl Pts',(10.0502525316942,-2.03724707618484,-10.2483873017624));
#10297=CARTESIAN_POINT('Ctrl Pts',(10.0502525316942,-2.08237185550883,-10.2926285935634));
#10298=CARTESIAN_POINT('Ctrl Pts',(10.0502525316942,-2.12845748520948,-10.3364410841241));
#10299=CARTESIAN_POINT('Ctrl Pts',(10.0502525316942,-2.17546854490588,-10.3798294947586));
#10300=CARTESIAN_POINT('Ctrl Pts',(10.0502525316942,-2.22337966776441,-10.4227985654164));
#10301=CARTESIAN_POINT('Ctrl Pts',(10.0502525316942,-2.26241558094358,-10.4568416324806));
#10302=CARTESIAN_POINT('Ctrl Pts',(10.0502525316942,-2.29208631967267,-10.4821883711236));
#10303=CARTESIAN_POINT('Ctrl Pts',(10.0502525316942,-2.31204152046505,-10.4990038742164));
#10304=CARTESIAN_POINT('Ctrl Pts',(10.0502525316942,-2.32206279789789,-10.5073910450885));
#10305=CARTESIAN_POINT('',(10.0502525316942,-3.02626384252387,-8.64769560732005));
#10306=CARTESIAN_POINT('Ctrl Pts',(10.0502525316942,-2.32206279789789,-10.5073910450885));
#10307=CARTESIAN_POINT('Ctrl Pts',(10.0502525316942,-2.35725738591831,-10.4919907084944));
#10308=CARTESIAN_POINT('Ctrl Pts',(10.0502525316942,-2.42540514342016,-10.4613854889436));
#10309=CARTESIAN_POINT('Ctrl Pts',(10.0502525316942,-2.52090250118004,-10.4160640224759));
#10310=CARTESIAN_POINT('Ctrl Pts',(10.0502525316942,-2.63475959960258,-10.3568102329785));
#10311=CARTESIAN_POINT('Ctrl Pts',(10.0502525316942,-2.75463520264158,-10.284700695789));
#10312=CARTESIAN_POINT('Ctrl Pts',(10.0502525316942,-2.85234290245999,-10.214525863806));
#10313=CARTESIAN_POINT('Ctrl Pts',(10.0502525316942,-2.92862275068379,-10.1462236683382));
#10314=CARTESIAN_POINT('Ctrl Pts',(10.0502525316942,-2.98490222577489,-10.0796737828909));
#10315=CARTESIAN_POINT('Ctrl Pts',(10.0502525316942,-3.02346758796109,-10.0146830316105));
#10316=CARTESIAN_POINT('Ctrl Pts',(10.0502525316942,-3.04779484151101,-9.95095717700994));
#10317=CARTESIAN_POINT('Ctrl Pts',(10.0502525316942,-3.06218133312374,-9.88813237627935));
#10318=CARTESIAN_POINT('Ctrl Pts',(10.0502525316942,-3.07104249021943,-9.82583523819669));
#10319=CARTESIAN_POINT('Ctrl Pts',(10.0502525316942,-3.07829719773955,-9.76373524529424));
#10320=CARTESIAN_POINT('Ctrl Pts',(10.0502525316942,-3.08676164713489,-9.70159659932322));
#10321=CARTESIAN_POINT('Ctrl Pts',(10.0502525316942,-3.09741227343545,-9.6393408394545));
#10322=CARTESIAN_POINT('Ctrl Pts',(10.0502525316942,-3.10978045352404,-9.57701601843134));
#10323=CARTESIAN_POINT('Ctrl Pts',(10.0502525316942,-3.12256569092543,-9.51474787896063));
#10324=CARTESIAN_POINT('Ctrl Pts',(10.0502525316942,-3.13416003631015,-9.45269834137241));
#10325=CARTESIAN_POINT('Ctrl Pts',(10.0502525316942,-3.14321765381094,-9.39102045019014));
#10326=CARTESIAN_POINT('Ctrl Pts',(10.0502525316942,-3.14917356053584,-9.32981717654858));
#10327=CARTESIAN_POINT('Ctrl Pts',(10.0502525316942,-3.15200362801959,-9.26915543181673));
#10328=CARTESIAN_POINT('Ctrl Pts',(10.0502525316942,-3.15201226138312,-9.2090779784702));
#10329=CARTESIAN_POINT('Ctrl Pts',(10.0502525316942,-3.14962527917495,-9.14961511949843));
#10330=CARTESIAN_POINT('Ctrl Pts',(10.0502525316942,-3.14515444717397,-9.09079785336098));
#10331=CARTESIAN_POINT('Ctrl Pts',(10.0502525316942,-3.13866723439399,-9.0326649146968));
#10332=CARTESIAN_POINT('Ctrl Pts',(10.0502525316942,-3.13008838265685,-8.97525648555044));
#10333=CARTESIAN_POINT('Ctrl Pts',(10.0502525316942,-3.11925542274306,-8.91861029840238));
#10334=CARTESIAN_POINT('Ctrl Pts',(10.0502525316942,-3.10598716411038,-8.86275714889703));
#10335=CARTESIAN_POINT('Ctrl Pts',(10.0502525316942,-3.09015949103058,-8.8077151330875));
#10336=CARTESIAN_POINT('Ctrl Pts',(10.0502525316942,-3.07171477588927,-8.75349084408744));
#10337=CARTESIAN_POINT('Ctrl Pts',(10.0502525316942,-3.0548499719756,-8.71076560553715));
#10338=CARTESIAN_POINT('Ctrl Pts',(10.0502525316942,-3.04101677653125,-8.67908828975171));
#10339=CARTESIAN_POINT('Ctrl Pts',(10.0502525316942,-3.0312690802849,-8.65813272696012));
#10340=CARTESIAN_POINT('Ctrl Pts',(10.0502525316942,-3.02626384252387,-8.64769560732005));
#10341=CARTESIAN_POINT('',(10.0502525316942,-4.11841212213242,-8.18410616705958));
#10342=CARTESIAN_POINT('Origin',(10.0502525316942,0.,0.));
#10343=CARTESIAN_POINT('',(10.0502525316942,-5.45537535466284,-9.2755658561365));
#10344=CARTESIAN_POINT('Ctrl Pts',(10.0502525316942,-4.11841212213242,-8.18410616705958));
#10345=CARTESIAN_POINT('Ctrl Pts',(10.0502525316942,-4.12237383820348,-8.19431842617809));
#10346=CARTESIAN_POINT('Ctrl Pts',(10.0502525316942,-4.1304870856583,-8.21464735012275));
#10347=CARTESIAN_POINT('Ctrl Pts',(10.0502525316942,-4.14322640185693,-8.24485395393399));
#10348=CARTESIAN_POINT('Ctrl Pts',(10.0502525316942,-4.16135311687778,-8.28455481633258));
#10349=CARTESIAN_POINT('Ctrl Pts',(10.0502525316942,-4.18592891379899,-8.33321297157003));
#10350=CARTESIAN_POINT('Ctrl Pts',(10.0502525316942,-4.21244876582417,-8.38088287416164));
#10351=CARTESIAN_POINT('Ctrl Pts',(10.0502525316942,-4.24094982636281,-8.42753204825146));
#10352=CARTESIAN_POINT('Ctrl Pts',(10.0502525316942,-4.27147990109805,-8.47311320506822));
#10353=CARTESIAN_POINT('Ctrl Pts',(10.0502525316942,-4.3040953182409,-8.51756357237276));
#10354=CARTESIAN_POINT('Ctrl Pts',(10.0502525316942,-4.33884232599626,-8.56081999110915));
#10355=CARTESIAN_POINT('Ctrl Pts',(10.0502525316942,-4.37573883085758,-8.60283329387128));
#10356=CARTESIAN_POINT('Ctrl Pts',(10.0502525316942,-4.41475679767577,-8.6435823082099));
#10357=CARTESIAN_POINT('Ctrl Pts',(10.0502525316942,-4.45580026211617,-8.68309075792173));
#10358=CARTESIAN_POINT('Ctrl Pts',(10.0502525316942,-4.4986943294444,-8.72143659100306));
#10359=CARTESIAN_POINT('Ctrl Pts',(10.0502525316942,-4.54322265243728,-8.75872782924178));
#10360=CARTESIAN_POINT('Ctrl Pts',(10.0502525316942,-4.58915808705618,-8.79508318101477));
#10361=CARTESIAN_POINT('Ctrl Pts',(10.0502525316942,-4.63629390238203,-8.83061212429863));
#10362=CARTESIAN_POINT('Ctrl Pts',(10.0502525316942,-4.68447828052063,-8.86539310688376));
#10363=CARTESIAN_POINT('Ctrl Pts',(10.0502525316942,-4.73363584056076,-8.89945965089929));
#10364=CARTESIAN_POINT('Ctrl Pts',(10.0502525316942,-4.78374147310216,-8.93281562325407));
#10365=CARTESIAN_POINT('Ctrl Pts',(10.0502525316942,-4.83480166455838,-8.96544592744964));
#10366=CARTESIAN_POINT('Ctrl Pts',(10.0502525316942,-4.88683372770265,-8.99732855257362));
#10367=CARTESIAN_POINT('Ctrl Pts',(10.0502525316942,-4.93984401744929,-9.02844713284016));
#10368=CARTESIAN_POINT('Ctrl Pts',(10.0502525316942,-4.99381190670161,-9.05880038387882));
#10369=CARTESIAN_POINT('Ctrl Pts',(10.0502525316942,-5.04870046735128,-9.08839676934597));
#10370=CARTESIAN_POINT('Ctrl Pts',(10.0502525316942,-5.10446294828982,-9.11725155657582));
#10371=CARTESIAN_POINT('Ctrl Pts',(10.0502525316942,-5.16105047473192,-9.14538320175401));
#10372=CARTESIAN_POINT('Ctrl Pts',(10.0502525316942,-5.21841931731543,-9.17281011362288));
#10373=CARTESIAN_POINT('Ctrl Pts',(10.0502525316942,-5.27653724822262,-9.19954772791879));
#10374=CARTESIAN_POINT('Ctrl Pts',(10.0502525316942,-5.33538160688598,-9.2256083913841));
#10375=CARTESIAN_POINT('Ctrl Pts',(10.0502525316942,-5.38302685274804,-9.24592251158686));
#10376=CARTESIAN_POINT('Ctrl Pts',(10.0502525316942,-5.41907797515233,-9.26085993003723));
#10377=CARTESIAN_POINT('Ctrl Pts',(10.0502525316942,-5.44325277512453,-9.27068592765741));
#10378=CARTESIAN_POINT('Ctrl Pts',(10.0502525316942,-5.45537535466284,-9.2755658561365));
#10379=CARTESIAN_POINT('',(10.0502525316942,-5.55043285230422,-7.28928030147641));
#10380=CARTESIAN_POINT('Ctrl Pts',(10.0502525316942,-5.45537535466284,-9.2755658561365));
#10381=CARTESIAN_POINT('Ctrl Pts',(10.0502525316942,-5.48408843121132,-9.25004353985722));
#10382=CARTESIAN_POINT('Ctrl Pts',(10.0502525316942,-5.53944326709657,-9.19987743117415));
#10383=CARTESIAN_POINT('Ctrl Pts',(10.0502525316942,-5.61626154813455,-9.12726384869626));
#10384=CARTESIAN_POINT('Ctrl Pts',(10.0502525316942,-5.70623565557996,-9.03572636773682));
#10385=CARTESIAN_POINT('Ctrl Pts',(10.0502525316942,-5.79796105654696,-8.93010252395574));
#10386=CARTESIAN_POINT('Ctrl Pts',(10.0502525316942,-5.86920138549131,-8.83316895299322));
#10387=CARTESIAN_POINT('Ctrl Pts',(10.0502525316942,-5.92064129305387,-8.74463793548674));
#10388=CARTESIAN_POINT('Ctrl Pts',(10.0502525316942,-5.95360120899603,-8.6639539190358));
#10389=CARTESIAN_POINT('Ctrl Pts',(10.0502525316942,-5.97019580138365,-8.59022668922188));
#10390=CARTESIAN_POINT('Ctrl Pts',(10.0502525316942,-5.97364002234323,-8.52210226517413));
#10391=CARTESIAN_POINT('Ctrl Pts',(10.0502525316942,-5.96790845784416,-8.45790665865659));
#10392=CARTESIAN_POINT('Ctrl Pts',(10.0502525316942,-5.95708504467347,-8.39592031140414));
#10393=CARTESIAN_POINT('Ctrl Pts',(10.0502525316942,-5.94479472837688,-8.33461788057945));
#10394=CARTESIAN_POINT('Ctrl Pts',(10.0502525316942,-5.93364300051867,-8.27290485770376));
#10395=CARTESIAN_POINT('Ctrl Pts',(10.0502525316942,-5.92453426026728,-8.2104048870761));
#10396=CARTESIAN_POINT('Ctrl Pts',(10.0502525316942,-5.91703766966772,-8.14730848207823));
#10397=CARTESIAN_POINT('Ctrl Pts',(10.0502525316942,-5.90995523970613,-8.08413710664289));
#10398=CARTESIAN_POINT('Ctrl Pts',(10.0502525316942,-5.90180775582857,-8.02154163982398));
#10399=CARTESIAN_POINT('Ctrl Pts',(10.0502525316942,-5.89136254542228,-7.96008352176745));
#10400=CARTESIAN_POINT('Ctrl Pts',(10.0502525316942,-5.87811409765682,-7.90003527315714));
#10401=CARTESIAN_POINT('Ctrl Pts',(10.0502525316942,-5.86206014174823,-7.84146798659238));
#10402=CARTESIAN_POINT('Ctrl Pts',(10.0502525316942,-5.84350339850201,-7.78432826524869));
#10403=CARTESIAN_POINT('Ctrl Pts',(10.0502525316942,-5.82285820956226,-7.72851334381364));
#10404=CARTESIAN_POINT('Ctrl Pts',(10.0502525316942,-5.80043066085532,-7.67395636265026));
#10405=CARTESIAN_POINT('Ctrl Pts',(10.0502525316942,-5.77629688888814,-7.62067331151744));
#10406=CARTESIAN_POINT('Ctrl Pts',(10.0502525316942,-5.75039773581461,-7.56872566186653));
#10407=CARTESIAN_POINT('Ctrl Pts',(10.0502525316942,-5.72259034420254,-7.51819950516883));
#10408=CARTESIAN_POINT('Ctrl Pts',(10.0502525316942,-5.69271190798352,-7.46918012077942));
#10409=CARTESIAN_POINT('Ctrl Pts',(10.0502525316942,-5.66064997807339,-7.42172307293681));
#10410=CARTESIAN_POINT('Ctrl Pts',(10.0502525316942,-5.62635178473812,-7.37585243997691));
#10411=CARTESIAN_POINT('Ctrl Pts',(10.0502525316942,-5.59710957827922,-7.34042983445952));
#10412=CARTESIAN_POINT('Ctrl Pts',(10.0502525316942,-5.5741645986968,-7.31457760934185));
#10413=CARTESIAN_POINT('Ctrl Pts',(10.0502525316942,-5.55841836363355,-7.2976598885924));
#10414=CARTESIAN_POINT('Ctrl Pts',(10.0502525316942,-5.55043285230422,-7.28928030147641));
#10415=CARTESIAN_POINT('',(10.0502525316942,-6.44587057493322,-6.51088816465466));
#10416=CARTESIAN_POINT('Origin',(10.0502525316942,0.,0.));
#10417=CARTESIAN_POINT('',(10.0502525316942,-8.05467776187827,-7.13578365451838));
#10418=CARTESIAN_POINT('Ctrl Pts',(10.0502525316942,-6.44587057493322,-6.51088816465466));
#10419=CARTESIAN_POINT('Ctrl Pts',(10.0502525316942,-6.45279415243689,-6.51937636264257));
#10420=CARTESIAN_POINT('Ctrl Pts',(10.0502525316942,-6.46679229227336,-6.5362031868863));
#10421=CARTESIAN_POINT('Ctrl Pts',(10.0502525316942,-6.48824245587723,-6.56099470907402));
#10422=CARTESIAN_POINT('Ctrl Pts',(10.0502525316942,-6.51775022748935,-6.59315100996711));
#10423=CARTESIAN_POINT('Ctrl Pts',(10.0502525316942,-6.55615939617772,-6.63183332667763));
#10424=CARTESIAN_POINT('Ctrl Pts',(10.0502525316942,-6.59611208427845,-6.66897501320444));
#10425=CARTESIAN_POINT('Ctrl Pts',(10.0502525316942,-6.63763359119236,-6.70453370213821));
#10426=CARTESIAN_POINT('Ctrl Pts',(10.0502525316942,-6.68075476979194,-6.73844964641633));
#10427=CARTESIAN_POINT('Ctrl Pts',(10.0502525316942,-6.72550979370064,-6.77064573971725));
#10428=CARTESIAN_POINT('Ctrl Pts',(10.0502525316942,-6.77192313035347,-6.801047622728));
#10429=CARTESIAN_POINT('Ctrl Pts',(10.0502525316942,-6.81999661627367,-6.82960300105583));
#10430=CARTESIAN_POINT('Ctrl Pts',(10.0502525316942,-6.86969704580336,-6.8563004018424));
#10431=CARTESIAN_POINT('Ctrl Pts',(10.0502525316942,-6.92094048249309,-6.88119204236944));
#10432=CARTESIAN_POINT('Ctrl Pts',(10.0502525316942,-6.97358467882161,-6.90440610103192));
#10433=CARTESIAN_POINT('Ctrl Pts',(10.0502525316942,-7.02745725692073,-6.92611216762375));
#10434=CARTESIAN_POINT('Ctrl Pts',(10.0502525316942,-7.08237887287821,-6.94649333188842));
#10435=CARTESIAN_POINT('Ctrl Pts',(10.0502525316942,-7.13818674446165,-6.96571759693621));
#10436=CARTESIAN_POINT('Ctrl Pts',(10.0502525316942,-7.19476072597386,-6.98390648535874));
#10437=CARTESIAN_POINT('Ctrl Pts',(10.0502525316942,-7.25203948481561,-7.00111517257795));
#10438=CARTESIAN_POINT('Ctrl Pts',(10.0502525316942,-7.31000033546873,-7.01735509547412));
#10439=CARTESIAN_POINT('Ctrl Pts',(10.0502525316942,-7.36864478180451,-7.032609892012));
#10440=CARTESIAN_POINT('Ctrl Pts',(10.0502525316942,-7.42798248750274,-7.0468532786288));
#10441=CARTESIAN_POINT('Ctrl Pts',(10.0502525316942,-7.48801443914016,-7.06006772676068));
#10442=CARTESIAN_POINT('Ctrl Pts',(10.0502525316942,-7.54872062228975,-7.07225838902223));
#10443=CARTESIAN_POINT('Ctrl Pts',(10.0502525316942,-7.6100685316471,-7.08344472624203));
#10444=CARTESIAN_POINT('Ctrl Pts',(10.0502525316942,-7.67201842213158,-7.09365570540476));
#10445=CARTESIAN_POINT('Ctrl Pts',(10.0502525316942,-7.73452951433514,-7.10292398252533));
#10446=CARTESIAN_POINT('Ctrl Pts',(10.0502525316942,-7.79756590777721,-7.11128057847415));
#10447=CARTESIAN_POINT('Ctrl Pts',(10.0502525316942,-7.86110172188657,-7.11875013245223));
#10448=CARTESIAN_POINT('Ctrl Pts',(10.0502525316942,-7.92511922053603,-7.12535138940982));
#10449=CARTESIAN_POINT('Ctrl Pts',(10.0502525316942,-7.97670995045205,-7.12994807512891));
#10450=CARTESIAN_POINT('Ctrl Pts',(10.0502525316942,-8.01561252148766,-7.13301399479354));
#10451=CARTESIAN_POINT('Ctrl Pts',(10.0502525316942,-8.04164052278268,-7.13488864983229));
#10452=CARTESIAN_POINT('Ctrl Pts',(10.0502525316942,-8.05467776187827,-7.13578365451838));
#10453=CARTESIAN_POINT('',(10.0502525316942,-7.53128682236137,-5.21733945232202));
#10454=CARTESIAN_POINT('Ctrl Pts',(10.0502525316942,-8.05467776187827,-7.13578365451838));
#10455=CARTESIAN_POINT('Ctrl Pts',(10.0502525316942,-8.07409869096647,-7.10263766069576));
#10456=CARTESIAN_POINT('Ctrl Pts',(10.0502525316942,-8.11124208821886,-7.03782127112617));
#10457=CARTESIAN_POINT('Ctrl Pts',(10.0502525316942,-8.16186178396251,-6.94502349601963));
#10458=CARTESIAN_POINT('Ctrl Pts',(10.0502525316942,-8.21914560790757,-6.83016265001357));
#10459=CARTESIAN_POINT('Ctrl Pts',(10.0502525316942,-8.27374208546745,-6.70136369739477));
#10460=CARTESIAN_POINT('Ctrl Pts',(10.0502525316942,-8.31154154378012,-6.58715992075444));
#10461=CARTESIAN_POINT('Ctrl Pts',(10.0502525316942,-8.33310621412631,-6.48706611403476));
#10462=CARTESIAN_POINT('Ctrl Pts',(10.0502525316942,-8.33952022470187,-6.40014588026893));
#10463=CARTESIAN_POINT('Ctrl Pts',(10.0502525316942,-8.33251965296669,-6.32489910686351));
#10464=CARTESIAN_POINT('Ctrl Pts',(10.0502525316942,-8.31474369699109,-6.25904460664515));
#10465=CARTESIAN_POINT('Ctrl Pts',(10.0502525316942,-8.28945512184757,-6.19976210758369));
#10466=CARTESIAN_POINT('Ctrl Pts',(10.0502525316942,-8.26000660950279,-6.1441542067148));
#10467=CARTESIAN_POINT('Ctrl Pts',(10.0502525316942,-8.22937433118026,-6.08965004701613));
#10468=CARTESIAN_POINT('Ctrl Pts',(10.0502525316942,-8.19969803488993,-6.03440354789477));
#10469=CARTESIAN_POINT('Ctrl Pts',(10.0502525316942,-8.17172155504672,-5.9777772990961));
#10470=CARTESIAN_POINT('Ctrl Pts',(10.0502525316942,-8.1450940122787,-5.92008562586321));
#10471=CARTESIAN_POINT('Ctrl Pts',(10.0502525316942,-8.11883719254497,-5.86219466883171));
#10472=CARTESIAN_POINT('Ctrl Pts',(10.0502525316942,-8.09174541189394,-5.80518055320261));
#10473=CARTESIAN_POINT('Ctrl Pts',(10.0502525316942,-8.06281982355119,-5.74995815707108));
#10474=CARTESIAN_POINT('Ctrl Pts',(10.0502525316942,-8.03166387167001,-5.69694287444675));
#10475=CARTESIAN_POINT('Ctrl Pts',(10.0502525316942,-7.99829736542789,-5.64620302012031));
#10476=CARTESIAN_POINT('Ctrl Pts',(10.0502525316942,-7.96299170889331,-5.59759426482043));
#10477=CARTESIAN_POINT('Ctrl Pts',(10.0502525316942,-7.92610920815888,-5.5508908343176));
#10478=CARTESIAN_POINT('Ctrl Pts',(10.0502525316942,-7.88792030747535,-5.50593455556538));
#10479=CARTESIAN_POINT('Ctrl Pts',(10.0502525316942,-7.84850235807098,-5.46271710825366));
#10480=CARTESIAN_POINT('Ctrl Pts',(10.0502525316942,-7.80781809321391,-5.42131523598658));
#10481=CARTESIAN_POINT('Ctrl Pts',(10.0502525316942,-7.76575825114004,-5.38185496199325));
#10482=CARTESIAN_POINT('Ctrl Pts',(10.0502525316942,-7.72219434684711,-5.34446770160195));
#10483=CARTESIAN_POINT('Ctrl Pts',(10.0502525316942,-7.67703660519485,-5.3092410482218));
#10484=CARTESIAN_POINT('Ctrl Pts',(10.0502525316942,-7.63024227979884,-5.27621420845565));
#10485=CARTESIAN_POINT('Ctrl Pts',(10.0502525316942,-7.59148510170534,-5.25156164740301));
#10486=CARTESIAN_POINT('Ctrl Pts',(10.0502525316942,-7.56167435245346,-5.23406510887067));
#10487=CARTESIAN_POINT('Ctrl Pts',(10.0502525316942,-7.54147092977177,-5.22284125454301));
#10488=CARTESIAN_POINT('Ctrl Pts',(10.0502525316942,-7.53128682236137,-5.21733945232202));
#10489=CARTESIAN_POINT('',(10.0502525316942,-8.14236230483842,-4.20033906466803));
#10490=CARTESIAN_POINT('Origin',(10.0502525316942,0.,0.));
#10491=CARTESIAN_POINT('',(10.0502525316942,-9.86553218952113,-4.29750123086779));
#10492=CARTESIAN_POINT('Ctrl Pts',(10.0502525316942,-8.14236230483842,-4.20033906466803));
#10493=CARTESIAN_POINT('Ctrl Pts',(10.0502525316942,-8.15157001576925,-4.20627231756552));
#10494=CARTESIAN_POINT('Ctrl Pts',(10.0502525316942,-8.17008281252941,-4.21794991531197));
#10495=CARTESIAN_POINT('Ctrl Pts',(10.0502525316942,-8.1981441320729,-4.23489958895176));
#10496=CARTESIAN_POINT('Ctrl Pts',(10.0502525316942,-8.23614453399815,-4.2563636455618));
#10497=CARTESIAN_POINT('Ctrl Pts',(10.0502525316942,-8.28462731741005,-4.28128362907021));
#10498=CARTESIAN_POINT('Ctrl Pts',(10.0502525316942,-8.33410199410829,-4.30426141247364));
#10499=CARTESIAN_POINT('Ctrl Pts',(10.0502525316942,-8.38457953300338,-4.32524888402656));
#10500=CARTESIAN_POINT('Ctrl Pts',(10.0502525316942,-8.43607081406306,-4.34417968683382));
#10501=CARTESIAN_POINT('Ctrl Pts',(10.0502525316942,-8.48858451117083,-4.36096992819547));
#10502=CARTESIAN_POINT('Ctrl Pts',(10.0502525316942,-8.54212091594884,-4.37554132734911));
#10503=CARTESIAN_POINT('Ctrl Pts',(10.0502525316942,-8.59666561517837,-4.38784358185488));
#10504=CARTESIAN_POINT('Ctrl Pts',(10.0502525316942,-8.65218348309394,-4.39787604148868));
#10505=CARTESIAN_POINT('Ctrl Pts',(10.0502525316942,-8.70861082741579,-4.4057143056259));
#10506=CARTESIAN_POINT('Ctrl Pts',(10.0502525316942,-8.76585197201427,-4.41152423606579));
#10507=CARTESIAN_POINT('Ctrl Pts',(10.0502525316942,-8.82379538192297,-4.41552038997767));
#10508=CARTESIAN_POINT('Ctrl Pts',(10.0502525316942,-8.88232706878773,-4.41793231637186));
#10509=CARTESIAN_POINT('Ctrl Pts',(10.0502525316942,-8.94134413332185,-4.41897009817737));
#10510=CARTESIAN_POINT('Ctrl Pts',(10.0502525316942,-9.00076986272314,-4.41878643730905));
#10511=CARTESIAN_POINT('Ctrl Pts',(10.0502525316942,-9.06056297636652,-4.41745276152696));
#10512=CARTESIAN_POINT('Ctrl Pts',(10.0502525316942,-9.12070543323243,-4.41498695816126));
#10513=CARTESIAN_POINT('Ctrl Pts',(10.0502525316942,-9.18119360744053,-4.4113730012699));
#10514=CARTESIAN_POINT('Ctrl Pts',(10.0502525316942,-9.24202856762888,-4.40658290745794));
#10515=CARTESIAN_POINT('Ctrl Pts',(10.0502525316942,-9.3032058354636,-4.40059970120156));
#10516=CARTESIAN_POINT('Ctrl Pts',(10.0502525316942,-9.36470796833893,-4.3934344677265));
#10517=CARTESIAN_POINT('Ctrl Pts',(10.0502525316942,-9.42651006560004,-4.38511576007206));
#10518=CARTESIAN_POINT('Ctrl Pts',(10.0502525316942,-9.48858327871958,-4.37568340938316));
#10519=CARTESIAN_POINT('Ctrl Pts',(10.0502525316942,-9.55089891543934,-4.36518107490567));
#10520=CARTESIAN_POINT('Ctrl Pts',(10.0502525316942,-9.61343241834946,-4.35364935309914));
#10521=CARTESIAN_POINT('Ctrl Pts',(10.0502525316942,-9.67616678749592,-4.34111967477257));
#10522=CARTESIAN_POINT('Ctrl Pts',(10.0502525316942,-9.73909094732754,-4.32761534819777));
#10523=CARTESIAN_POINT('Ctrl Pts',(10.0502525316942,-9.78957710119959,-4.316044643808));
#10524=CARTESIAN_POINT('Ctrl Pts',(10.0502525316942,-9.8275230661634,-4.30693895110861));
#10525=CARTESIAN_POINT('Ctrl Pts',(10.0502525316942,-9.85285646666673,-4.30067875926925));
#10526=CARTESIAN_POINT('Ctrl Pts',(10.0502525316942,-9.86553218952113,-4.29750123086779));
#10527=CARTESIAN_POINT('',(10.0502525316942,-8.77492596468499,-2.63468906623289));
#10528=CARTESIAN_POINT('Ctrl Pts',(10.0502525316942,-9.86553218952113,-4.29750123086779));
#10529=CARTESIAN_POINT('Ctrl Pts',(10.0502525316942,-9.87375991529634,-4.25997612031891));
#10530=CARTESIAN_POINT('Ctrl Pts',(10.0502525316942,-9.88905601939953,-4.18685412967622));
#10531=CARTESIAN_POINT('Ctrl Pts',(10.0502525316942,-9.9085221213413,-4.08295585472858));
#10532=CARTESIAN_POINT('Ctrl Pts',(10.0502525316942,-9.9275083219784,-3.95601502356553));
#10533=CARTESIAN_POINT('Ctrl Pts',(10.0502525316942,-9.93963159251159,-3.81664870098641));
#10534=CARTESIAN_POINT('Ctrl Pts',(10.0502525316942,-9.94029010584861,-3.69635378003033));
#10535=CARTESIAN_POINT('Ctrl Pts',(10.0502525316942,-9.92986863879505,-3.59449506329372));
#10536=CARTESIAN_POINT('Ctrl Pts',(10.0502525316942,-9.90910889595984,-3.50984697030288));
#10537=CARTESIAN_POINT('Ctrl Pts',(10.0502525316942,-9.87919842483915,-3.44044633176199));
#10538=CARTESIAN_POINT('Ctrl Pts',(10.0502525316942,-9.84194232635164,-3.38330805268968));
#10539=CARTESIAN_POINT('Ctrl Pts',(10.0502525316942,-9.79957216249457,-3.3347416451379));
#10540=CARTESIAN_POINT('Ctrl Pts',(10.0502525316942,-9.75438117654386,-3.29095547943263));
#10541=CARTESIAN_POINT('Ctrl Pts',(10.0502525316942,-9.70840543702524,-3.24858483776411));
#10542=CARTESIAN_POINT('Ctrl Pts',(10.0502525316942,-9.66310949495059,-3.20521277465607));
#10543=CARTESIAN_POINT('Ctrl Pts',(10.0502525316942,-9.61900380828622,-3.16000321945708));
#10544=CARTESIAN_POINT('Ctrl Pts',(10.0502525316942,-9.57585180276088,-3.11336354092674));
#10545=CARTESIAN_POINT('Ctrl Pts',(10.0502525316942,-9.53299079371256,-3.06641977252332));
#10546=CARTESIAN_POINT('Ctrl Pts',(10.0502525316942,-9.4896066485377,-3.02056794696251));
#10547=CARTESIAN_POINT('Ctrl Pts',(10.0502525316942,-9.44503212038191,-2.97698682564639));
#10548=CARTESIAN_POINT('Ctrl Pts',(10.0502525316942,-9.39901842603143,-2.9361940142505));
#10549=CARTESIAN_POINT('Ctrl Pts',(10.0502525316942,-9.35160551556488,-2.8982483626292));
#10550=CARTESIAN_POINT('Ctrl Pts',(10.0502525316942,-9.30300690939252,-2.86292873701901));
#10551=CARTESIAN_POINT('Ctrl Pts',(10.0502525316942,-9.25349741301079,-2.82990845462794));
#10552=CARTESIAN_POINT('Ctrl Pts',(10.0502525316942,-9.20328535602728,-2.79895351207997));
#10553=CARTESIAN_POINT('Ctrl Pts',(10.0502525316942,-9.15244173271444,-2.77003209344587));
#10554=CARTESIAN_POINT('Ctrl Pts',(10.0502525316942,-9.10095481538197,-2.74322870228394));
#10555=CARTESIAN_POINT('Ctrl Pts',(10.0502525316942,-9.04875963323664,-2.71869695754934));
#10556=CARTESIAN_POINT('Ctrl Pts',(10.0502525316942,-8.99577459934956,-2.69660154669561));
#10557=CARTESIAN_POINT('Ctrl Pts',(10.0502525316942,-8.94194140034058,-2.67705351804929));
#10558=CARTESIAN_POINT('Ctrl Pts',(10.0502525316942,-8.88723149748883,-2.66010336866474));
#10559=CARTESIAN_POINT('Ctrl Pts',(10.0502525316942,-8.84275317038967,-2.64863401651716));
#10560=CARTESIAN_POINT('Ctrl Pts',(10.0502525316942,-8.8089947353088,-2.64120584766726));
#10561=CARTESIAN_POINT('Ctrl Pts',(10.0502525316942,-8.78631177678628,-2.63677452882418));
#10562=CARTESIAN_POINT('Ctrl Pts',(10.0502525316942,-8.77492596468499,-2.63468906623289));
#10563=CARTESIAN_POINT('',(10.0502525316942,-9.041822881172,-1.47863151154858));
#10564=CARTESIAN_POINT('Origin',(10.0502525316942,0.,0.));
#10565=CARTESIAN_POINT('',(10.0502525316942,-10.7106795892491,-1.03854944428814));
#10566=CARTESIAN_POINT('Ctrl Pts',(10.0502525316942,-9.041822881172,-1.47863151154858));
#10567=CARTESIAN_POINT('Ctrl Pts',(10.0502525316942,-9.05241341063017,-1.48142903122265));
#10568=CARTESIAN_POINT('Ctrl Pts',(10.0502525316942,-9.0736287027809,-1.48681431784179));
#10569=CARTESIAN_POINT('Ctrl Pts',(10.0502525316942,-9.10555434079238,-1.49426299078246));
#10570=CARTESIAN_POINT('Ctrl Pts',(10.0502525316942,-9.14832762892595,-1.50293375169959));
#10571=CARTESIAN_POINT('Ctrl Pts',(10.0502525316942,-9.20213819442161,-1.51165206039235));
#10572=CARTESIAN_POINT('Ctrl Pts',(10.0502525316942,-9.25629193365179,-1.51821671513724));
#10573=CARTESIAN_POINT('Ctrl Pts',(10.0502525316942,-9.31078441132333,-1.52257856936539));
#10574=CARTESIAN_POINT('Ctrl Pts',(10.0502525316942,-9.36560546949212,-1.52467115182437));
#10575=CARTESIAN_POINT('Ctrl Pts',(10.0502525316942,-9.42073743324162,-1.52441199543777));
#10576=CARTESIAN_POINT('Ctrl Pts',(10.0502525316942,-9.47615638983506,-1.52172656066024));
#10577=CARTESIAN_POINT('Ctrl Pts',(10.0502525316942,-9.53183308717807,-1.51657146095807));
#10578=CARTESIAN_POINT('Ctrl Pts',(10.0502525316942,-9.58773391775221,-1.50895693238989));
#10579=CARTESIAN_POINT('Ctrl Pts',(10.0502525316942,-9.64382166809154,-1.49897455623114));
#10580=CARTESIAN_POINT('Ctrl Pts',(10.0502525316942,-9.70005659890418,-1.48681164197681));
#10581=CARTESIAN_POINT('Ctrl Pts',(10.0502525316942,-9.75639893594512,-1.472706711821));
#10582=CARTESIAN_POINT('Ctrl Pts',(10.0502525316942,-9.81281120439258,-1.45691330418438));
#10583=CARTESIAN_POINT('Ctrl Pts',(10.0502525316942,-9.86926046040473,-1.43966301743384));
#10584=CARTESIAN_POINT('Ctrl Pts',(10.0502525316942,-9.9257209332579,-1.42112478528011));
#10585=CARTESIAN_POINT('Ctrl Pts',(10.0502525316942,-9.98217543513636,-1.40137929597453));
#10586=CARTESIAN_POINT('Ctrl Pts',(10.0502525316942,-10.0386123354999,-1.38044913636065));
#10587=CARTESIAN_POINT('Ctrl Pts',(10.0502525316942,-10.0950232336429,-1.3583201853205));
#10588=CARTESIAN_POINT('Ctrl Pts',(10.0502525316942,-10.1514004985561,-1.33496549883664));
#10589=CARTESIAN_POINT('Ctrl Pts',(10.0502525316942,-10.2077346253654,-1.31037031610781));
#10590=CARTESIAN_POINT('Ctrl Pts',(10.0502525316942,-10.26401245069,-1.2845505698718));
#10591=CARTESIAN_POINT('Ctrl Pts',(10.0502525316942,-10.3202191159745,-1.2575411104082));
#10592=CARTESIAN_POINT('Ctrl Pts',(10.0502525316942,-10.3763394931394,-1.22938873407215));
#10593=CARTESIAN_POINT('Ctrl Pts',(10.0502525316942,-10.4323597856746,-1.20014382966931));
#10594=CARTESIAN_POINT('Ctrl Pts',(10.0502525316942,-10.4882691830915,-1.16985259538408));
#10595=CARTESIAN_POINT('Ctrl Pts',(10.0502525316942,-10.5440612301269,-1.13855017696687));
#10596=CARTESIAN_POINT('Ctrl Pts',(10.0502525316942,-10.599732595958,-1.10626216443499));
#10597=CARTESIAN_POINT('Ctrl Pts',(10.0502525316942,-10.6441722372873,-1.07965669109989));
#10598=CARTESIAN_POINT('Ctrl Pts',(10.0502525316942,-10.6774471807436,-1.05927071468098));
#10599=CARTESIAN_POINT('Ctrl Pts',(10.0502525316942,-10.6996061707058,-1.04548846715806));
#10600=CARTESIAN_POINT('Ctrl Pts',(10.0502525316942,-10.7106795892491,-1.03854944428814));
#10601=CARTESIAN_POINT('Ctrl Pts',(10.0502525316942,-10.7106795892491,-1.03854944428814));
#10602=CARTESIAN_POINT('Ctrl Pts',(10.0502525316942,-10.7069087245865,-1.00031843628634));
#10603=CARTESIAN_POINT('Ctrl Pts',(10.0502525316942,-10.6988602462966,-0.926048534485518));
#10604=CARTESIAN_POINT('Ctrl Pts',(10.0502525316942,-10.6852672767501,-0.821220046750494));
#10605=CARTESIAN_POINT('Ctrl Pts',(10.0502525316942,-10.6640973524763,-0.694625083433484));
#10606=CARTESIAN_POINT('Ctrl Pts',(10.0502525316942,-10.6325607057952,-0.558333537570359));
#10607=CARTESIAN_POINT('Ctrl Pts',(10.0502525316942,-10.596013814283,-0.443722777305705));
#10608=CARTESIAN_POINT('Ctrl Pts',(10.0502525316942,-10.5546263356355,-0.35006979143776));
#10609=CARTESIAN_POINT('Ctrl Pts',(10.0502525316942,-10.5087249476599,-0.275979784341796));
#10610=CARTESIAN_POINT('Ctrl Pts',(10.0502525316942,-10.4588324224655,-0.219218698708487));
#10611=CARTESIAN_POINT('Ctrl Pts',(10.0502525316942,-10.4057430679645,-0.176389733643621));
#10612=CARTESIAN_POINT('Ctrl Pts',(10.0502525316942,-10.3504388022425,-0.143293435954743));
#10613=CARTESIAN_POINT('Ctrl Pts',(10.0502525316942,-10.2939289512549,-0.1156151003885));
#10614=CARTESIAN_POINT('Ctrl Pts',(10.0502525316942,-10.237110176256,-0.0895255103702559));
#10615=CARTESIAN_POINT('Ctrl Pts',(10.0502525316942,-10.1806284708027,-0.0622734430034757));
#10616=CARTESIAN_POINT('Ctrl Pts',(10.0502525316942,-10.1247109492303,-0.0329060076605434));
#10617=CARTESIAN_POINT('Ctrl Pts',(10.0502525316942,-10.0692584999061,-0.0018837405250373));
#10618=CARTESIAN_POINT('Ctrl Pts',(10.0502525316942,-10.0139888357391,0.0295176561224922));
#10619=CARTESIAN_POINT('Ctrl Pts',(10.0502525316942,-9.95855906844526,0.0597188954606694));
#10620=CARTESIAN_POINT('Ctrl Pts',(10.0502525316942,-9.90269886586131,0.0873927181594359));
#10621=CARTESIAN_POINT('Ctrl Pts',(10.0502525316942,-9.84633157004081,0.111969973727218));
#10622=CARTESIAN_POINT('Ctrl Pts',(10.0502525316942,-9.78951336137147,0.133407037879776));
#10623=CARTESIAN_POINT('Ctrl Pts',(10.0502525316942,-9.73237897573987,0.151980202759258));
#10624=CARTESIAN_POINT('Ctrl Pts',(10.0502525316942,-9.67508881816964,0.168085081732297));
#10625=CARTESIAN_POINT('Ctrl Pts',(10.0502525316942,-9.61776871087166,0.182008602623653));
#10626=CARTESIAN_POINT('Ctrl Pts',(10.0502525316942,-9.56047634174856,0.193802962616848));
#10627=CARTESIAN_POINT('Ctrl Pts',(10.0502525316942,-9.50322667013965,0.203384169996506));
#10628=CARTESIAN_POINT('Ctrl Pts',(10.0502525316942,-9.44600537601646,0.210586047375026));
#10629=CARTESIAN_POINT('Ctrl Pts',(10.0502525316942,-9.38878575682053,0.215226755929044));
#10630=CARTESIAN_POINT('Ctrl Pts',(10.0502525316942,-9.33154666905179,0.21718266259851));
#10631=CARTESIAN_POINT('Ctrl Pts',(10.0502525316942,-9.27427657522174,0.216396922881075));
#10632=CARTESIAN_POINT('Ctrl Pts',(10.0502525316942,-9.2284309476721,0.2135603660237));
#10633=CARTESIAN_POINT('Ctrl Pts',(10.0502525316942,-9.1940293375968,0.210193044269049));
#10634=CARTESIAN_POINT('Ctrl Pts',(10.0502525316942,-9.1710872092551,0.207398059264383));
#10635=CARTESIAN_POINT('Ctrl Pts',(10.0502525316942,-9.15961421508102,0.205863042617261));
#10636=CARTESIAN_POINT('',(10.0502525316942,-10.5073910450885,2.32206279789789));
#10637=CARTESIAN_POINT('Ctrl Pts',(10.0502525316942,-9.05620683581208,1.38781479615277));
#10638=CARTESIAN_POINT('Ctrl Pts',(10.0502525316942,-9.06714350898568,1.38842685041928));
#10639=CARTESIAN_POINT('Ctrl Pts',(10.0502525316942,-9.08898459591562,1.38986102430324));
#10640=CARTESIAN_POINT('Ctrl Pts',(10.0502525316942,-9.12164944850753,1.39264248006707));
#10641=CARTESIAN_POINT('Ctrl Pts',(10.0502525316942,-9.16500867538789,1.39761376933417));
#10642=CARTESIAN_POINT('Ctrl Pts',(10.0502525316942,-9.21887966989633,1.40595054425593));
#10643=CARTESIAN_POINT('Ctrl Pts',(10.0502525316942,-9.27241152635132,1.41644161231465));
#10644=CARTESIAN_POINT('Ctrl Pts',(10.0502525316942,-9.32558483941339,1.42913234409394));
#10645=CARTESIAN_POINT('Ctrl Pts',(10.0502525316942,-9.37836940755697,1.44408281853422));
#10646=CARTESIAN_POINT('Ctrl Pts',(10.0502525316942,-9.43072293720942,1.4613660046363));
#10647=CARTESIAN_POINT('Ctrl Pts',(10.0502525316942,-9.48259965202034,1.48104540427845));
#10648=CARTESIAN_POINT('Ctrl Pts',(10.0502525316942,-9.53395832441854,1.50315324111201));
#10649=CARTESIAN_POINT('Ctrl Pts',(10.0502525316942,-9.58477015487067,1.52766939477237));
#10650=CARTESIAN_POINT('Ctrl Pts',(10.0502525316942,-9.63502805143792,1.55449526669738));
#10651=CARTESIAN_POINT('Ctrl Pts',(10.0502525316942,-9.68475210162498,1.5834404348547));
#10652=CARTESIAN_POINT('Ctrl Pts',(10.0502525316942,-9.73397818528844,1.61426576023972));
#10653=CARTESIAN_POINT('Ctrl Pts',(10.0502525316942,-9.78274900943559,1.64671853312854));
#10654=CARTESIAN_POINT('Ctrl Pts',(10.0502525316942,-9.8311048104422,1.68056831017818));
#10655=CARTESIAN_POINT('Ctrl Pts',(10.0502525316942,-9.87907328228114,1.71564646229066));
#10656=CARTESIAN_POINT('Ctrl Pts',(10.0502525316942,-9.92666301240917,1.75187093905158));
#10657=CARTESIAN_POINT('Ctrl Pts',(10.0502525316942,-9.97386991924375,1.78921666506164));
#10658=CARTESIAN_POINT('Ctrl Pts',(10.0502525316942,-10.0206816495736,1.8276944743413));
#10659=CARTESIAN_POINT('Ctrl Pts',(10.0502525316942,-10.0670826197184,1.86732763406234));
#10660=CARTESIAN_POINT('Ctrl Pts',(10.0502525316942,-10.1130592286672,1.9081272454134));
#10661=CARTESIAN_POINT('Ctrl Pts',(10.0502525316942,-10.1586038807877,1.95007408775204));
#10662=CARTESIAN_POINT('Ctrl Pts',(10.0502525316942,-10.2037132140826,1.99313042494654));
#10663=CARTESIAN_POINT('Ctrl Pts',(10.0502525316942,-10.2483873017624,2.03724707618484));
#10664=CARTESIAN_POINT('Ctrl Pts',(10.0502525316942,-10.2926285935634,2.08237185550883));
#10665=CARTESIAN_POINT('Ctrl Pts',(10.0502525316942,-10.3364410841241,2.12845748520948));
#10666=CARTESIAN_POINT('Ctrl Pts',(10.0502525316942,-10.3798294947586,2.17546854490588));
#10667=CARTESIAN_POINT('Ctrl Pts',(10.0502525316942,-10.4227985654164,2.22337966776441));
#10668=CARTESIAN_POINT('Ctrl Pts',(10.0502525316942,-10.4568416324806,2.26241558094358));
#10669=CARTESIAN_POINT('Ctrl Pts',(10.0502525316942,-10.4821883711236,2.29208631967267));
#10670=CARTESIAN_POINT('Ctrl Pts',(10.0502525316942,-10.4990038742164,2.31204152046505));
#10671=CARTESIAN_POINT('Ctrl Pts',(10.0502525316942,-10.5073910450885,2.32206279789789));
#10672=CARTESIAN_POINT('',(10.0502525316942,-8.64769560732005,3.02626384252387));
#10673=CARTESIAN_POINT('Ctrl Pts',(10.0502525316942,-10.5073910450885,2.32206279789789));
#10674=CARTESIAN_POINT('Ctrl Pts',(10.0502525316942,-10.4919907084944,2.35725738591831));
#10675=CARTESIAN_POINT('Ctrl Pts',(10.0502525316942,-10.4613854889436,2.42540514342016));
#10676=CARTESIAN_POINT('Ctrl Pts',(10.0502525316942,-10.4160640224759,2.52090250118004));
#10677=CARTESIAN_POINT('Ctrl Pts',(10.0502525316942,-10.3568102329785,2.63475959960257));
#10678=CARTESIAN_POINT('Ctrl Pts',(10.0502525316942,-10.284700695789,2.75463520264158));
#10679=CARTESIAN_POINT('Ctrl Pts',(10.0502525316942,-10.214525863806,2.85234290245999));
#10680=CARTESIAN_POINT('Ctrl Pts',(10.0502525316942,-10.1462236683382,2.92862275068379));
#10681=CARTESIAN_POINT('Ctrl Pts',(10.0502525316942,-10.0796737828909,2.98490222577489));
#10682=CARTESIAN_POINT('Ctrl Pts',(10.0502525316942,-10.0146830316105,3.02346758796109));
#10683=CARTESIAN_POINT('Ctrl Pts',(10.0502525316942,-9.95095717700994,3.04779484151101));
#10684=CARTESIAN_POINT('Ctrl Pts',(10.0502525316942,-9.88813237627935,3.06218133312374));
#10685=CARTESIAN_POINT('Ctrl Pts',(10.0502525316942,-9.82583523819669,3.07104249021943));
#10686=CARTESIAN_POINT('Ctrl Pts',(10.0502525316942,-9.76373524529424,3.07829719773955));
#10687=CARTESIAN_POINT('Ctrl Pts',(10.0502525316942,-9.70159659932322,3.08676164713489));
#10688=CARTESIAN_POINT('Ctrl Pts',(10.0502525316942,-9.6393408394545,3.09741227343545));
#10689=CARTESIAN_POINT('Ctrl Pts',(10.0502525316942,-9.57701601843134,3.10978045352404));
#10690=CARTESIAN_POINT('Ctrl Pts',(10.0502525316942,-9.51474787896063,3.12256569092543));
#10691=CARTESIAN_POINT('Ctrl Pts',(10.0502525316942,-9.45269834137241,3.13416003631015));
#10692=CARTESIAN_POINT('Ctrl Pts',(10.0502525316942,-9.39102045019014,3.14321765381094));
#10693=CARTESIAN_POINT('Ctrl Pts',(10.0502525316942,-9.32981717654858,3.14917356053584));
#10694=CARTESIAN_POINT('Ctrl Pts',(10.0502525316942,-9.26915543181673,3.15200362801959));
#10695=CARTESIAN_POINT('Ctrl Pts',(10.0502525316942,-9.2090779784702,3.15201226138312));
#10696=CARTESIAN_POINT('Ctrl Pts',(10.0502525316942,-9.14961511949843,3.14962527917495));
#10697=CARTESIAN_POINT('Ctrl Pts',(10.0502525316942,-9.09079785336098,3.14515444717397));
#10698=CARTESIAN_POINT('Ctrl Pts',(10.0502525316942,-9.0326649146968,3.13866723439399));
#10699=CARTESIAN_POINT('Ctrl Pts',(10.0502525316942,-8.97525648555044,3.13008838265685));
#10700=CARTESIAN_POINT('Ctrl Pts',(10.0502525316942,-8.91861029840238,3.11925542274306));
#10701=CARTESIAN_POINT('Ctrl Pts',(10.0502525316942,-8.86275714889703,3.10598716411038));
#10702=CARTESIAN_POINT('Ctrl Pts',(10.0502525316942,-8.8077151330875,3.09015949103058));
#10703=CARTESIAN_POINT('Ctrl Pts',(10.0502525316942,-8.75349084408744,3.07171477588927));
#10704=CARTESIAN_POINT('Ctrl Pts',(10.0502525316942,-8.71076560553715,3.0548499719756));
#10705=CARTESIAN_POINT('Ctrl Pts',(10.0502525316942,-8.67908828975171,3.04101677653125));
#10706=CARTESIAN_POINT('Ctrl Pts',(10.0502525316942,-8.65813272696012,3.0312690802849));
#10707=CARTESIAN_POINT('Ctrl Pts',(10.0502525316942,-8.64769560732005,3.02626384252387));
#10708=CARTESIAN_POINT('',(10.0502525316942,-8.18410616705958,4.11841212213242));
#10709=CARTESIAN_POINT('Origin',(10.0502525316942,0.,0.));
#10710=CARTESIAN_POINT('',(10.0502525316942,-9.2755658561365,5.45537535466284));
#10711=CARTESIAN_POINT('Ctrl Pts',(10.0502525316942,-8.18410616705958,4.11841212213242));
#10712=CARTESIAN_POINT('Ctrl Pts',(10.0502525316942,-8.19431842617809,4.12237383820348));
#10713=CARTESIAN_POINT('Ctrl Pts',(10.0502525316942,-8.21464735012275,4.1304870856583));
#10714=CARTESIAN_POINT('Ctrl Pts',(10.0502525316942,-8.24485395393399,4.14322640185693));
#10715=CARTESIAN_POINT('Ctrl Pts',(10.0502525316942,-8.28455481633258,4.16135311687778));
#10716=CARTESIAN_POINT('Ctrl Pts',(10.0502525316942,-8.33321297157003,4.18592891379899));
#10717=CARTESIAN_POINT('Ctrl Pts',(10.0502525316942,-8.38088287416164,4.21244876582417));
#10718=CARTESIAN_POINT('Ctrl Pts',(10.0502525316942,-8.42753204825146,4.24094982636281));
#10719=CARTESIAN_POINT('Ctrl Pts',(10.0502525316942,-8.47311320506822,4.27147990109805));
#10720=CARTESIAN_POINT('Ctrl Pts',(10.0502525316942,-8.51756357237276,4.3040953182409));
#10721=CARTESIAN_POINT('Ctrl Pts',(10.0502525316942,-8.56081999110915,4.33884232599626));
#10722=CARTESIAN_POINT('Ctrl Pts',(10.0502525316942,-8.60283329387128,4.37573883085758));
#10723=CARTESIAN_POINT('Ctrl Pts',(10.0502525316942,-8.6435823082099,4.41475679767577));
#10724=CARTESIAN_POINT('Ctrl Pts',(10.0502525316942,-8.68309075792173,4.45580026211617));
#10725=CARTESIAN_POINT('Ctrl Pts',(10.0502525316942,-8.72143659100306,4.4986943294444));
#10726=CARTESIAN_POINT('Ctrl Pts',(10.0502525316942,-8.75872782924178,4.54322265243728));
#10727=CARTESIAN_POINT('Ctrl Pts',(10.0502525316942,-8.79508318101477,4.58915808705618));
#10728=CARTESIAN_POINT('Ctrl Pts',(10.0502525316942,-8.83061212429863,4.63629390238203));
#10729=CARTESIAN_POINT('Ctrl Pts',(10.0502525316942,-8.86539310688376,4.68447828052063));
#10730=CARTESIAN_POINT('Ctrl Pts',(10.0502525316942,-8.89945965089929,4.73363584056076));
#10731=CARTESIAN_POINT('Ctrl Pts',(10.0502525316942,-8.93281562325407,4.78374147310216));
#10732=CARTESIAN_POINT('Ctrl Pts',(10.0502525316942,-8.96544592744964,4.83480166455838));
#10733=CARTESIAN_POINT('Ctrl Pts',(10.0502525316942,-8.99732855257362,4.88683372770265));
#10734=CARTESIAN_POINT('Ctrl Pts',(10.0502525316942,-9.02844713284016,4.93984401744929));
#10735=CARTESIAN_POINT('Ctrl Pts',(10.0502525316942,-9.05880038387882,4.99381190670161));
#10736=CARTESIAN_POINT('Ctrl Pts',(10.0502525316942,-9.08839676934597,5.04870046735128));
#10737=CARTESIAN_POINT('Ctrl Pts',(10.0502525316942,-9.11725155657582,5.10446294828982));
#10738=CARTESIAN_POINT('Ctrl Pts',(10.0502525316942,-9.14538320175401,5.16105047473192));
#10739=CARTESIAN_POINT('Ctrl Pts',(10.0502525316942,-9.17281011362288,5.21841931731543));
#10740=CARTESIAN_POINT('Ctrl Pts',(10.0502525316942,-9.19954772791879,5.27653724822262));
#10741=CARTESIAN_POINT('Ctrl Pts',(10.0502525316942,-9.2256083913841,5.33538160688598));
#10742=CARTESIAN_POINT('Ctrl Pts',(10.0502525316942,-9.24592251158686,5.38302685274804));
#10743=CARTESIAN_POINT('Ctrl Pts',(10.0502525316942,-9.26085993003723,5.41907797515233));
#10744=CARTESIAN_POINT('Ctrl Pts',(10.0502525316942,-9.27068592765741,5.44325277512453));
#10745=CARTESIAN_POINT('Ctrl Pts',(10.0502525316942,-9.2755658561365,5.45537535466284));
#10746=CARTESIAN_POINT('',(10.0502525316942,-7.28928030147641,5.55043285230422));
#10747=CARTESIAN_POINT('Ctrl Pts',(10.0502525316942,-9.2755658561365,5.45537535466284));
#10748=CARTESIAN_POINT('Ctrl Pts',(10.0502525316942,-9.25004353985722,5.48408843121132));
#10749=CARTESIAN_POINT('Ctrl Pts',(10.0502525316942,-9.19987743117415,5.53944326709657));
#10750=CARTESIAN_POINT('Ctrl Pts',(10.0502525316942,-9.12726384869626,5.61626154813455));
#10751=CARTESIAN_POINT('Ctrl Pts',(10.0502525316942,-9.03572636773682,5.70623565557996));
#10752=CARTESIAN_POINT('Ctrl Pts',(10.0502525316942,-8.93010252395574,5.79796105654696));
#10753=CARTESIAN_POINT('Ctrl Pts',(10.0502525316942,-8.83316895299322,5.86920138549131));
#10754=CARTESIAN_POINT('Ctrl Pts',(10.0502525316942,-8.74463793548674,5.92064129305387));
#10755=CARTESIAN_POINT('Ctrl Pts',(10.0502525316942,-8.6639539190358,5.95360120899603));
#10756=CARTESIAN_POINT('Ctrl Pts',(10.0502525316942,-8.59022668922188,5.97019580138365));
#10757=CARTESIAN_POINT('Ctrl Pts',(10.0502525316942,-8.52210226517413,5.97364002234323));
#10758=CARTESIAN_POINT('Ctrl Pts',(10.0502525316942,-8.45790665865659,5.96790845784416));
#10759=CARTESIAN_POINT('Ctrl Pts',(10.0502525316942,-8.39592031140414,5.95708504467347));
#10760=CARTESIAN_POINT('Ctrl Pts',(10.0502525316942,-8.33461788057945,5.94479472837688));
#10761=CARTESIAN_POINT('Ctrl Pts',(10.0502525316942,-8.27290485770376,5.93364300051867));
#10762=CARTESIAN_POINT('Ctrl Pts',(10.0502525316942,-8.2104048870761,5.92453426026728));
#10763=CARTESIAN_POINT('Ctrl Pts',(10.0502525316942,-8.14730848207823,5.91703766966772));
#10764=CARTESIAN_POINT('Ctrl Pts',(10.0502525316942,-8.08413710664289,5.90995523970613));
#10765=CARTESIAN_POINT('Ctrl Pts',(10.0502525316942,-8.02154163982398,5.90180775582857));
#10766=CARTESIAN_POINT('Ctrl Pts',(10.0502525316942,-7.96008352176745,5.89136254542228));
#10767=CARTESIAN_POINT('Ctrl Pts',(10.0502525316942,-7.90003527315714,5.87811409765682));
#10768=CARTESIAN_POINT('Ctrl Pts',(10.0502525316942,-7.84146798659238,5.86206014174823));
#10769=CARTESIAN_POINT('Ctrl Pts',(10.0502525316942,-7.78432826524869,5.84350339850201));
#10770=CARTESIAN_POINT('Ctrl Pts',(10.0502525316942,-7.72851334381364,5.82285820956226));
#10771=CARTESIAN_POINT('Ctrl Pts',(10.0502525316942,-7.67395636265026,5.80043066085532));
#10772=CARTESIAN_POINT('Ctrl Pts',(10.0502525316942,-7.62067331151744,5.77629688888814));
#10773=CARTESIAN_POINT('Ctrl Pts',(10.0502525316942,-7.56872566186653,5.75039773581461));
#10774=CARTESIAN_POINT('Ctrl Pts',(10.0502525316942,-7.51819950516883,5.72259034420254));
#10775=CARTESIAN_POINT('Ctrl Pts',(10.0502525316942,-7.46918012077942,5.69271190798352));
#10776=CARTESIAN_POINT('Ctrl Pts',(10.0502525316942,-7.42172307293681,5.66064997807339));
#10777=CARTESIAN_POINT('Ctrl Pts',(10.0502525316942,-7.37585243997691,5.62635178473812));
#10778=CARTESIAN_POINT('Ctrl Pts',(10.0502525316942,-7.34042983445952,5.59710957827922));
#10779=CARTESIAN_POINT('Ctrl Pts',(10.0502525316942,-7.31457760934185,5.5741645986968));
#10780=CARTESIAN_POINT('Ctrl Pts',(10.0502525316942,-7.2976598885924,5.55841836363355));
#10781=CARTESIAN_POINT('Ctrl Pts',(10.0502525316942,-7.28928030147641,5.55043285230422));
#10782=CARTESIAN_POINT('',(10.0502525316942,-6.51088816465466,6.44587057493322));
#10783=CARTESIAN_POINT('Origin',(10.0502525316942,0.,0.));
#10784=CARTESIAN_POINT('',(10.0502525316942,-7.13578365451838,8.05467776187827));
#10785=CARTESIAN_POINT('Ctrl Pts',(10.0502525316942,-6.51088816465466,6.44587057493322));
#10786=CARTESIAN_POINT('Ctrl Pts',(10.0502525316942,-6.51937636264257,6.45279415243689));
#10787=CARTESIAN_POINT('Ctrl Pts',(10.0502525316942,-6.5362031868863,6.46679229227336));
#10788=CARTESIAN_POINT('Ctrl Pts',(10.0502525316942,-6.56099470907402,6.48824245587723));
#10789=CARTESIAN_POINT('Ctrl Pts',(10.0502525316942,-6.59315100996711,6.51775022748935));
#10790=CARTESIAN_POINT('Ctrl Pts',(10.0502525316942,-6.63183332667763,6.55615939617772));
#10791=CARTESIAN_POINT('Ctrl Pts',(10.0502525316942,-6.66897501320444,6.59611208427845));
#10792=CARTESIAN_POINT('Ctrl Pts',(10.0502525316942,-6.70453370213821,6.63763359119236));
#10793=CARTESIAN_POINT('Ctrl Pts',(10.0502525316942,-6.73844964641633,6.68075476979194));
#10794=CARTESIAN_POINT('Ctrl Pts',(10.0502525316942,-6.77064573971725,6.72550979370064));
#10795=CARTESIAN_POINT('Ctrl Pts',(10.0502525316942,-6.801047622728,6.77192313035347));
#10796=CARTESIAN_POINT('Ctrl Pts',(10.0502525316942,-6.82960300105583,6.81999661627367));
#10797=CARTESIAN_POINT('Ctrl Pts',(10.0502525316942,-6.8563004018424,6.86969704580336));
#10798=CARTESIAN_POINT('Ctrl Pts',(10.0502525316942,-6.88119204236944,6.92094048249309));
#10799=CARTESIAN_POINT('Ctrl Pts',(10.0502525316942,-6.90440610103192,6.97358467882161));
#10800=CARTESIAN_POINT('Ctrl Pts',(10.0502525316942,-6.92611216762375,7.02745725692073));
#10801=CARTESIAN_POINT('Ctrl Pts',(10.0502525316942,-6.94649333188842,7.08237887287821));
#10802=CARTESIAN_POINT('Ctrl Pts',(10.0502525316942,-6.96571759693621,7.13818674446165));
#10803=CARTESIAN_POINT('Ctrl Pts',(10.0502525316942,-6.98390648535874,7.19476072597386));
#10804=CARTESIAN_POINT('Ctrl Pts',(10.0502525316942,-7.00111517257795,7.25203948481561));
#10805=CARTESIAN_POINT('Ctrl Pts',(10.0502525316942,-7.01735509547412,7.31000033546873));
#10806=CARTESIAN_POINT('Ctrl Pts',(10.0502525316942,-7.032609892012,7.36864478180451));
#10807=CARTESIAN_POINT('Ctrl Pts',(10.0502525316942,-7.0468532786288,7.42798248750274));
#10808=CARTESIAN_POINT('Ctrl Pts',(10.0502525316942,-7.06006772676068,7.48801443914016));
#10809=CARTESIAN_POINT('Ctrl Pts',(10.0502525316942,-7.07225838902223,7.54872062228975));
#10810=CARTESIAN_POINT('Ctrl Pts',(10.0502525316942,-7.08344472624203,7.6100685316471));
#10811=CARTESIAN_POINT('Ctrl Pts',(10.0502525316942,-7.09365570540476,7.67201842213158));
#10812=CARTESIAN_POINT('Ctrl Pts',(10.0502525316942,-7.10292398252533,7.73452951433514));
#10813=CARTESIAN_POINT('Ctrl Pts',(10.0502525316942,-7.11128057847415,7.79756590777721));
#10814=CARTESIAN_POINT('Ctrl Pts',(10.0502525316942,-7.11875013245223,7.86110172188657));
#10815=CARTESIAN_POINT('Ctrl Pts',(10.0502525316942,-7.12535138940982,7.92511922053603));
#10816=CARTESIAN_POINT('Ctrl Pts',(10.0502525316942,-7.12994807512891,7.97670995045205));
#10817=CARTESIAN_POINT('Ctrl Pts',(10.0502525316942,-7.13301399479354,8.01561252148766));
#10818=CARTESIAN_POINT('Ctrl Pts',(10.0502525316942,-7.13488864983229,8.04164052278268));
#10819=CARTESIAN_POINT('Ctrl Pts',(10.0502525316942,-7.13578365451838,8.05467776187827));
#10820=CARTESIAN_POINT('',(10.0502525316942,-5.21733945232202,7.53128682236137));
#10821=CARTESIAN_POINT('Ctrl Pts',(10.0502525316942,-7.13578365451838,8.05467776187827));
#10822=CARTESIAN_POINT('Ctrl Pts',(10.0502525316942,-7.10263766069576,8.07409869096647));
#10823=CARTESIAN_POINT('Ctrl Pts',(10.0502525316942,-7.03782127112617,8.11124208821886));
#10824=CARTESIAN_POINT('Ctrl Pts',(10.0502525316942,-6.94502349601963,8.16186178396251));
#10825=CARTESIAN_POINT('Ctrl Pts',(10.0502525316942,-6.83016265001357,8.21914560790757));
#10826=CARTESIAN_POINT('Ctrl Pts',(10.0502525316942,-6.70136369739477,8.27374208546745));
#10827=CARTESIAN_POINT('Ctrl Pts',(10.0502525316942,-6.58715992075444,8.31154154378012));
#10828=CARTESIAN_POINT('Ctrl Pts',(10.0502525316942,-6.48706611403476,8.33310621412631));
#10829=CARTESIAN_POINT('Ctrl Pts',(10.0502525316942,-6.40014588026893,8.33952022470187));
#10830=CARTESIAN_POINT('Ctrl Pts',(10.0502525316942,-6.32489910686351,8.33251965296669));
#10831=CARTESIAN_POINT('Ctrl Pts',(10.0502525316942,-6.25904460664515,8.31474369699109));
#10832=CARTESIAN_POINT('Ctrl Pts',(10.0502525316942,-6.19976210758369,8.28945512184757));
#10833=CARTESIAN_POINT('Ctrl Pts',(10.0502525316942,-6.1441542067148,8.26000660950279));
#10834=CARTESIAN_POINT('Ctrl Pts',(10.0502525316942,-6.08965004701613,8.22937433118026));
#10835=CARTESIAN_POINT('Ctrl Pts',(10.0502525316942,-6.03440354789477,8.19969803488993));
#10836=CARTESIAN_POINT('Ctrl Pts',(10.0502525316942,-5.9777772990961,8.17172155504672));
#10837=CARTESIAN_POINT('Ctrl Pts',(10.0502525316942,-5.92008562586321,8.1450940122787));
#10838=CARTESIAN_POINT('Ctrl Pts',(10.0502525316942,-5.86219466883171,8.11883719254497));
#10839=CARTESIAN_POINT('Ctrl Pts',(10.0502525316942,-5.80518055320261,8.09174541189394));
#10840=CARTESIAN_POINT('Ctrl Pts',(10.0502525316942,-5.74995815707108,8.06281982355119));
#10841=CARTESIAN_POINT('Ctrl Pts',(10.0502525316942,-5.69694287444675,8.03166387167001));
#10842=CARTESIAN_POINT('Ctrl Pts',(10.0502525316942,-5.64620302012031,7.99829736542789));
#10843=CARTESIAN_POINT('Ctrl Pts',(10.0502525316942,-5.59759426482043,7.96299170889331));
#10844=CARTESIAN_POINT('Ctrl Pts',(10.0502525316942,-5.5508908343176,7.92610920815888));
#10845=CARTESIAN_POINT('Ctrl Pts',(10.0502525316942,-5.50593455556538,7.88792030747535));
#10846=CARTESIAN_POINT('Ctrl Pts',(10.0502525316942,-5.46271710825366,7.84850235807098));
#10847=CARTESIAN_POINT('Ctrl Pts',(10.0502525316942,-5.42131523598658,7.80781809321391));
#10848=CARTESIAN_POINT('Ctrl Pts',(10.0502525316942,-5.38185496199325,7.76575825114004));
#10849=CARTESIAN_POINT('Ctrl Pts',(10.0502525316942,-5.34446770160195,7.72219434684711));
#10850=CARTESIAN_POINT('Ctrl Pts',(10.0502525316942,-5.3092410482218,7.67703660519485));
#10851=CARTESIAN_POINT('Ctrl Pts',(10.0502525316942,-5.27621420845565,7.63024227979884));
#10852=CARTESIAN_POINT('Ctrl Pts',(10.0502525316942,-5.25156164740301,7.59148510170534));
#10853=CARTESIAN_POINT('Ctrl Pts',(10.0502525316942,-5.23406510887067,7.56167435245346));
#10854=CARTESIAN_POINT('Ctrl Pts',(10.0502525316942,-5.22284125454301,7.54147092977177));
#10855=CARTESIAN_POINT('Ctrl Pts',(10.0502525316942,-5.21733945232202,7.53128682236137));
#10856=CARTESIAN_POINT('',(10.0502525316942,-4.20033906466803,8.14236230483842));
#10857=CARTESIAN_POINT('Origin',(10.0502525316942,0.,0.));
#10858=CARTESIAN_POINT('',(10.0502525316942,-4.29750123086779,9.86553218952113));
#10859=CARTESIAN_POINT('Ctrl Pts',(10.0502525316942,-4.20033906466803,8.14236230483842));
#10860=CARTESIAN_POINT('Ctrl Pts',(10.0502525316942,-4.20627231756552,8.15157001576925));
#10861=CARTESIAN_POINT('Ctrl Pts',(10.0502525316942,-4.21794991531197,8.17008281252941));
#10862=CARTESIAN_POINT('Ctrl Pts',(10.0502525316942,-4.23489958895176,8.1981441320729));
#10863=CARTESIAN_POINT('Ctrl Pts',(10.0502525316942,-4.2563636455618,8.23614453399815));
#10864=CARTESIAN_POINT('Ctrl Pts',(10.0502525316942,-4.28128362907021,8.28462731741005));
#10865=CARTESIAN_POINT('Ctrl Pts',(10.0502525316942,-4.30426141247364,8.33410199410829));
#10866=CARTESIAN_POINT('Ctrl Pts',(10.0502525316942,-4.32524888402656,8.38457953300338));
#10867=CARTESIAN_POINT('Ctrl Pts',(10.0502525316942,-4.34417968683382,8.43607081406306));
#10868=CARTESIAN_POINT('Ctrl Pts',(10.0502525316942,-4.36096992819547,8.48858451117083));
#10869=CARTESIAN_POINT('Ctrl Pts',(10.0502525316942,-4.37554132734911,8.54212091594884));
#10870=CARTESIAN_POINT('Ctrl Pts',(10.0502525316942,-4.38784358185488,8.59666561517837));
#10871=CARTESIAN_POINT('Ctrl Pts',(10.0502525316942,-4.39787604148868,8.65218348309394));
#10872=CARTESIAN_POINT('Ctrl Pts',(10.0502525316942,-4.4057143056259,8.70861082741579));
#10873=CARTESIAN_POINT('Ctrl Pts',(10.0502525316942,-4.41152423606579,8.76585197201427));
#10874=CARTESIAN_POINT('Ctrl Pts',(10.0502525316942,-4.41552038997767,8.82379538192297));
#10875=CARTESIAN_POINT('Ctrl Pts',(10.0502525316942,-4.41793231637186,8.88232706878773));
#10876=CARTESIAN_POINT('Ctrl Pts',(10.0502525316942,-4.41897009817737,8.94134413332185));
#10877=CARTESIAN_POINT('Ctrl Pts',(10.0502525316942,-4.41878643730905,9.00076986272314));
#10878=CARTESIAN_POINT('Ctrl Pts',(10.0502525316942,-4.41745276152696,9.06056297636652));
#10879=CARTESIAN_POINT('Ctrl Pts',(10.0502525316942,-4.41498695816126,9.12070543323243));
#10880=CARTESIAN_POINT('Ctrl Pts',(10.0502525316942,-4.4113730012699,9.18119360744053));
#10881=CARTESIAN_POINT('Ctrl Pts',(10.0502525316942,-4.40658290745794,9.24202856762888));
#10882=CARTESIAN_POINT('Ctrl Pts',(10.0502525316942,-4.40059970120156,9.3032058354636));
#10883=CARTESIAN_POINT('Ctrl Pts',(10.0502525316942,-4.3934344677265,9.36470796833893));
#10884=CARTESIAN_POINT('Ctrl Pts',(10.0502525316942,-4.38511576007207,9.42651006560004));
#10885=CARTESIAN_POINT('Ctrl Pts',(10.0502525316942,-4.37568340938316,9.48858327871958));
#10886=CARTESIAN_POINT('Ctrl Pts',(10.0502525316942,-4.36518107490567,9.55089891543934));
#10887=CARTESIAN_POINT('Ctrl Pts',(10.0502525316942,-4.35364935309914,9.61343241834946));
#10888=CARTESIAN_POINT('Ctrl Pts',(10.0502525316942,-4.34111967477257,9.67616678749592));
#10889=CARTESIAN_POINT('Ctrl Pts',(10.0502525316942,-4.32761534819777,9.73909094732754));
#10890=CARTESIAN_POINT('Ctrl Pts',(10.0502525316942,-4.316044643808,9.78957710119959));
#10891=CARTESIAN_POINT('Ctrl Pts',(10.0502525316942,-4.30693895110861,9.8275230661634));
#10892=CARTESIAN_POINT('Ctrl Pts',(10.0502525316942,-4.30067875926925,9.85285646666673));
#10893=CARTESIAN_POINT('Ctrl Pts',(10.0502525316942,-4.29750123086779,9.86553218952113));
#10894=CARTESIAN_POINT('',(10.0502525316942,-2.63468906623289,8.77492596468499));
#10895=CARTESIAN_POINT('Ctrl Pts',(10.0502525316942,-4.29750123086779,9.86553218952113));
#10896=CARTESIAN_POINT('Ctrl Pts',(10.0502525316942,-4.25997612031891,9.87375991529634));
#10897=CARTESIAN_POINT('Ctrl Pts',(10.0502525316942,-4.18685412967622,9.88905601939953));
#10898=CARTESIAN_POINT('Ctrl Pts',(10.0502525316942,-4.08295585472858,9.9085221213413));
#10899=CARTESIAN_POINT('Ctrl Pts',(10.0502525316942,-3.95601502356553,9.9275083219784));
#10900=CARTESIAN_POINT('Ctrl Pts',(10.0502525316942,-3.81664870098641,9.93963159251159));
#10901=CARTESIAN_POINT('Ctrl Pts',(10.0502525316942,-3.69635378003033,9.94029010584861));
#10902=CARTESIAN_POINT('Ctrl Pts',(10.0502525316942,-3.59449506329373,9.92986863879505));
#10903=CARTESIAN_POINT('Ctrl Pts',(10.0502525316942,-3.50984697030288,9.90910889595984));
#10904=CARTESIAN_POINT('Ctrl Pts',(10.0502525316942,-3.44044633176199,9.87919842483915));
#10905=CARTESIAN_POINT('Ctrl Pts',(10.0502525316942,-3.38330805268968,9.84194232635164));
#10906=CARTESIAN_POINT('Ctrl Pts',(10.0502525316942,-3.3347416451379,9.79957216249457));
#10907=CARTESIAN_POINT('Ctrl Pts',(10.0502525316942,-3.29095547943264,9.75438117654386));
#10908=CARTESIAN_POINT('Ctrl Pts',(10.0502525316942,-3.24858483776411,9.70840543702524));
#10909=CARTESIAN_POINT('Ctrl Pts',(10.0502525316942,-3.20521277465607,9.66310949495059));
#10910=CARTESIAN_POINT('Ctrl Pts',(10.0502525316942,-3.16000321945708,9.61900380828622));
#10911=CARTESIAN_POINT('Ctrl Pts',(10.0502525316942,-3.11336354092674,9.57585180276088));
#10912=CARTESIAN_POINT('Ctrl Pts',(10.0502525316942,-3.06641977252332,9.53299079371256));
#10913=CARTESIAN_POINT('Ctrl Pts',(10.0502525316942,-3.02056794696251,9.4896066485377));
#10914=CARTESIAN_POINT('Ctrl Pts',(10.0502525316942,-2.97698682564639,9.44503212038191));
#10915=CARTESIAN_POINT('Ctrl Pts',(10.0502525316942,-2.9361940142505,9.39901842603143));
#10916=CARTESIAN_POINT('Ctrl Pts',(10.0502525316942,-2.89824836262921,9.35160551556488));
#10917=CARTESIAN_POINT('Ctrl Pts',(10.0502525316942,-2.86292873701901,9.30300690939252));
#10918=CARTESIAN_POINT('Ctrl Pts',(10.0502525316942,-2.82990845462794,9.25349741301079));
#10919=CARTESIAN_POINT('Ctrl Pts',(10.0502525316942,-2.79895351207997,9.20328535602728));
#10920=CARTESIAN_POINT('Ctrl Pts',(10.0502525316942,-2.77003209344587,9.15244173271444));
#10921=CARTESIAN_POINT('Ctrl Pts',(10.0502525316942,-2.74322870228394,9.10095481538197));
#10922=CARTESIAN_POINT('Ctrl Pts',(10.0502525316942,-2.71869695754934,9.04875963323664));
#10923=CARTESIAN_POINT('Ctrl Pts',(10.0502525316942,-2.69660154669561,8.99577459934956));
#10924=CARTESIAN_POINT('Ctrl Pts',(10.0502525316942,-2.67705351804929,8.94194140034058));
#10925=CARTESIAN_POINT('Ctrl Pts',(10.0502525316942,-2.66010336866474,8.88723149748883));
#10926=CARTESIAN_POINT('Ctrl Pts',(10.0502525316942,-2.64863401651716,8.84275317038967));
#10927=CARTESIAN_POINT('Ctrl Pts',(10.0502525316942,-2.64120584766726,8.8089947353088));
#10928=CARTESIAN_POINT('Ctrl Pts',(10.0502525316942,-2.63677452882418,8.78631177678628));
#10929=CARTESIAN_POINT('Ctrl Pts',(10.0502525316942,-2.63468906623289,8.77492596468499));
#10930=CARTESIAN_POINT('',(10.0502525316942,-1.47863151154858,9.041822881172));
#10931=CARTESIAN_POINT('Origin',(10.0502525316942,0.,0.));
#10932=CARTESIAN_POINT('',(10.0502525316942,-1.03854944428814,10.7106795892491));
#10933=CARTESIAN_POINT('Ctrl Pts',(10.0502525316942,-1.47863151154858,9.041822881172));
#10934=CARTESIAN_POINT('Ctrl Pts',(10.0502525316942,-1.48142903122265,9.05241341063017));
#10935=CARTESIAN_POINT('Ctrl Pts',(10.0502525316942,-1.48681431784179,9.0736287027809));
#10936=CARTESIAN_POINT('Ctrl Pts',(10.0502525316942,-1.49426299078246,9.10555434079238));
#10937=CARTESIAN_POINT('Ctrl Pts',(10.0502525316942,-1.50293375169959,9.14832762892595));
#10938=CARTESIAN_POINT('Ctrl Pts',(10.0502525316942,-1.51165206039235,9.20213819442161));
#10939=CARTESIAN_POINT('Ctrl Pts',(10.0502525316942,-1.51821671513724,9.25629193365179));
#10940=CARTESIAN_POINT('Ctrl Pts',(10.0502525316942,-1.52257856936539,9.31078441132333));
#10941=CARTESIAN_POINT('Ctrl Pts',(10.0502525316942,-1.52467115182437,9.36560546949212));
#10942=CARTESIAN_POINT('Ctrl Pts',(10.0502525316942,-1.52441199543777,9.42073743324162));
#10943=CARTESIAN_POINT('Ctrl Pts',(10.0502525316942,-1.52172656066024,9.47615638983506));
#10944=CARTESIAN_POINT('Ctrl Pts',(10.0502525316942,-1.51657146095807,9.53183308717807));
#10945=CARTESIAN_POINT('Ctrl Pts',(10.0502525316942,-1.50895693238989,9.58773391775221));
#10946=CARTESIAN_POINT('Ctrl Pts',(10.0502525316942,-1.49897455623114,9.64382166809154));
#10947=CARTESIAN_POINT('Ctrl Pts',(10.0502525316942,-1.48681164197681,9.70005659890418));
#10948=CARTESIAN_POINT('Ctrl Pts',(10.0502525316942,-1.472706711821,9.75639893594512));
#10949=CARTESIAN_POINT('Ctrl Pts',(10.0502525316942,-1.45691330418438,9.81281120439258));
#10950=CARTESIAN_POINT('Ctrl Pts',(10.0502525316942,-1.43966301743384,9.86926046040473));
#10951=CARTESIAN_POINT('Ctrl Pts',(10.0502525316942,-1.42112478528011,9.9257209332579));
#10952=CARTESIAN_POINT('Ctrl Pts',(10.0502525316942,-1.40137929597453,9.98217543513636));
#10953=CARTESIAN_POINT('Ctrl Pts',(10.0502525316942,-1.38044913636065,10.0386123354999));
#10954=CARTESIAN_POINT('Ctrl Pts',(10.0502525316942,-1.3583201853205,10.0950232336429));
#10955=CARTESIAN_POINT('Ctrl Pts',(10.0502525316942,-1.33496549883664,10.1514004985561));
#10956=CARTESIAN_POINT('Ctrl Pts',(10.0502525316942,-1.31037031610782,10.2077346253654));
#10957=CARTESIAN_POINT('Ctrl Pts',(10.0502525316942,-1.2845505698718,10.26401245069));
#10958=CARTESIAN_POINT('Ctrl Pts',(10.0502525316942,-1.2575411104082,10.3202191159745));
#10959=CARTESIAN_POINT('Ctrl Pts',(10.0502525316942,-1.22938873407215,10.3763394931394));
#10960=CARTESIAN_POINT('Ctrl Pts',(10.0502525316942,-1.20014382966931,10.4323597856746));
#10961=CARTESIAN_POINT('Ctrl Pts',(10.0502525316942,-1.16985259538408,10.4882691830915));
#10962=CARTESIAN_POINT('Ctrl Pts',(10.0502525316942,-1.13855017696687,10.5440612301269));
#10963=CARTESIAN_POINT('Ctrl Pts',(10.0502525316942,-1.10626216443499,10.599732595958));
#10964=CARTESIAN_POINT('Ctrl Pts',(10.0502525316942,-1.07965669109989,10.6441722372873));
#10965=CARTESIAN_POINT('Ctrl Pts',(10.0502525316942,-1.05927071468098,10.6774471807436));
#10966=CARTESIAN_POINT('Ctrl Pts',(10.0502525316942,-1.04548846715806,10.6996061707058));
#10967=CARTESIAN_POINT('Ctrl Pts',(10.0502525316942,-1.03854944428814,10.7106795892491));
#10968=CARTESIAN_POINT('',(10.0502525316942,0.205863042617261,9.15961421508102));
#10969=CARTESIAN_POINT('Ctrl Pts',(10.0502525316942,-1.03854944428814,10.7106795892491));
#10970=CARTESIAN_POINT('Ctrl Pts',(10.0502525316942,-1.00031843628634,10.7069087245865));
#10971=CARTESIAN_POINT('Ctrl Pts',(10.0502525316942,-0.926048534485518,
10.6988602462966));
#10972=CARTESIAN_POINT('Ctrl Pts',(10.0502525316942,-0.821220046750495,
10.6852672767501));
#10973=CARTESIAN_POINT('Ctrl Pts',(10.0502525316942,-0.694625083433484,
10.6640973524763));
#10974=CARTESIAN_POINT('Ctrl Pts',(10.0502525316942,-0.55833353757036,10.6325607057952));
#10975=CARTESIAN_POINT('Ctrl Pts',(10.0502525316942,-0.443722777305706,
10.596013814283));
#10976=CARTESIAN_POINT('Ctrl Pts',(10.0502525316942,-0.350069791437761,
10.5546263356355));
#10977=CARTESIAN_POINT('Ctrl Pts',(10.0502525316942,-0.275979784341796,
10.5087249476599));
#10978=CARTESIAN_POINT('Ctrl Pts',(10.0502525316942,-0.219218698708488,
10.4588324224655));
#10979=CARTESIAN_POINT('Ctrl Pts',(10.0502525316942,-0.176389733643622,
10.4057430679645));
#10980=CARTESIAN_POINT('Ctrl Pts',(10.0502525316942,-0.143293435954744,
10.3504388022425));
#10981=CARTESIAN_POINT('Ctrl Pts',(10.0502525316942,-0.115615100388501,
10.2939289512549));
#10982=CARTESIAN_POINT('Ctrl Pts',(10.0502525316942,-0.0895255103702565,
10.237110176256));
#10983=CARTESIAN_POINT('Ctrl Pts',(10.0502525316942,-0.0622734430034763,
10.1806284708027));
#10984=CARTESIAN_POINT('Ctrl Pts',(10.0502525316942,-0.032906007660544,
10.1247109492303));
#10985=CARTESIAN_POINT('Ctrl Pts',(10.0502525316942,-0.00188374052503792,
10.0692584999061));
#10986=CARTESIAN_POINT('Ctrl Pts',(10.0502525316942,0.0295176561224916,
10.0139888357391));
#10987=CARTESIAN_POINT('Ctrl Pts',(10.0502525316942,0.0597188954606688,
9.95855906844526));
#10988=CARTESIAN_POINT('Ctrl Pts',(10.0502525316942,0.0873927181594353,
9.90269886586131));
#10989=CARTESIAN_POINT('Ctrl Pts',(10.0502525316942,0.111969973727217,9.84633157004081));
#10990=CARTESIAN_POINT('Ctrl Pts',(10.0502525316942,0.133407037879775,9.78951336137147));
#10991=CARTESIAN_POINT('Ctrl Pts',(10.0502525316942,0.151980202759257,9.73237897573987));
#10992=CARTESIAN_POINT('Ctrl Pts',(10.0502525316942,0.168085081732296,9.67508881816964));
#10993=CARTESIAN_POINT('Ctrl Pts',(10.0502525316942,0.182008602623653,9.61776871087166));
#10994=CARTESIAN_POINT('Ctrl Pts',(10.0502525316942,0.193802962616848,9.56047634174856));
#10995=CARTESIAN_POINT('Ctrl Pts',(10.0502525316942,0.203384169996505,9.50322667013965));
#10996=CARTESIAN_POINT('Ctrl Pts',(10.0502525316942,0.210586047375026,9.44600537601646));
#10997=CARTESIAN_POINT('Ctrl Pts',(10.0502525316942,0.215226755929044,9.38878575682053));
#10998=CARTESIAN_POINT('Ctrl Pts',(10.0502525316942,0.217182662598509,9.33154666905179));
#10999=CARTESIAN_POINT('Ctrl Pts',(10.0502525316942,0.216396922881074,9.27427657522174));
#11000=CARTESIAN_POINT('Ctrl Pts',(10.0502525316942,0.213560366023699,9.2284309476721));
#11001=CARTESIAN_POINT('Ctrl Pts',(10.0502525316942,0.210193044269048,9.1940293375968));
#11002=CARTESIAN_POINT('Ctrl Pts',(10.0502525316942,0.207398059264382,9.1710872092551));
#11003=CARTESIAN_POINT('Ctrl Pts',(10.0502525316942,0.205863042617261,9.15961421508102));
#11004=CARTESIAN_POINT('',(10.0502525316942,1.38781479615277,9.05620683581208));
#11005=CARTESIAN_POINT('Origin',(10.0502525316942,0.,0.));
#11006=CARTESIAN_POINT('',(10.0502525316942,2.32206279789789,10.5073910450885));
#11007=CARTESIAN_POINT('Ctrl Pts',(10.0502525316942,1.38781479615277,9.05620683581208));
#11008=CARTESIAN_POINT('Ctrl Pts',(10.0502525316942,1.38842685041928,9.06714350898568));
#11009=CARTESIAN_POINT('Ctrl Pts',(10.0502525316942,1.38986102430324,9.08898459591562));
#11010=CARTESIAN_POINT('Ctrl Pts',(10.0502525316942,1.39264248006707,9.12164944850753));
#11011=CARTESIAN_POINT('Ctrl Pts',(10.0502525316942,1.39761376933417,9.16500867538789));
#11012=CARTESIAN_POINT('Ctrl Pts',(10.0502525316942,1.40595054425593,9.21887966989634));
#11013=CARTESIAN_POINT('Ctrl Pts',(10.0502525316942,1.41644161231465,9.27241152635132));
#11014=CARTESIAN_POINT('Ctrl Pts',(10.0502525316942,1.42913234409394,9.32558483941339));
#11015=CARTESIAN_POINT('Ctrl Pts',(10.0502525316942,1.44408281853422,9.37836940755697));
#11016=CARTESIAN_POINT('Ctrl Pts',(10.0502525316942,1.4613660046363,9.43072293720942));
#11017=CARTESIAN_POINT('Ctrl Pts',(10.0502525316942,1.48104540427845,9.48259965202034));
#11018=CARTESIAN_POINT('Ctrl Pts',(10.0502525316942,1.50315324111201,9.53395832441854));
#11019=CARTESIAN_POINT('Ctrl Pts',(10.0502525316942,1.52766939477237,9.58477015487067));
#11020=CARTESIAN_POINT('Ctrl Pts',(10.0502525316942,1.55449526669738,9.63502805143792));
#11021=CARTESIAN_POINT('Ctrl Pts',(10.0502525316942,1.5834404348547,9.68475210162498));
#11022=CARTESIAN_POINT('Ctrl Pts',(10.0502525316942,1.61426576023972,9.73397818528844));
#11023=CARTESIAN_POINT('Ctrl Pts',(10.0502525316942,1.64671853312854,9.78274900943559));
#11024=CARTESIAN_POINT('Ctrl Pts',(10.0502525316942,1.68056831017818,9.8311048104422));
#11025=CARTESIAN_POINT('Ctrl Pts',(10.0502525316942,1.71564646229066,9.87907328228115));
#11026=CARTESIAN_POINT('Ctrl Pts',(10.0502525316942,1.75187093905158,9.92666301240917));
#11027=CARTESIAN_POINT('Ctrl Pts',(10.0502525316942,1.78921666506164,9.97386991924375));
#11028=CARTESIAN_POINT('Ctrl Pts',(10.0502525316942,1.8276944743413,10.0206816495737));
#11029=CARTESIAN_POINT('Ctrl Pts',(10.0502525316942,1.86732763406234,10.0670826197184));
#11030=CARTESIAN_POINT('Ctrl Pts',(10.0502525316942,1.9081272454134,10.1130592286672));
#11031=CARTESIAN_POINT('Ctrl Pts',(10.0502525316942,1.95007408775204,10.1586038807877));
#11032=CARTESIAN_POINT('Ctrl Pts',(10.0502525316942,1.99313042494654,10.2037132140826));
#11033=CARTESIAN_POINT('Ctrl Pts',(10.0502525316942,2.03724707618484,10.2483873017624));
#11034=CARTESIAN_POINT('Ctrl Pts',(10.0502525316942,2.08237185550883,10.2926285935634));
#11035=CARTESIAN_POINT('Ctrl Pts',(10.0502525316942,2.12845748520948,10.3364410841241));
#11036=CARTESIAN_POINT('Ctrl Pts',(10.0502525316942,2.17546854490588,10.3798294947586));
#11037=CARTESIAN_POINT('Ctrl Pts',(10.0502525316942,2.22337966776441,10.4227985654164));
#11038=CARTESIAN_POINT('Ctrl Pts',(10.0502525316942,2.26241558094358,10.4568416324806));
#11039=CARTESIAN_POINT('Ctrl Pts',(10.0502525316942,2.29208631967267,10.4821883711236));
#11040=CARTESIAN_POINT('Ctrl Pts',(10.0502525316942,2.31204152046505,10.4990038742164));
#11041=CARTESIAN_POINT('Ctrl Pts',(10.0502525316942,2.32206279789789,10.5073910450885));
#11042=CARTESIAN_POINT('',(10.0502525316942,3.02626384252387,8.64769560732005));
#11043=CARTESIAN_POINT('Ctrl Pts',(10.0502525316942,2.32206279789789,10.5073910450885));
#11044=CARTESIAN_POINT('Ctrl Pts',(10.0502525316942,2.35725738591831,10.4919907084944));
#11045=CARTESIAN_POINT('Ctrl Pts',(10.0502525316942,2.42540514342016,10.4613854889436));
#11046=CARTESIAN_POINT('Ctrl Pts',(10.0502525316942,2.52090250118004,10.4160640224759));
#11047=CARTESIAN_POINT('Ctrl Pts',(10.0502525316942,2.63475959960257,10.3568102329785));
#11048=CARTESIAN_POINT('Ctrl Pts',(10.0502525316942,2.75463520264158,10.284700695789));
#11049=CARTESIAN_POINT('Ctrl Pts',(10.0502525316942,2.85234290245999,10.214525863806));
#11050=CARTESIAN_POINT('Ctrl Pts',(10.0502525316942,2.92862275068379,10.1462236683382));
#11051=CARTESIAN_POINT('Ctrl Pts',(10.0502525316942,2.98490222577489,10.0796737828909));
#11052=CARTESIAN_POINT('Ctrl Pts',(10.0502525316942,3.02346758796109,10.0146830316105));
#11053=CARTESIAN_POINT('Ctrl Pts',(10.0502525316942,3.04779484151101,9.95095717700994));
#11054=CARTESIAN_POINT('Ctrl Pts',(10.0502525316942,3.06218133312374,9.88813237627935));
#11055=CARTESIAN_POINT('Ctrl Pts',(10.0502525316942,3.07104249021943,9.82583523819669));
#11056=CARTESIAN_POINT('Ctrl Pts',(10.0502525316942,3.07829719773955,9.76373524529424));
#11057=CARTESIAN_POINT('Ctrl Pts',(10.0502525316942,3.08676164713489,9.70159659932322));
#11058=CARTESIAN_POINT('Ctrl Pts',(10.0502525316942,3.09741227343545,9.6393408394545));
#11059=CARTESIAN_POINT('Ctrl Pts',(10.0502525316942,3.10978045352404,9.57701601843134));
#11060=CARTESIAN_POINT('Ctrl Pts',(10.0502525316942,3.12256569092543,9.51474787896063));
#11061=CARTESIAN_POINT('Ctrl Pts',(10.0502525316942,3.13416003631015,9.45269834137241));
#11062=CARTESIAN_POINT('Ctrl Pts',(10.0502525316942,3.14321765381094,9.39102045019014));
#11063=CARTESIAN_POINT('Ctrl Pts',(10.0502525316942,3.14917356053584,9.32981717654858));
#11064=CARTESIAN_POINT('Ctrl Pts',(10.0502525316942,3.15200362801959,9.26915543181673));
#11065=CARTESIAN_POINT('Ctrl Pts',(10.0502525316942,3.15201226138312,9.2090779784702));
#11066=CARTESIAN_POINT('Ctrl Pts',(10.0502525316942,3.14962527917495,9.14961511949843));
#11067=CARTESIAN_POINT('Ctrl Pts',(10.0502525316942,3.14515444717397,9.09079785336099));
#11068=CARTESIAN_POINT('Ctrl Pts',(10.0502525316942,3.13866723439399,9.0326649146968));
#11069=CARTESIAN_POINT('Ctrl Pts',(10.0502525316942,3.13008838265685,8.97525648555044));
#11070=CARTESIAN_POINT('Ctrl Pts',(10.0502525316942,3.11925542274306,8.91861029840238));
#11071=CARTESIAN_POINT('Ctrl Pts',(10.0502525316942,3.10598716411038,8.86275714889703));
#11072=CARTESIAN_POINT('Ctrl Pts',(10.0502525316942,3.09015949103058,8.8077151330875));
#11073=CARTESIAN_POINT('Ctrl Pts',(10.0502525316942,3.07171477588927,8.75349084408744));
#11074=CARTESIAN_POINT('Ctrl Pts',(10.0502525316942,3.0548499719756,8.71076560553715));
#11075=CARTESIAN_POINT('Ctrl Pts',(10.0502525316942,3.04101677653125,8.67908828975171));
#11076=CARTESIAN_POINT('Ctrl Pts',(10.0502525316942,3.0312690802849,8.65813272696012));
#11077=CARTESIAN_POINT('Ctrl Pts',(10.0502525316942,3.02626384252387,8.64769560732005));
#11078=CARTESIAN_POINT('',(10.0502525316942,4.11841212213242,8.18410616705958));
#11079=CARTESIAN_POINT('Origin',(10.0502525316942,0.,0.));
#11080=CARTESIAN_POINT('',(10.0502525316942,5.45537535466284,9.2755658561365));
#11081=CARTESIAN_POINT('Ctrl Pts',(10.0502525316942,4.11841212213242,8.18410616705958));
#11082=CARTESIAN_POINT('Ctrl Pts',(10.0502525316942,4.12237383820348,8.19431842617809));
#11083=CARTESIAN_POINT('Ctrl Pts',(10.0502525316942,4.1304870856583,8.21464735012276));
#11084=CARTESIAN_POINT('Ctrl Pts',(10.0502525316942,4.14322640185693,8.24485395393398));
#11085=CARTESIAN_POINT('Ctrl Pts',(10.0502525316942,4.16135311687778,8.28455481633258));
#11086=CARTESIAN_POINT('Ctrl Pts',(10.0502525316942,4.18592891379899,8.33321297157003));
#11087=CARTESIAN_POINT('Ctrl Pts',(10.0502525316942,4.21244876582416,8.38088287416164));
#11088=CARTESIAN_POINT('Ctrl Pts',(10.0502525316942,4.24094982636281,8.42753204825146));
#11089=CARTESIAN_POINT('Ctrl Pts',(10.0502525316942,4.27147990109805,8.47311320506822));
#11090=CARTESIAN_POINT('Ctrl Pts',(10.0502525316942,4.3040953182409,8.51756357237276));
#11091=CARTESIAN_POINT('Ctrl Pts',(10.0502525316942,4.33884232599626,8.56081999110915));
#11092=CARTESIAN_POINT('Ctrl Pts',(10.0502525316942,4.37573883085758,8.60283329387128));
#11093=CARTESIAN_POINT('Ctrl Pts',(10.0502525316942,4.41475679767577,8.6435823082099));
#11094=CARTESIAN_POINT('Ctrl Pts',(10.0502525316942,4.45580026211617,8.68309075792173));
#11095=CARTESIAN_POINT('Ctrl Pts',(10.0502525316942,4.4986943294444,8.72143659100306));
#11096=CARTESIAN_POINT('Ctrl Pts',(10.0502525316942,4.54322265243728,8.75872782924178));
#11097=CARTESIAN_POINT('Ctrl Pts',(10.0502525316942,4.58915808705618,8.79508318101477));
#11098=CARTESIAN_POINT('Ctrl Pts',(10.0502525316942,4.63629390238203,8.83061212429863));
#11099=CARTESIAN_POINT('Ctrl Pts',(10.0502525316942,4.68447828052063,8.86539310688376));
#11100=CARTESIAN_POINT('Ctrl Pts',(10.0502525316942,4.73363584056076,8.89945965089929));
#11101=CARTESIAN_POINT('Ctrl Pts',(10.0502525316942,4.78374147310216,8.93281562325407));
#11102=CARTESIAN_POINT('Ctrl Pts',(10.0502525316942,4.83480166455838,8.96544592744964));
#11103=CARTESIAN_POINT('Ctrl Pts',(10.0502525316942,4.88683372770265,8.99732855257363));
#11104=CARTESIAN_POINT('Ctrl Pts',(10.0502525316942,4.93984401744929,9.02844713284016));
#11105=CARTESIAN_POINT('Ctrl Pts',(10.0502525316942,4.99381190670161,9.05880038387882));
#11106=CARTESIAN_POINT('Ctrl Pts',(10.0502525316942,5.04870046735128,9.08839676934597));
#11107=CARTESIAN_POINT('Ctrl Pts',(10.0502525316942,5.10446294828982,9.11725155657582));
#11108=CARTESIAN_POINT('Ctrl Pts',(10.0502525316942,5.16105047473192,9.14538320175401));
#11109=CARTESIAN_POINT('Ctrl Pts',(10.0502525316942,5.21841931731542,9.17281011362288));
#11110=CARTESIAN_POINT('Ctrl Pts',(10.0502525316942,5.27653724822262,9.19954772791879));
#11111=CARTESIAN_POINT('Ctrl Pts',(10.0502525316942,5.33538160688598,9.22560839138411));
#11112=CARTESIAN_POINT('Ctrl Pts',(10.0502525316942,5.38302685274804,9.24592251158686));
#11113=CARTESIAN_POINT('Ctrl Pts',(10.0502525316942,5.41907797515232,9.26085993003723));
#11114=CARTESIAN_POINT('Ctrl Pts',(10.0502525316942,5.44325277512453,9.27068592765741));
#11115=CARTESIAN_POINT('Ctrl Pts',(10.0502525316942,5.45537535466284,9.2755658561365));
#11116=CARTESIAN_POINT('',(10.0502525316942,5.55043285230422,7.28928030147641));
#11117=CARTESIAN_POINT('Ctrl Pts',(10.0502525316942,5.45537535466284,9.2755658561365));
#11118=CARTESIAN_POINT('Ctrl Pts',(10.0502525316942,5.48408843121132,9.25004353985723));
#11119=CARTESIAN_POINT('Ctrl Pts',(10.0502525316942,5.53944326709657,9.19987743117415));
#11120=CARTESIAN_POINT('Ctrl Pts',(10.0502525316942,5.61626154813455,9.12726384869626));
#11121=CARTESIAN_POINT('Ctrl Pts',(10.0502525316942,5.70623565557996,9.03572636773683));
#11122=CARTESIAN_POINT('Ctrl Pts',(10.0502525316942,5.79796105654696,8.93010252395574));
#11123=CARTESIAN_POINT('Ctrl Pts',(10.0502525316942,5.86920138549131,8.83316895299322));
#11124=CARTESIAN_POINT('Ctrl Pts',(10.0502525316942,5.92064129305387,8.74463793548674));
#11125=CARTESIAN_POINT('Ctrl Pts',(10.0502525316942,5.95360120899603,8.6639539190358));
#11126=CARTESIAN_POINT('Ctrl Pts',(10.0502525316942,5.97019580138365,8.59022668922188));
#11127=CARTESIAN_POINT('Ctrl Pts',(10.0502525316942,5.97364002234322,8.52210226517413));
#11128=CARTESIAN_POINT('Ctrl Pts',(10.0502525316942,5.96790845784416,8.4579066586566));
#11129=CARTESIAN_POINT('Ctrl Pts',(10.0502525316942,5.95708504467347,8.39592031140414));
#11130=CARTESIAN_POINT('Ctrl Pts',(10.0502525316942,5.94479472837688,8.33461788057945));
#11131=CARTESIAN_POINT('Ctrl Pts',(10.0502525316942,5.93364300051867,8.27290485770376));
#11132=CARTESIAN_POINT('Ctrl Pts',(10.0502525316942,5.92453426026728,8.2104048870761));
#11133=CARTESIAN_POINT('Ctrl Pts',(10.0502525316942,5.91703766966772,8.14730848207823));
#11134=CARTESIAN_POINT('Ctrl Pts',(10.0502525316942,5.90995523970613,8.08413710664289));
#11135=CARTESIAN_POINT('Ctrl Pts',(10.0502525316942,5.90180775582857,8.02154163982398));
#11136=CARTESIAN_POINT('Ctrl Pts',(10.0502525316942,5.89136254542228,7.96008352176745));
#11137=CARTESIAN_POINT('Ctrl Pts',(10.0502525316942,5.87811409765682,7.90003527315714));
#11138=CARTESIAN_POINT('Ctrl Pts',(10.0502525316942,5.86206014174823,7.84146798659238));
#11139=CARTESIAN_POINT('Ctrl Pts',(10.0502525316942,5.84350339850201,7.78432826524869));
#11140=CARTESIAN_POINT('Ctrl Pts',(10.0502525316942,5.82285820956226,7.72851334381365));
#11141=CARTESIAN_POINT('Ctrl Pts',(10.0502525316942,5.80043066085532,7.67395636265026));
#11142=CARTESIAN_POINT('Ctrl Pts',(10.0502525316942,5.77629688888814,7.62067331151744));
#11143=CARTESIAN_POINT('Ctrl Pts',(10.0502525316942,5.75039773581461,7.56872566186653));
#11144=CARTESIAN_POINT('Ctrl Pts',(10.0502525316942,5.72259034420254,7.51819950516883));
#11145=CARTESIAN_POINT('Ctrl Pts',(10.0502525316942,5.69271190798352,7.46918012077942));
#11146=CARTESIAN_POINT('Ctrl Pts',(10.0502525316942,5.66064997807339,7.42172307293681));
#11147=CARTESIAN_POINT('Ctrl Pts',(10.0502525316942,5.62635178473812,7.37585243997691));
#11148=CARTESIAN_POINT('Ctrl Pts',(10.0502525316942,5.59710957827922,7.34042983445952));
#11149=CARTESIAN_POINT('Ctrl Pts',(10.0502525316942,5.5741645986968,7.31457760934185));
#11150=CARTESIAN_POINT('Ctrl Pts',(10.0502525316942,5.55841836363355,7.2976598885924));
#11151=CARTESIAN_POINT('Ctrl Pts',(10.0502525316942,5.55043285230422,7.28928030147641));
#11152=CARTESIAN_POINT('',(10.0502525316942,6.44587057493322,6.51088816465466));
#11153=CARTESIAN_POINT('Origin',(10.0502525316942,0.,0.));
#11154=CARTESIAN_POINT('',(10.0502525316942,8.05467776187827,7.13578365451838));
#11155=CARTESIAN_POINT('Ctrl Pts',(10.0502525316942,6.44587057493322,6.51088816465466));
#11156=CARTESIAN_POINT('Ctrl Pts',(10.0502525316942,6.45279415243689,6.51937636264257));
#11157=CARTESIAN_POINT('Ctrl Pts',(10.0502525316942,6.46679229227336,6.5362031868863));
#11158=CARTESIAN_POINT('Ctrl Pts',(10.0502525316942,6.48824245587723,6.56099470907402));
#11159=CARTESIAN_POINT('Ctrl Pts',(10.0502525316942,6.51775022748935,6.59315100996711));
#11160=CARTESIAN_POINT('Ctrl Pts',(10.0502525316942,6.55615939617772,6.63183332667763));
#11161=CARTESIAN_POINT('Ctrl Pts',(10.0502525316942,6.59611208427845,6.66897501320444));
#11162=CARTESIAN_POINT('Ctrl Pts',(10.0502525316942,6.63763359119236,6.70453370213821));
#11163=CARTESIAN_POINT('Ctrl Pts',(10.0502525316942,6.68075476979194,6.73844964641633));
#11164=CARTESIAN_POINT('Ctrl Pts',(10.0502525316942,6.72550979370064,6.77064573971725));
#11165=CARTESIAN_POINT('Ctrl Pts',(10.0502525316942,6.77192313035347,6.801047622728));
#11166=CARTESIAN_POINT('Ctrl Pts',(10.0502525316942,6.81999661627367,6.82960300105583));
#11167=CARTESIAN_POINT('Ctrl Pts',(10.0502525316942,6.86969704580336,6.8563004018424));
#11168=CARTESIAN_POINT('Ctrl Pts',(10.0502525316942,6.92094048249309,6.88119204236944));
#11169=CARTESIAN_POINT('Ctrl Pts',(10.0502525316942,6.97358467882161,6.90440610103192));
#11170=CARTESIAN_POINT('Ctrl Pts',(10.0502525316942,7.02745725692073,6.92611216762375));
#11171=CARTESIAN_POINT('Ctrl Pts',(10.0502525316942,7.08237887287821,6.94649333188842));
#11172=CARTESIAN_POINT('Ctrl Pts',(10.0502525316942,7.13818674446165,6.96571759693621));
#11173=CARTESIAN_POINT('Ctrl Pts',(10.0502525316942,7.19476072597385,6.98390648535874));
#11174=CARTESIAN_POINT('Ctrl Pts',(10.0502525316942,7.25203948481561,7.00111517257795));
#11175=CARTESIAN_POINT('Ctrl Pts',(10.0502525316942,7.31000033546873,7.01735509547412));
#11176=CARTESIAN_POINT('Ctrl Pts',(10.0502525316942,7.36864478180451,7.032609892012));
#11177=CARTESIAN_POINT('Ctrl Pts',(10.0502525316942,7.42798248750274,7.0468532786288));
#11178=CARTESIAN_POINT('Ctrl Pts',(10.0502525316942,7.48801443914016,7.06006772676068));
#11179=CARTESIAN_POINT('Ctrl Pts',(10.0502525316942,7.54872062228975,7.07225838902223));
#11180=CARTESIAN_POINT('Ctrl Pts',(10.0502525316942,7.6100685316471,7.08344472624203));
#11181=CARTESIAN_POINT('Ctrl Pts',(10.0502525316942,7.67201842213158,7.09365570540476));
#11182=CARTESIAN_POINT('Ctrl Pts',(10.0502525316942,7.73452951433514,7.10292398252533));
#11183=CARTESIAN_POINT('Ctrl Pts',(10.0502525316942,7.7975659077772,7.11128057847415));
#11184=CARTESIAN_POINT('Ctrl Pts',(10.0502525316942,7.86110172188656,7.11875013245223));
#11185=CARTESIAN_POINT('Ctrl Pts',(10.0502525316942,7.92511922053603,7.12535138940982));
#11186=CARTESIAN_POINT('Ctrl Pts',(10.0502525316942,7.97670995045205,7.12994807512891));
#11187=CARTESIAN_POINT('Ctrl Pts',(10.0502525316942,8.01561252148766,7.13301399479354));
#11188=CARTESIAN_POINT('Ctrl Pts',(10.0502525316942,8.04164052278268,7.13488864983229));
#11189=CARTESIAN_POINT('Ctrl Pts',(10.0502525316942,8.05467776187827,7.13578365451838));
#11190=CARTESIAN_POINT('',(10.0502525316942,7.53128682236137,5.21733945232202));
#11191=CARTESIAN_POINT('Ctrl Pts',(10.0502525316942,8.05467776187827,7.13578365451838));
#11192=CARTESIAN_POINT('Ctrl Pts',(10.0502525316942,8.07409869096647,7.10263766069576));
#11193=CARTESIAN_POINT('Ctrl Pts',(10.0502525316942,8.11124208821886,7.03782127112617));
#11194=CARTESIAN_POINT('Ctrl Pts',(10.0502525316942,8.1618617839625,6.94502349601963));
#11195=CARTESIAN_POINT('Ctrl Pts',(10.0502525316942,8.21914560790756,6.83016265001357));
#11196=CARTESIAN_POINT('Ctrl Pts',(10.0502525316942,8.27374208546745,6.70136369739477));
#11197=CARTESIAN_POINT('Ctrl Pts',(10.0502525316942,8.31154154378012,6.58715992075444));
#11198=CARTESIAN_POINT('Ctrl Pts',(10.0502525316942,8.33310621412631,6.48706611403476));
#11199=CARTESIAN_POINT('Ctrl Pts',(10.0502525316942,8.33952022470187,6.40014588026893));
#11200=CARTESIAN_POINT('Ctrl Pts',(10.0502525316942,8.33251965296669,6.32489910686351));
#11201=CARTESIAN_POINT('Ctrl Pts',(10.0502525316942,8.31474369699109,6.25904460664515));
#11202=CARTESIAN_POINT('Ctrl Pts',(10.0502525316942,8.28945512184757,6.19976210758369));
#11203=CARTESIAN_POINT('Ctrl Pts',(10.0502525316942,8.26000660950279,6.1441542067148));
#11204=CARTESIAN_POINT('Ctrl Pts',(10.0502525316942,8.22937433118026,6.08965004701613));
#11205=CARTESIAN_POINT('Ctrl Pts',(10.0502525316942,8.19969803488993,6.03440354789477));
#11206=CARTESIAN_POINT('Ctrl Pts',(10.0502525316942,8.17172155504672,5.9777772990961));
#11207=CARTESIAN_POINT('Ctrl Pts',(10.0502525316942,8.1450940122787,5.92008562586321));
#11208=CARTESIAN_POINT('Ctrl Pts',(10.0502525316942,8.11883719254497,5.86219466883171));
#11209=CARTESIAN_POINT('Ctrl Pts',(10.0502525316942,8.09174541189393,5.80518055320261));
#11210=CARTESIAN_POINT('Ctrl Pts',(10.0502525316942,8.06281982355119,5.74995815707108));
#11211=CARTESIAN_POINT('Ctrl Pts',(10.0502525316942,8.03166387167001,5.69694287444675));
#11212=CARTESIAN_POINT('Ctrl Pts',(10.0502525316942,7.99829736542789,5.64620302012031));
#11213=CARTESIAN_POINT('Ctrl Pts',(10.0502525316942,7.96299170889331,5.59759426482043));
#11214=CARTESIAN_POINT('Ctrl Pts',(10.0502525316942,7.92610920815888,5.5508908343176));
#11215=CARTESIAN_POINT('Ctrl Pts',(10.0502525316942,7.88792030747535,5.50593455556538));
#11216=CARTESIAN_POINT('Ctrl Pts',(10.0502525316942,7.84850235807098,5.46271710825366));
#11217=CARTESIAN_POINT('Ctrl Pts',(10.0502525316942,7.80781809321391,5.42131523598658));
#11218=CARTESIAN_POINT('Ctrl Pts',(10.0502525316942,7.76575825114004,5.38185496199325));
#11219=CARTESIAN_POINT('Ctrl Pts',(10.0502525316942,7.72219434684711,5.34446770160195));
#11220=CARTESIAN_POINT('Ctrl Pts',(10.0502525316942,7.67703660519484,5.3092410482218));
#11221=CARTESIAN_POINT('Ctrl Pts',(10.0502525316942,7.63024227979884,5.27621420845565));
#11222=CARTESIAN_POINT('Ctrl Pts',(10.0502525316942,7.59148510170534,5.25156164740301));
#11223=CARTESIAN_POINT('Ctrl Pts',(10.0502525316942,7.56167435245346,5.23406510887067));
#11224=CARTESIAN_POINT('Ctrl Pts',(10.0502525316942,7.54147092977177,5.22284125454301));
#11225=CARTESIAN_POINT('Ctrl Pts',(10.0502525316942,7.53128682236137,5.21733945232202));
#11226=CARTESIAN_POINT('',(10.0502525316942,8.14236230483842,4.20033906466803));
#11227=CARTESIAN_POINT('Origin',(10.0502525316942,0.,0.));
#11228=CARTESIAN_POINT('',(10.0502525316942,9.86553218952113,4.2975012308678));
#11229=CARTESIAN_POINT('Ctrl Pts',(10.0502525316942,8.14236230483842,4.20033906466803));
#11230=CARTESIAN_POINT('Ctrl Pts',(10.0502525316942,8.15157001576925,4.20627231756552));
#11231=CARTESIAN_POINT('Ctrl Pts',(10.0502525316942,8.17008281252941,4.21794991531197));
#11232=CARTESIAN_POINT('Ctrl Pts',(10.0502525316942,8.1981441320729,4.23489958895177));
#11233=CARTESIAN_POINT('Ctrl Pts',(10.0502525316942,8.23614453399815,4.2563636455618));
#11234=CARTESIAN_POINT('Ctrl Pts',(10.0502525316942,8.28462731741005,4.28128362907022));
#11235=CARTESIAN_POINT('Ctrl Pts',(10.0502525316942,8.33410199410829,4.30426141247364));
#11236=CARTESIAN_POINT('Ctrl Pts',(10.0502525316942,8.38457953300338,4.32524888402656));
#11237=CARTESIAN_POINT('Ctrl Pts',(10.0502525316942,8.43607081406306,4.34417968683382));
#11238=CARTESIAN_POINT('Ctrl Pts',(10.0502525316942,8.48858451117083,4.36096992819547));
#11239=CARTESIAN_POINT('Ctrl Pts',(10.0502525316942,8.54212091594884,4.37554132734912));
#11240=CARTESIAN_POINT('Ctrl Pts',(10.0502525316942,8.59666561517837,4.38784358185488));
#11241=CARTESIAN_POINT('Ctrl Pts',(10.0502525316942,8.65218348309394,4.39787604148868));
#11242=CARTESIAN_POINT('Ctrl Pts',(10.0502525316942,8.70861082741579,4.4057143056259));
#11243=CARTESIAN_POINT('Ctrl Pts',(10.0502525316942,8.76585197201427,4.41152423606579));
#11244=CARTESIAN_POINT('Ctrl Pts',(10.0502525316942,8.82379538192297,4.41552038997767));
#11245=CARTESIAN_POINT('Ctrl Pts',(10.0502525316942,8.88232706878773,4.41793231637186));
#11246=CARTESIAN_POINT('Ctrl Pts',(10.0502525316942,8.94134413332185,4.41897009817738));
#11247=CARTESIAN_POINT('Ctrl Pts',(10.0502525316942,9.00076986272314,4.41878643730905));
#11248=CARTESIAN_POINT('Ctrl Pts',(10.0502525316942,9.06056297636652,4.41745276152696));
#11249=CARTESIAN_POINT('Ctrl Pts',(10.0502525316942,9.12070543323243,4.41498695816126));
#11250=CARTESIAN_POINT('Ctrl Pts',(10.0502525316942,9.18119360744053,4.4113730012699));
#11251=CARTESIAN_POINT('Ctrl Pts',(10.0502525316942,9.24202856762888,4.40658290745794));
#11252=CARTESIAN_POINT('Ctrl Pts',(10.0502525316942,9.3032058354636,4.40059970120156));
#11253=CARTESIAN_POINT('Ctrl Pts',(10.0502525316942,9.36470796833893,4.3934344677265));
#11254=CARTESIAN_POINT('Ctrl Pts',(10.0502525316942,9.42651006560004,4.38511576007207));
#11255=CARTESIAN_POINT('Ctrl Pts',(10.0502525316942,9.48858327871958,4.37568340938317));
#11256=CARTESIAN_POINT('Ctrl Pts',(10.0502525316942,9.55089891543934,4.36518107490567));
#11257=CARTESIAN_POINT('Ctrl Pts',(10.0502525316942,9.61343241834946,4.35364935309914));
#11258=CARTESIAN_POINT('Ctrl Pts',(10.0502525316942,9.67616678749592,4.34111967477257));
#11259=CARTESIAN_POINT('Ctrl Pts',(10.0502525316942,9.73909094732754,4.32761534819777));
#11260=CARTESIAN_POINT('Ctrl Pts',(10.0502525316942,9.78957710119959,4.31604464380801));
#11261=CARTESIAN_POINT('Ctrl Pts',(10.0502525316942,9.8275230661634,4.30693895110861));
#11262=CARTESIAN_POINT('Ctrl Pts',(10.0502525316942,9.85285646666673,4.30067875926925));
#11263=CARTESIAN_POINT('Ctrl Pts',(10.0502525316942,9.86553218952113,4.2975012308678));
#11264=CARTESIAN_POINT('',(10.0502525316942,8.77492596468499,2.63468906623289));
#11265=CARTESIAN_POINT('Ctrl Pts',(10.0502525316942,9.86553218952113,4.2975012308678));
#11266=CARTESIAN_POINT('Ctrl Pts',(10.0502525316942,9.87375991529634,4.25997612031891));
#11267=CARTESIAN_POINT('Ctrl Pts',(10.0502525316942,9.88905601939953,4.18685412967622));
#11268=CARTESIAN_POINT('Ctrl Pts',(10.0502525316942,9.9085221213413,4.08295585472858));
#11269=CARTESIAN_POINT('Ctrl Pts',(10.0502525316942,9.9275083219784,3.95601502356554));
#11270=CARTESIAN_POINT('Ctrl Pts',(10.0502525316942,9.93963159251159,3.81664870098642));
#11271=CARTESIAN_POINT('Ctrl Pts',(10.0502525316942,9.94029010584861,3.69635378003033));
#11272=CARTESIAN_POINT('Ctrl Pts',(10.0502525316942,9.92986863879505,3.59449506329373));
#11273=CARTESIAN_POINT('Ctrl Pts',(10.0502525316942,9.90910889595984,3.50984697030289));
#11274=CARTESIAN_POINT('Ctrl Pts',(10.0502525316942,9.87919842483915,3.44044633176199));
#11275=CARTESIAN_POINT('Ctrl Pts',(10.0502525316942,9.84194232635164,3.38330805268968));
#11276=CARTESIAN_POINT('Ctrl Pts',(10.0502525316942,9.79957216249457,3.3347416451379));
#11277=CARTESIAN_POINT('Ctrl Pts',(10.0502525316942,9.75438117654386,3.29095547943264));
#11278=CARTESIAN_POINT('Ctrl Pts',(10.0502525316942,9.70840543702524,3.24858483776411));
#11279=CARTESIAN_POINT('Ctrl Pts',(10.0502525316942,9.66310949495059,3.20521277465607));
#11280=CARTESIAN_POINT('Ctrl Pts',(10.0502525316942,9.61900380828622,3.16000321945709));
#11281=CARTESIAN_POINT('Ctrl Pts',(10.0502525316942,9.57585180276088,3.11336354092674));
#11282=CARTESIAN_POINT('Ctrl Pts',(10.0502525316942,9.53299079371256,3.06641977252332));
#11283=CARTESIAN_POINT('Ctrl Pts',(10.0502525316942,9.4896066485377,3.02056794696251));
#11284=CARTESIAN_POINT('Ctrl Pts',(10.0502525316942,9.44503212038191,2.97698682564639));
#11285=CARTESIAN_POINT('Ctrl Pts',(10.0502525316942,9.39901842603143,2.9361940142505));
#11286=CARTESIAN_POINT('Ctrl Pts',(10.0502525316942,9.35160551556488,2.89824836262921));
#11287=CARTESIAN_POINT('Ctrl Pts',(10.0502525316942,9.30300690939252,2.86292873701902));
#11288=CARTESIAN_POINT('Ctrl Pts',(10.0502525316942,9.25349741301079,2.82990845462794));
#11289=CARTESIAN_POINT('Ctrl Pts',(10.0502525316942,9.20328535602728,2.79895351207997));
#11290=CARTESIAN_POINT('Ctrl Pts',(10.0502525316942,9.15244173271444,2.77003209344587));
#11291=CARTESIAN_POINT('Ctrl Pts',(10.0502525316942,9.10095481538197,2.74322870228394));
#11292=CARTESIAN_POINT('Ctrl Pts',(10.0502525316942,9.04875963323664,2.71869695754935));
#11293=CARTESIAN_POINT('Ctrl Pts',(10.0502525316942,8.99577459934956,2.69660154669561));
#11294=CARTESIAN_POINT('Ctrl Pts',(10.0502525316942,8.94194140034058,2.67705351804929));
#11295=CARTESIAN_POINT('Ctrl Pts',(10.0502525316942,8.88723149748883,2.66010336866474));
#11296=CARTESIAN_POINT('Ctrl Pts',(10.0502525316942,8.84275317038967,2.64863401651716));
#11297=CARTESIAN_POINT('Ctrl Pts',(10.0502525316942,8.8089947353088,2.64120584766726));
#11298=CARTESIAN_POINT('Ctrl Pts',(10.0502525316942,8.78631177678628,2.63677452882418));
#11299=CARTESIAN_POINT('Ctrl Pts',(10.0502525316942,8.77492596468499,2.63468906623289));
#11300=CARTESIAN_POINT('',(10.0502525316942,9.041822881172,1.47863151154858));
#11301=CARTESIAN_POINT('Origin',(10.0502525316942,0.,0.));
#11302=CARTESIAN_POINT('',(10.0502525316942,10.7106795892491,1.03854944428815));
#11303=CARTESIAN_POINT('Ctrl Pts',(10.0502525316942,9.041822881172,1.47863151154858));
#11304=CARTESIAN_POINT('Ctrl Pts',(10.0502525316942,9.05241341063017,1.48142903122266));
#11305=CARTESIAN_POINT('Ctrl Pts',(10.0502525316942,9.0736287027809,1.48681431784179));
#11306=CARTESIAN_POINT('Ctrl Pts',(10.0502525316942,9.10555434079238,1.49426299078246));
#11307=CARTESIAN_POINT('Ctrl Pts',(10.0502525316942,9.14832762892595,1.50293375169959));
#11308=CARTESIAN_POINT('Ctrl Pts',(10.0502525316942,9.20213819442161,1.51165206039235));
#11309=CARTESIAN_POINT('Ctrl Pts',(10.0502525316942,9.25629193365179,1.51821671513724));
#11310=CARTESIAN_POINT('Ctrl Pts',(10.0502525316942,9.31078441132333,1.5225785693654));
#11311=CARTESIAN_POINT('Ctrl Pts',(10.0502525316942,9.36560546949212,1.52467115182437));
#11312=CARTESIAN_POINT('Ctrl Pts',(10.0502525316942,9.42073743324162,1.52441199543777));
#11313=CARTESIAN_POINT('Ctrl Pts',(10.0502525316942,9.47615638983506,1.52172656066024));
#11314=CARTESIAN_POINT('Ctrl Pts',(10.0502525316942,9.53183308717807,1.51657146095807));
#11315=CARTESIAN_POINT('Ctrl Pts',(10.0502525316942,9.58773391775221,1.50895693238989));
#11316=CARTESIAN_POINT('Ctrl Pts',(10.0502525316942,9.64382166809154,1.49897455623114));
#11317=CARTESIAN_POINT('Ctrl Pts',(10.0502525316942,9.70005659890418,1.48681164197681));
#11318=CARTESIAN_POINT('Ctrl Pts',(10.0502525316942,9.75639893594512,1.472706711821));
#11319=CARTESIAN_POINT('Ctrl Pts',(10.0502525316942,9.81281120439258,1.45691330418438));
#11320=CARTESIAN_POINT('Ctrl Pts',(10.0502525316942,9.86926046040473,1.43966301743384));
#11321=CARTESIAN_POINT('Ctrl Pts',(10.0502525316942,9.9257209332579,1.42112478528011));
#11322=CARTESIAN_POINT('Ctrl Pts',(10.0502525316942,9.98217543513636,1.40137929597453));
#11323=CARTESIAN_POINT('Ctrl Pts',(10.0502525316942,10.0386123354999,1.38044913636065));
#11324=CARTESIAN_POINT('Ctrl Pts',(10.0502525316942,10.0950232336429,1.3583201853205));
#11325=CARTESIAN_POINT('Ctrl Pts',(10.0502525316942,10.1514004985561,1.33496549883664));
#11326=CARTESIAN_POINT('Ctrl Pts',(10.0502525316942,10.2077346253654,1.31037031610782));
#11327=CARTESIAN_POINT('Ctrl Pts',(10.0502525316942,10.26401245069,1.2845505698718));
#11328=CARTESIAN_POINT('Ctrl Pts',(10.0502525316942,10.3202191159745,1.2575411104082));
#11329=CARTESIAN_POINT('Ctrl Pts',(10.0502525316942,10.3763394931394,1.22938873407215));
#11330=CARTESIAN_POINT('Ctrl Pts',(10.0502525316942,10.4323597856746,1.20014382966931));
#11331=CARTESIAN_POINT('Ctrl Pts',(10.0502525316942,10.4882691830915,1.16985259538409));
#11332=CARTESIAN_POINT('Ctrl Pts',(10.0502525316942,10.5440612301269,1.13855017696687));
#11333=CARTESIAN_POINT('Ctrl Pts',(10.0502525316942,10.599732595958,1.10626216443499));
#11334=CARTESIAN_POINT('Ctrl Pts',(10.0502525316942,10.6441722372873,1.07965669109989));
#11335=CARTESIAN_POINT('Ctrl Pts',(10.0502525316942,10.6774471807436,1.05927071468098));
#11336=CARTESIAN_POINT('Ctrl Pts',(10.0502525316942,10.6996061707058,1.04548846715806));
#11337=CARTESIAN_POINT('Ctrl Pts',(10.0502525316942,10.7106795892491,1.03854944428815));
#11338=CARTESIAN_POINT('',(10.0502525316942,9.15961421508102,-0.20586304261726));
#11339=CARTESIAN_POINT('Ctrl Pts',(10.0502525316942,10.7106795892491,1.03854944428815));
#11340=CARTESIAN_POINT('Ctrl Pts',(10.0502525316942,10.7069087245865,1.00031843628634));
#11341=CARTESIAN_POINT('Ctrl Pts',(10.0502525316942,10.6988602462966,0.926048534485519));
#11342=CARTESIAN_POINT('Ctrl Pts',(10.0502525316942,10.6852672767501,0.821220046750495));
#11343=CARTESIAN_POINT('Ctrl Pts',(10.0502525316942,10.6640973524763,0.694625083433485));
#11344=CARTESIAN_POINT('Ctrl Pts',(10.0502525316942,10.6325607057952,0.55833353757036));
#11345=CARTESIAN_POINT('Ctrl Pts',(10.0502525316942,10.596013814283,0.443722777305706));
#11346=CARTESIAN_POINT('Ctrl Pts',(10.0502525316942,10.5546263356355,0.350069791437762));
#11347=CARTESIAN_POINT('Ctrl Pts',(10.0502525316942,10.5087249476599,0.275979784341797));
#11348=CARTESIAN_POINT('Ctrl Pts',(10.0502525316942,10.4588324224655,0.219218698708488));
#11349=CARTESIAN_POINT('Ctrl Pts',(10.0502525316942,10.4057430679645,0.176389733643622));
#11350=CARTESIAN_POINT('Ctrl Pts',(10.0502525316942,10.3504388022425,0.143293435954745));
#11351=CARTESIAN_POINT('Ctrl Pts',(10.0502525316942,10.2939289512549,0.115615100388502));
#11352=CARTESIAN_POINT('Ctrl Pts',(10.0502525316942,10.237110176256,0.0895255103702571));
#11353=CARTESIAN_POINT('Ctrl Pts',(10.0502525316942,10.1806284708027,0.0622734430034769));
#11354=CARTESIAN_POINT('Ctrl Pts',(10.0502525316942,10.1247109492303,0.0329060076605447));
#11355=CARTESIAN_POINT('Ctrl Pts',(10.0502525316942,10.0692584999061,0.00188374052503854));
#11356=CARTESIAN_POINT('Ctrl Pts',(10.0502525316942,10.0139888357391,-0.0295176561224909));
#11357=CARTESIAN_POINT('Ctrl Pts',(10.0502525316942,9.95855906844526,-0.0597188954606682));
#11358=CARTESIAN_POINT('Ctrl Pts',(10.0502525316942,9.90269886586131,-0.0873927181594347));
#11359=CARTESIAN_POINT('Ctrl Pts',(10.0502525316942,9.84633157004081,-0.111969973727217));
#11360=CARTESIAN_POINT('Ctrl Pts',(10.0502525316942,9.78951336137147,-0.133407037879775));
#11361=CARTESIAN_POINT('Ctrl Pts',(10.0502525316942,9.73237897573987,-0.151980202759256));
#11362=CARTESIAN_POINT('Ctrl Pts',(10.0502525316942,9.67508881816964,-0.168085081732296));
#11363=CARTESIAN_POINT('Ctrl Pts',(10.0502525316942,9.61776871087166,-0.182008602623652));
#11364=CARTESIAN_POINT('Ctrl Pts',(10.0502525316942,9.56047634174856,-0.193802962616847));
#11365=CARTESIAN_POINT('Ctrl Pts',(10.0502525316942,9.50322667013965,-0.203384169996504));
#11366=CARTESIAN_POINT('Ctrl Pts',(10.0502525316942,9.44600537601646,-0.210586047375025));
#11367=CARTESIAN_POINT('Ctrl Pts',(10.0502525316942,9.38878575682053,-0.215226755929043));
#11368=CARTESIAN_POINT('Ctrl Pts',(10.0502525316942,9.33154666905179,-0.217182662598509));
#11369=CARTESIAN_POINT('Ctrl Pts',(10.0502525316942,9.27427657522174,-0.216396922881074));
#11370=CARTESIAN_POINT('Ctrl Pts',(10.0502525316942,9.2284309476721,-0.213560366023699));
#11371=CARTESIAN_POINT('Ctrl Pts',(10.0502525316942,9.1940293375968,-0.210193044269048));
#11372=CARTESIAN_POINT('Ctrl Pts',(10.0502525316942,9.1710872092551,-0.207398059264382));
#11373=CARTESIAN_POINT('Ctrl Pts',(10.0502525316942,9.15961421508102,-0.20586304261726));
#11374=CARTESIAN_POINT('',(10.0502525316942,9.05620683581208,-1.38781479615277));
#11375=CARTESIAN_POINT('Origin',(10.0502525316942,0.,0.));
#11376=CARTESIAN_POINT('',(10.0502525316942,10.5073910450885,-2.3220627978979));
#11377=CARTESIAN_POINT('Ctrl Pts',(10.0502525316942,9.05620683581208,-1.38781479615277));
#11378=CARTESIAN_POINT('Ctrl Pts',(10.0502525316942,9.06714350898568,-1.38842685041928));
#11379=CARTESIAN_POINT('Ctrl Pts',(10.0502525316942,9.08898459591562,-1.38986102430324));
#11380=CARTESIAN_POINT('Ctrl Pts',(10.0502525316942,9.12164944850753,-1.39264248006707));
#11381=CARTESIAN_POINT('Ctrl Pts',(10.0502525316942,9.16500867538789,-1.39761376933418));
#11382=CARTESIAN_POINT('Ctrl Pts',(10.0502525316942,9.21887966989633,-1.40595054425593));
#11383=CARTESIAN_POINT('Ctrl Pts',(10.0502525316942,9.27241152635132,-1.41644161231465));
#11384=CARTESIAN_POINT('Ctrl Pts',(10.0502525316942,9.32558483941339,-1.42913234409394));
#11385=CARTESIAN_POINT('Ctrl Pts',(10.0502525316942,9.37836940755697,-1.44408281853422));
#11386=CARTESIAN_POINT('Ctrl Pts',(10.0502525316942,9.43072293720942,-1.4613660046363));
#11387=CARTESIAN_POINT('Ctrl Pts',(10.0502525316942,9.48259965202034,-1.48104540427845));
#11388=CARTESIAN_POINT('Ctrl Pts',(10.0502525316942,9.53395832441854,-1.50315324111201));
#11389=CARTESIAN_POINT('Ctrl Pts',(10.0502525316942,9.58477015487067,-1.52766939477237));
#11390=CARTESIAN_POINT('Ctrl Pts',(10.0502525316942,9.63502805143792,-1.55449526669738));
#11391=CARTESIAN_POINT('Ctrl Pts',(10.0502525316942,9.68475210162498,-1.5834404348547));
#11392=CARTESIAN_POINT('Ctrl Pts',(10.0502525316942,9.73397818528844,-1.61426576023973));
#11393=CARTESIAN_POINT('Ctrl Pts',(10.0502525316942,9.78274900943559,-1.64671853312855));
#11394=CARTESIAN_POINT('Ctrl Pts',(10.0502525316942,9.8311048104422,-1.68056831017819));
#11395=CARTESIAN_POINT('Ctrl Pts',(10.0502525316942,9.87907328228114,-1.71564646229066));
#11396=CARTESIAN_POINT('Ctrl Pts',(10.0502525316942,9.92666301240917,-1.75187093905158));
#11397=CARTESIAN_POINT('Ctrl Pts',(10.0502525316942,9.97386991924375,-1.78921666506164));
#11398=CARTESIAN_POINT('Ctrl Pts',(10.0502525316942,10.0206816495736,-1.82769447434131));
#11399=CARTESIAN_POINT('Ctrl Pts',(10.0502525316942,10.0670826197184,-1.86732763406234));
#11400=CARTESIAN_POINT('Ctrl Pts',(10.0502525316942,10.1130592286672,-1.90812724541341));
#11401=CARTESIAN_POINT('Ctrl Pts',(10.0502525316942,10.1586038807877,-1.95007408775204));
#11402=CARTESIAN_POINT('Ctrl Pts',(10.0502525316942,10.2037132140826,-1.99313042494655));
#11403=CARTESIAN_POINT('Ctrl Pts',(10.0502525316942,10.2483873017624,-2.03724707618484));
#11404=CARTESIAN_POINT('Ctrl Pts',(10.0502525316942,10.2926285935634,-2.08237185550883));
#11405=CARTESIAN_POINT('Ctrl Pts',(10.0502525316942,10.3364410841241,-2.12845748520948));
#11406=CARTESIAN_POINT('Ctrl Pts',(10.0502525316942,10.3798294947586,-2.17546854490588));
#11407=CARTESIAN_POINT('Ctrl Pts',(10.0502525316942,10.4227985654164,-2.22337966776441));
#11408=CARTESIAN_POINT('Ctrl Pts',(10.0502525316942,10.4568416324806,-2.26241558094358));
#11409=CARTESIAN_POINT('Ctrl Pts',(10.0502525316942,10.4821883711236,-2.29208631967268));
#11410=CARTESIAN_POINT('Ctrl Pts',(10.0502525316942,10.4990038742164,-2.31204152046505));
#11411=CARTESIAN_POINT('Ctrl Pts',(10.0502525316942,10.5073910450885,-2.3220627978979));
#11412=CARTESIAN_POINT('Ctrl Pts',(10.0502525316942,10.5073910450885,-2.3220627978979));
#11413=CARTESIAN_POINT('Ctrl Pts',(10.0502525316942,10.4919907084944,-2.35725738591831));
#11414=CARTESIAN_POINT('Ctrl Pts',(10.0502525316942,10.4613854889436,-2.42540514342016));
#11415=CARTESIAN_POINT('Ctrl Pts',(10.0502525316942,10.4160640224759,-2.52090250118004));
#11416=CARTESIAN_POINT('Ctrl Pts',(10.0502525316942,10.3568102329785,-2.63475959960258));
#11417=CARTESIAN_POINT('Ctrl Pts',(10.0502525316942,10.284700695789,-2.75463520264159));
#11418=CARTESIAN_POINT('Ctrl Pts',(10.0502525316942,10.214525863806,-2.85234290245999));
#11419=CARTESIAN_POINT('Ctrl Pts',(10.0502525316942,10.1462236683382,-2.92862275068379));
#11420=CARTESIAN_POINT('Ctrl Pts',(10.0502525316942,10.0796737828909,-2.98490222577489));
#11421=CARTESIAN_POINT('Ctrl Pts',(10.0502525316942,10.0146830316105,-3.02346758796109));
#11422=CARTESIAN_POINT('Ctrl Pts',(10.0502525316942,9.95095717700994,-3.04779484151101));
#11423=CARTESIAN_POINT('Ctrl Pts',(10.0502525316942,9.88813237627935,-3.06218133312374));
#11424=CARTESIAN_POINT('Ctrl Pts',(10.0502525316942,9.82583523819669,-3.07104249021943));
#11425=CARTESIAN_POINT('Ctrl Pts',(10.0502525316942,9.76373524529424,-3.07829719773955));
#11426=CARTESIAN_POINT('Ctrl Pts',(10.0502525316942,9.70159659932322,-3.08676164713489));
#11427=CARTESIAN_POINT('Ctrl Pts',(10.0502525316942,9.6393408394545,-3.09741227343545));
#11428=CARTESIAN_POINT('Ctrl Pts',(10.0502525316942,9.57701601843134,-3.10978045352405));
#11429=CARTESIAN_POINT('Ctrl Pts',(10.0502525316942,9.51474787896063,-3.12256569092544));
#11430=CARTESIAN_POINT('Ctrl Pts',(10.0502525316942,9.45269834137241,-3.13416003631015));
#11431=CARTESIAN_POINT('Ctrl Pts',(10.0502525316942,9.39102045019014,-3.14321765381094));
#11432=CARTESIAN_POINT('Ctrl Pts',(10.0502525316942,9.32981717654858,-3.14917356053584));
#11433=CARTESIAN_POINT('Ctrl Pts',(10.0502525316942,9.26915543181673,-3.1520036280196));
#11434=CARTESIAN_POINT('Ctrl Pts',(10.0502525316942,9.2090779784702,-3.15201226138312));
#11435=CARTESIAN_POINT('Ctrl Pts',(10.0502525316942,9.14961511949843,-3.14962527917495));
#11436=CARTESIAN_POINT('Ctrl Pts',(10.0502525316942,9.09079785336098,-3.14515444717397));
#11437=CARTESIAN_POINT('Ctrl Pts',(10.0502525316942,9.0326649146968,-3.13866723439399));
#11438=CARTESIAN_POINT('Ctrl Pts',(10.0502525316942,8.97525648555044,-3.13008838265685));
#11439=CARTESIAN_POINT('Ctrl Pts',(10.0502525316942,8.91861029840238,-3.11925542274306));
#11440=CARTESIAN_POINT('Ctrl Pts',(10.0502525316942,8.86275714889703,-3.10598716411038));
#11441=CARTESIAN_POINT('Ctrl Pts',(10.0502525316942,8.8077151330875,-3.09015949103058));
#11442=CARTESIAN_POINT('Ctrl Pts',(10.0502525316942,8.75349084408744,-3.07171477588927));
#11443=CARTESIAN_POINT('Ctrl Pts',(10.0502525316942,8.71076560553715,-3.0548499719756));
#11444=CARTESIAN_POINT('Ctrl Pts',(10.0502525316942,8.67908828975171,-3.04101677653125));
#11445=CARTESIAN_POINT('Ctrl Pts',(10.0502525316942,8.65813272696012,-3.0312690802849));
#11446=CARTESIAN_POINT('Ctrl Pts',(10.0502525316942,8.64769560732005,-3.02626384252387));
#11447=CARTESIAN_POINT('Origin',(29.1,0.,0.));
#11448=CARTESIAN_POINT('',(29.35,6.525,7.99082036443648E-16));
#11449=CARTESIAN_POINT('',(29.1,6.275,-7.68465866464964E-16));
#11450=CARTESIAN_POINT('Origin',(29.35,0.,0.));
#11451=CARTESIAN_POINT('Origin',(29.35,6.025,0.));
#11452=CARTESIAN_POINT('',(29.35,9.5,-1.16341445918999E-15));
#11453=CARTESIAN_POINT('Origin',(29.35,0.,0.));
#11454=CARTESIAN_POINT('Origin',(29.1,0.,0.));
#11455=CARTESIAN_POINT('',(28.85,10.,1.22464679914735E-15));
#11456=CARTESIAN_POINT('',(29.1,9.75,1.19403062916867E-15));
#11457=CARTESIAN_POINT('',(28.85,-10.,-1.22464679914735E-15));
#11458=CARTESIAN_POINT('Origin',(28.85,0.,0.));
#11459=CARTESIAN_POINT('Origin',(28.85,0.,0.));
#11460=CARTESIAN_POINT('Origin',(25.175,0.,0.));
#11461=CARTESIAN_POINT('',(25.175,-10.,-1.22464679914735E-15));
#11462=CARTESIAN_POINT('',(21.,-10.,-1.22464679914735E-15));
#11463=CARTESIAN_POINT('',(25.175,-10.,-1.22464679914735E-15));
#11464=CARTESIAN_POINT('Origin',(21.,0.,0.));
#11465=CARTESIAN_POINT('Origin',(15.75,0.,0.));
#11466=CARTESIAN_POINT('',(14.657256909085,15.1882841634002,3.83755346941362));
#11467=CARTESIAN_POINT('',(15.8,14.2806055031745,2.18414382321291));
#11468=CARTESIAN_POINT('Ctrl Pts',(14.657256909085,15.1882841634002,3.83755346941362));
#11469=CARTESIAN_POINT('Ctrl Pts',(14.6761465353606,15.2204809626378,3.62787322776073));
#11470=CARTESIAN_POINT('Ctrl Pts',(14.7000757634306,15.250028813069,3.38542345093701));
#11471=CARTESIAN_POINT('Ctrl Pts',(14.7590833374976,15.2622828979219,3.01772165354622));
#11472=CARTESIAN_POINT('Ctrl Pts',(14.7853594609317,15.2539028616426,2.91067193741133));
#11473=CARTESIAN_POINT('Ctrl Pts',(14.8353557732887,15.2268021501321,2.76471831385531));
#11474=CARTESIAN_POINT('Ctrl Pts',(14.8603859823923,15.2082738029837,2.71637224456181));
#11475=CARTESIAN_POINT('Ctrl Pts',(14.9364214749741,15.1451099616486,2.60757230132236));
#11476=CARTESIAN_POINT('Ctrl Pts',(14.9903198942808,15.0921202332377,2.57646607024933));
#11477=CARTESIAN_POINT('Ctrl Pts',(15.1263879851351,14.9660446513584,2.44988270035784));
#11478=CARTESIAN_POINT('Ctrl Pts',(15.1678275509266,14.9286624842201,2.40426863543054));
#11479=CARTESIAN_POINT('Ctrl Pts',(15.2552258947253,14.8473025034558,2.32210737310919));
#11480=CARTESIAN_POINT('Ctrl Pts',(15.3550596759664,14.7532054284997,2.23331369045724));
#11481=CARTESIAN_POINT('Ctrl Pts',(15.6054597342241,14.494507028123,2.15739979472749));
#11482=CARTESIAN_POINT('Ctrl Pts',(15.7019486088056,14.3906763868982,2.15624789525753));
#11483=CARTESIAN_POINT('Ctrl Pts',(15.8,14.2806055031745,2.18414382321291));
#11484=CARTESIAN_POINT('',(15.8,13.6345795785203,4.77539710335946));
#11485=CARTESIAN_POINT('Ctrl Pts',(15.8,13.6345795785203,4.77539710335946));
#11486=CARTESIAN_POINT('Ctrl Pts',(15.7459792937635,13.6911731184475,4.78813278866882));
#11487=CARTESIAN_POINT('Ctrl Pts',(15.6927059160363,13.7497509471747,4.79279589805565));
#11488=CARTESIAN_POINT('Ctrl Pts',(15.5867247540199,13.8716787063213,4.78623681742322));
#11489=CARTESIAN_POINT('Ctrl Pts',(15.5350561720989,13.9340337592383,4.77448531899119));
#11490=CARTESIAN_POINT('Ctrl Pts',(15.4151906303965,14.0850539296161,4.72742125274313));
#11491=CARTESIAN_POINT('Ctrl Pts',(15.3214773869192,14.2091728778631,4.67408522803015));
#11492=CARTESIAN_POINT('Ctrl Pts',(15.0123014953173,14.6493868178153,4.37489871211529));
#11493=CARTESIAN_POINT('Ctrl Pts',(14.8382414780521,14.911826741515,4.14365161073496));
#11494=CARTESIAN_POINT('Ctrl Pts',(14.657256909085,15.1882841634002,3.83755346941362));
#11495=CARTESIAN_POINT('Origin',(15.8,0.,0.));
#11496=CARTESIAN_POINT('Origin',(15.75,0.,0.));
#11497=CARTESIAN_POINT('',(14.657256909085,13.2590473860729,8.34316815560344));
#11498=CARTESIAN_POINT('',(15.8,12.9067253609027,6.49019400603778));
#11499=CARTESIAN_POINT('Ctrl Pts',(14.657256909085,13.2590473860729,8.34316815560344));
#11500=CARTESIAN_POINT('Ctrl Pts',(14.6761465353607,13.3544631198478,8.15369975356842));
#11501=CARTESIAN_POINT('Ctrl Pts',(14.7000757634309,13.4574858968645,7.93224710137492));
#11502=CARTESIAN_POINT('Ctrl Pts',(14.7590833374989,13.5827663283719,7.58632863137928));
#11503=CARTESIAN_POINT('Ctrl Pts',(14.7853594609332,13.6078766217888,7.48192872766003));
#11504=CARTESIAN_POINT('Ctrl Pts',(14.8353557732894,13.6272044635794,7.33474400248666));
#11505=CARTESIAN_POINT('Ctrl Pts',(14.8603859823931,13.6245227153103,7.2830385841017));
#11506=CARTESIAN_POINT('Ctrl Pts',(14.9364214749747,13.5980713638623,7.16004498870931));
#11507=CARTESIAN_POINT('Ctrl Pts',(14.990319894283,13.5572874913918,7.11408647834175));
#11508=CARTESIAN_POINT('Ctrl Pts',(15.1263879851328,13.4764989002042,6.95473904218075));
#11509=CARTESIAN_POINT('Ctrl Pts',(15.1678275509254,13.4550418677986,6.89980576356338));
#11510=CARTESIAN_POINT('Ctrl Pts',(15.2552258947258,13.4030531542626,6.79652414292547));
#11511=CARTESIAN_POINT('Ctrl Pts',(15.3550596759664,13.3410002748942,6.68299873715169));
#11512=CARTESIAN_POINT('Ctrl Pts',(15.6054597342243,13.1184221593503,6.53085812980638));
#11513=CARTESIAN_POINT('Ctrl Pts',(15.7019486088058,13.0200293079344,6.4976771756342));
#11514=CARTESIAN_POINT('Ctrl Pts',(15.8,12.9067253609027,6.49019400603777));
#11515=CARTESIAN_POINT('',(15.8,11.4915768952696,8.7549893339674));
#11516=CARTESIAN_POINT('Ctrl Pts',(15.8,11.4915768952696,8.7549893339674));
#11517=CARTESIAN_POINT('Ctrl Pts',(15.7459792937636,11.5414650070019,8.78459005607964));
#11518=CARTESIAN_POINT('Ctrl Pts',(15.6927059160362,11.5957348526763,8.80712648121854));
#11519=CARTESIAN_POINT('Ctrl Pts',(15.58672475402,11.7137219099126,8.83856617450447));
#11520=CARTESIAN_POINT('Ctrl Pts',(15.5350561720991,11.776656502038,8.84665860638097));
#11521=CARTESIAN_POINT('Ctrl Pts',(15.4151906304017,11.9348288154563,8.84856581863247));
#11522=CARTESIAN_POINT('Ctrl Pts',(15.321477386924,12.0693546880299,8.83619510911057));
#11523=CARTESIAN_POINT('Ctrl Pts',(15.0123014953181,12.5804767420976,8.68768541216616));
#11524=CARTESIAN_POINT('Ctrl Pts',(14.8382414780511,12.9015312258979,8.54885474594821));
#11525=CARTESIAN_POINT('Ctrl Pts',(14.657256909085,13.2590473860729,8.34316815560344));
#11526=CARTESIAN_POINT('Origin',(15.8,0.,0.));
#11527=CARTESIAN_POINT('Origin',(15.75,0.,0.));
#11528=CARTESIAN_POINT('',(14.657256909085,10.0319226693815,12.0320954124521));
#11529=CARTESIAN_POINT('',(15.8,10.2694450138623,10.160938779711));
#11530=CARTESIAN_POINT('Ctrl Pts',(14.657256909085,10.0319226693815,12.0320954124521));
#11531=CARTESIAN_POINT('Ctrl Pts',(14.6761465353608,10.1812173808714,11.8813853373316));
#11532=CARTESIAN_POINT('Ctrl Pts',(14.7000757634311,10.3476304972585,11.7026071383166));
#11533=CARTESIAN_POINT('Ctrl Pts',(14.7590833374986,10.5736739539014,11.4123329057223));
#11534=CARTESIAN_POINT('Ctrl Pts',(14.7853594609326,10.6298166065432,11.3208022043886));
#11535=CARTESIAN_POINT('Ctrl Pts',(14.8353557732898,10.6936810578157,11.1867938439891));
#11536=CARTESIAN_POINT('Ctrl Pts',(14.8603859823935,10.7071084166316,11.1367903631164));
#11537=CARTESIAN_POINT('Ctrl Pts',(14.936421474975,10.719958797647,11.0116425856352));
#11538=CARTESIAN_POINT('Ctrl Pts',(14.9903198942818,10.6953729907149,10.9553305351824));
#11539=CARTESIAN_POINT('Ctrl Pts',(15.1263879851324,10.6677795404068,10.7788170700374));
#11540=CARTESIAN_POINT('Ctrl Pts',(15.1678275509255,10.6643480065665,10.719941829784));
#11541=CARTESIAN_POINT('Ctrl Pts',(15.255225894726,10.6468195777682,10.6056497754642));
#11542=CARTESIAN_POINT('Ctrl Pts',(15.3550596759663,10.6228850621673,10.4785053042637));
#11543=CARTESIAN_POINT('Ctrl Pts',(15.6054597342236,10.4582147281995,10.2650305679762));
#11544=CARTESIAN_POINT('Ctrl Pts',(15.7019486088043,10.3748910444333,10.2030685420815));
#11545=CARTESIAN_POINT('Ctrl Pts',(15.8,10.2694450138623,10.160938779711));
#11546=CARTESIAN_POINT('',(15.8,8.22369859898568,11.8775822089691));
#11547=CARTESIAN_POINT('Ctrl Pts',(15.8,8.22369859898568,11.8775822089691));
#11548=CARTESIAN_POINT('Ctrl Pts',(15.7459792937635,8.26199788655591,11.9211504429636));
#11549=CARTESIAN_POINT('Ctrl Pts',(15.6927059160359,8.30664743856279,11.9593541615416));
#11550=CARTESIAN_POINT('Ctrl Pts',(15.58672475402,8.4091443986622,12.0257150925135));
#11551=CARTESIAN_POINT('Ctrl Pts',(15.5350561720987,8.46649805362822,12.0528593110833));
#11552=CARTESIAN_POINT('Ctrl Pts',(15.4151906304096,8.61633950199434,12.1035511106054));
#11553=CARTESIAN_POINT('Ctrl Pts',(15.3214773869304,8.74810396918937,12.1333566475148));
#11554=CARTESIAN_POINT('Ctrl Pts',(15.0123014953204,9.2801019495249,12.1500609334098));
#11555=CARTESIAN_POINT('Ctrl Pts',(14.8382414780566,9.62834394362251,12.1172364152589));
#11556=CARTESIAN_POINT('Ctrl Pts',(14.657256909085,10.0319226693815,12.0320954124521));
#11557=CARTESIAN_POINT('Origin',(15.8,0.,0.));
#11558=CARTESIAN_POINT('Origin',(15.75,0.,0.));
#11559=CARTESIAN_POINT('',(14.657256909085,5.82280346529581,14.5432373377918));
#11560=CARTESIAN_POINT('',(15.8,6.62691983743441,12.8370600702028));
#11561=CARTESIAN_POINT('Ctrl Pts',(14.657256909085,5.82280346529581,14.5432373377918));
#11562=CARTESIAN_POINT('Ctrl Pts',(14.6761465353606,6.01136314794049,14.4460381417988));
#11563=CARTESIAN_POINT('Ctrl Pts',(14.7000757634306,6.2248769283947,14.3274344517058));
#11564=CARTESIAN_POINT('Ctrl Pts',(14.7590833374957,6.52955670169151,14.121218520862));
#11565=CARTESIAN_POINT('Ctrl Pts',(14.7853594609288,6.61123607955352,14.0515166846917));
#11566=CARTESIAN_POINT('Ctrl Pts',(14.8353557732898,6.7133856428566,13.9438023610666));
#11567=CARTESIAN_POINT('Ctrl Pts',(14.8603859823939,6.74160774532212,13.9003955068086));
#11568=CARTESIAN_POINT('Ctrl Pts',(14.9364214749747,6.79250197397385,13.7853438836539));
#11569=CARTESIAN_POINT('Ctrl Pts',(14.9903198942818,6.78652086266014,13.7241905089624));
#11570=CARTESIAN_POINT('Ctrl Pts',(15.1263879851336,6.81482359240408,13.547789382642));
#11571=CARTESIAN_POINT('Ctrl Pts',(15.167827550926,6.82975345957039,13.490735299478));
#11572=CARTESIAN_POINT('Ctrl Pts',(15.2552258947248,6.84840112024766,13.3766205140753));
#11573=CARTESIAN_POINT('Ctrl Pts',(15.355059675966,6.86492784556332,13.248302764155));
#11574=CARTESIAN_POINT('Ctrl Pts',(15.6054597342238,6.7742843727849,12.9943902934785));
#11575=CARTESIAN_POINT('Ctrl Pts',(15.7019486088051,6.71418615938417,12.9097124706704));
#11576=CARTESIAN_POINT('Ctrl Pts',(15.8,6.62691983743441,12.8370600702028));
#11577=CARTESIAN_POINT('',(15.8,4.15082738595568,13.8375145813754));
#11578=CARTESIAN_POINT('Ctrl Pts',(15.8,4.15082738595568,13.8375145813754));
#11579=CARTESIAN_POINT('Ctrl Pts',(15.7459792937636,4.17378884824957,13.8907855649509));
#11580=CARTESIAN_POINT('Ctrl Pts',(15.6927059160364,4.20444749734611,13.9409169308122));
#11581=CARTESIAN_POINT('Ctrl Pts',(15.5867247540198,4.28142124371676,14.0357032291837));
#11582=CARTESIAN_POINT('Ctrl Pts',(15.5350561720987,4.32757978616832,14.0792421692081));
#11583=CARTESIAN_POINT('Ctrl Pts',(15.4151906303927,4.4544228445381,14.1737564894865));
#11584=CARTESIAN_POINT('Ctrl Pts',(15.3214773869154,4.57052788225498,14.2428206991992));
#11585=CARTESIAN_POINT('Ctrl Pts',(15.0123014953169,5.07132611986995,14.4231038360399));
#11586=CARTESIAN_POINT('Ctrl Pts',(14.8382414780529,5.41266727154756,14.4994985584882));
#11587=CARTESIAN_POINT('Ctrl Pts',(14.657256909085,5.82280346529581,14.5432373377918));
#11588=CARTESIAN_POINT('Origin',(15.8,0.,0.));
#11589=CARTESIAN_POINT('Origin',(15.75,0.,0.));
#11590=CARTESIAN_POINT('',(14.657256909085,1.04370768816965,15.6307858638156));
#11591=CARTESIAN_POINT('',(15.8,2.33570557485288,14.2566004799664));
#11592=CARTESIAN_POINT('Ctrl Pts',(14.657256909085,1.04370768816965,15.6307858638156));
#11593=CARTESIAN_POINT('Ctrl Pts',(14.6761465353608,1.25307480646283,15.5966120814786));
#11594=CARTESIAN_POINT('Ctrl Pts',(14.7000757634309,1.49278903451672,15.5497926558526));
#11595=CARTESIAN_POINT('Ctrl Pts',(14.759083337499,1.84628094545359,15.4478208788453));
#11596=CARTESIAN_POINT('Ctrl Pts',(14.7853594609334,1.94550170192429,15.4067708092064));
#11597=CARTESIAN_POINT('Ctrl Pts',(14.8353557732896,2.07593726626537,15.3358943508599));
#11598=CARTESIAN_POINT('Ctrl Pts',(14.8603859823935,2.11619153635695,15.303333088545));
#11599=CARTESIAN_POINT('Ctrl Pts',(14.9364214749743,2.20014773094338,15.2096396742024));
#11600=CARTESIAN_POINT('Ctrl Pts',(14.990319894281,2.21335678809665,15.1496310936678));
#11601=CARTESIAN_POINT('Ctrl Pts',(15.1263879851348,2.29478522950975,14.9906096774748));
#11602=CARTESIAN_POINT('Ctrl Pts',(15.1678275509262,2.32661505826123,14.9409616025797));
#11603=CARTESIAN_POINT('Ctrl Pts',(15.2552258947253,2.37961344546108,14.838194436371));
#11604=CARTESIAN_POINT('Ctrl Pts',(15.3550596759664,2.43498366067059,14.7212640431372));
#11605=CARTESIAN_POINT('Ctrl Pts',(15.605459734224,2.42723986374774,14.4517685598142));
#11606=CARTESIAN_POINT('Ctrl Pts',(15.7019486088055,2.39624995256951,14.3526637953743));
#11607=CARTESIAN_POINT('Ctrl Pts',(15.8,2.33570557485288,14.2566004799664));
#11608=CARTESIAN_POINT('',(15.8,-0.328355732126619,14.4429346149236));
#11609=CARTESIAN_POINT('Ctrl Pts',(15.8,-0.328355732126618,14.4429346149236));
#11610=CARTESIAN_POINT('Ctrl Pts',(15.7459792937636,-0.322979723020242,
14.500693813047));
#11611=CARTESIAN_POINT('Ctrl Pts',(15.6927059160364,-0.309313059018563,
14.5578456188155));
#11612=CARTESIAN_POINT('Ctrl Pts',(15.5867247540198,-0.265397252979737,
14.6717789412865));
#11613=CARTESIAN_POINT('Ctrl Pts',(15.5350561720987,-0.234952142783135,
14.7274507079624));
#11614=CARTESIAN_POINT('Ctrl Pts',(15.4151906304043,-0.143523756760452,
14.8565358287886));
#11615=CARTESIAN_POINT('Ctrl Pts',(15.321477386926,-0.0544433185749542,
14.9580982252671));
#11616=CARTESIAN_POINT('Ctrl Pts',(15.012301495319,0.366133555586479,15.2843128435225));
#11617=CARTESIAN_POINT('Ctrl Pts',(14.8382414780528,0.667161014655142,15.4624487588678));
#11618=CARTESIAN_POINT('Ctrl Pts',(14.657256909085,1.04370768816965,15.6307858638156));
#11619=CARTESIAN_POINT('Origin',(15.8,0.,0.));
#11620=CARTESIAN_POINT('Origin',(15.75,0.,0.));
#11621=CARTESIAN_POINT('',(14.657256909085,-3.83755346941362,15.1882841634002));
#11622=CARTESIAN_POINT('',(15.8,-2.18414382321291,14.2806055031745));
#11623=CARTESIAN_POINT('Ctrl Pts',(14.657256909085,-3.83755346941362,15.1882841634002));
#11624=CARTESIAN_POINT('Ctrl Pts',(14.6761465353606,-3.62787322776029,15.2204809626379));
#11625=CARTESIAN_POINT('Ctrl Pts',(14.7000757634306,-3.38542345093672,15.2500288130691));
#11626=CARTESIAN_POINT('Ctrl Pts',(14.7590833374979,-3.01772165354433,15.2622828979219));
#11627=CARTESIAN_POINT('Ctrl Pts',(14.7853594609321,-2.91067193741018,15.2539028616423));
#11628=CARTESIAN_POINT('Ctrl Pts',(14.8353557732891,-2.76471831385429,15.226802150132));
#11629=CARTESIAN_POINT('Ctrl Pts',(14.8603859823928,-2.71637224456103,15.2082738029833));
#11630=CARTESIAN_POINT('Ctrl Pts',(14.9364214749744,-2.60757230132201,15.1451099616484));
#11631=CARTESIAN_POINT('Ctrl Pts',(14.9903198942815,-2.57646607024861,15.092120233237));
#11632=CARTESIAN_POINT('Ctrl Pts',(15.1263879851344,-2.44988270035848,14.9660446513591));
#11633=CARTESIAN_POINT('Ctrl Pts',(15.1678275509266,-2.4042686354305,14.9286624842201));
#11634=CARTESIAN_POINT('Ctrl Pts',(15.2552258947252,-2.32210737310926,14.8473025034559));
#11635=CARTESIAN_POINT('Ctrl Pts',(15.3550596759664,-2.23331369045724,14.7532054284997));
#11636=CARTESIAN_POINT('Ctrl Pts',(15.605459734224,-2.1573997947275,14.4945070281231));
#11637=CARTESIAN_POINT('Ctrl Pts',(15.7019486088056,-2.15624789525753,14.3906763868982));
#11638=CARTESIAN_POINT('Ctrl Pts',(15.8,-2.18414382321291,14.2806055031745));
#11639=CARTESIAN_POINT('',(15.8,-4.77539710335946,13.6345795785203));
#11640=CARTESIAN_POINT('Ctrl Pts',(15.8,-4.77539710335946,13.6345795785203));
#11641=CARTESIAN_POINT('Ctrl Pts',(15.7459792937632,-4.78813278866891,13.6911731184479));
#11642=CARTESIAN_POINT('Ctrl Pts',(15.692705916036,-4.79279589805564,13.749750947175));
#11643=CARTESIAN_POINT('Ctrl Pts',(15.5867247540198,-4.78623681742321,13.8716787063214));
#11644=CARTESIAN_POINT('Ctrl Pts',(15.5350561720987,-4.77448531899113,13.9340337592385));
#11645=CARTESIAN_POINT('Ctrl Pts',(15.4151906304068,-4.72742125274714,14.0850539296032));
#11646=CARTESIAN_POINT('Ctrl Pts',(15.3214773869283,-4.67408522803895,14.2091728778501));
#11647=CARTESIAN_POINT('Ctrl Pts',(15.0123014953194,-4.37489871211733,14.6493868178123));
#11648=CARTESIAN_POINT('Ctrl Pts',(14.8382414780541,-4.14365161073839,14.9118267415119));
#11649=CARTESIAN_POINT('Ctrl Pts',(14.657256909085,-3.83755346941362,15.1882841634002));
#11650=CARTESIAN_POINT('Origin',(15.8,0.,0.));
#11651=CARTESIAN_POINT('Origin',(15.75,0.,0.));
#11652=CARTESIAN_POINT('',(14.657256909085,-8.34316815560344,13.2590473860729));
#11653=CARTESIAN_POINT('',(15.8,-6.49019400603777,12.9067253609027));
#11654=CARTESIAN_POINT('Ctrl Pts',(14.657256909085,-8.34316815560344,13.2590473860729));
#11655=CARTESIAN_POINT('Ctrl Pts',(14.6761465353607,-8.15369975356933,13.3544631198474));
#11656=CARTESIAN_POINT('Ctrl Pts',(14.7000757634308,-7.93224710137545,13.4574858968644));
#11657=CARTESIAN_POINT('Ctrl Pts',(14.7590833374967,-7.58632863139194,13.5827663283673));
#11658=CARTESIAN_POINT('Ctrl Pts',(14.7853594609301,-7.48192872766908,13.6078766217876));
#11659=CARTESIAN_POINT('Ctrl Pts',(14.8353557732899,-7.33474400248519,13.6272044635796));
#11660=CARTESIAN_POINT('Ctrl Pts',(14.8603859823939,-7.28303858410022,13.62452271531));
#11661=CARTESIAN_POINT('Ctrl Pts',(14.9364214749749,-7.16004498870914,13.5980713638622));
#11662=CARTESIAN_POINT('Ctrl Pts',(14.9903198942826,-7.11408647834217,13.5572874913921));
#11663=CARTESIAN_POINT('Ctrl Pts',(15.1263879851326,-6.95473904218106,13.4764989002043));
#11664=CARTESIAN_POINT('Ctrl Pts',(15.1678275509258,-6.89980576356297,13.4550418677983));
#11665=CARTESIAN_POINT('Ctrl Pts',(15.2552258947243,-6.79652414292717,13.4030531542635));
#11666=CARTESIAN_POINT('Ctrl Pts',(15.3550596759657,-6.6829987371522,13.3410002748947));
#11667=CARTESIAN_POINT('Ctrl Pts',(15.6054597342234,-6.53085812980684,13.1184221593511));
#11668=CARTESIAN_POINT('Ctrl Pts',(15.7019486088045,-6.49767717563431,13.0200293079359));
#11669=CARTESIAN_POINT('Ctrl Pts',(15.8,-6.49019400603777,12.9067253609027));
#11670=CARTESIAN_POINT('',(15.8,-8.7549893339674,11.4915768952696));
#11671=CARTESIAN_POINT('Ctrl Pts',(15.8,-8.7549893339674,11.4915768952696));
#11672=CARTESIAN_POINT('Ctrl Pts',(15.7459792937626,-8.78459005608021,11.5414650070028));
#11673=CARTESIAN_POINT('Ctrl Pts',(15.6927059160353,-8.80712648121881,11.5957348526773));
#11674=CARTESIAN_POINT('Ctrl Pts',(15.5867247540199,-8.83856617450449,11.7137219099127));
#11675=CARTESIAN_POINT('Ctrl Pts',(15.5350561720989,-8.84665860638097,11.7766565020382));
#11676=CARTESIAN_POINT('Ctrl Pts',(15.4151906303964,-8.84856581863256,11.9348288154633));
#11677=CARTESIAN_POINT('Ctrl Pts',(15.3214773869192,-8.83619510910824,12.0693546880378));
#11678=CARTESIAN_POINT('Ctrl Pts',(15.0123014953169,-8.68768541216563,12.5804767420995));
#11679=CARTESIAN_POINT('Ctrl Pts',(14.8382414780509,-8.54885474594795,12.9015312258984));
#11680=CARTESIAN_POINT('Ctrl Pts',(14.657256909085,-8.34316815560344,13.2590473860729));
#11681=CARTESIAN_POINT('Origin',(15.8,0.,0.));
#11682=CARTESIAN_POINT('Origin',(15.75,0.,0.));
#11683=CARTESIAN_POINT('',(14.657256909085,-12.0320954124521,10.0319226693815));
#11684=CARTESIAN_POINT('',(15.8,-10.160938779711,10.2694450138623));
#11685=CARTESIAN_POINT('Ctrl Pts',(14.657256909085,-12.0320954124521,10.0319226693815));
#11686=CARTESIAN_POINT('Ctrl Pts',(14.6761465353606,-11.8813853373331,10.1812173808699));
#11687=CARTESIAN_POINT('Ctrl Pts',(14.7000757634307,-11.7026071383195,10.3476304972558));
#11688=CARTESIAN_POINT('Ctrl Pts',(14.7590833374962,-11.4123329057338,10.5736739538928));
#11689=CARTESIAN_POINT('Ctrl Pts',(14.7853594609295,-11.3208022043972,10.6298166065389));
#11690=CARTESIAN_POINT('Ctrl Pts',(14.8353557732893,-11.1867938439903,10.6936810578153));
#11691=CARTESIAN_POINT('Ctrl Pts',(14.860385982393,-11.1367903631174,10.7071084166315));
#11692=CARTESIAN_POINT('Ctrl Pts',(14.9364214749746,-11.0116425856357,10.7199587976471));
#11693=CARTESIAN_POINT('Ctrl Pts',(14.9903198942805,-10.9553305351842,10.6953729907151));
#11694=CARTESIAN_POINT('Ctrl Pts',(15.1263879851341,-10.7788170700351,10.6677795404065));
#11695=CARTESIAN_POINT('Ctrl Pts',(15.1678275509254,-10.719941829784,10.6643480065666));
#11696=CARTESIAN_POINT('Ctrl Pts',(15.2552258947242,-10.6056497754665,10.6468195777685));
#11697=CARTESIAN_POINT('Ctrl Pts',(15.3550596759655,-10.4785053042644,10.6228850621678));
#11698=CARTESIAN_POINT('Ctrl Pts',(15.605459734223,-10.2650305679767,10.4582147281999));
#11699=CARTESIAN_POINT('Ctrl Pts',(15.7019486088037,-10.2030685420817,10.3748910444339));
#11700=CARTESIAN_POINT('Ctrl Pts',(15.8,-10.160938779711,10.2694450138623));
#11701=CARTESIAN_POINT('',(15.8,-11.8775822089691,8.22369859898568));
#11702=CARTESIAN_POINT('Ctrl Pts',(15.8,-11.8775822089691,8.22369859898568));
#11703=CARTESIAN_POINT('Ctrl Pts',(15.7459792937652,-11.9211504429623,8.26199788655478));
#11704=CARTESIAN_POINT('Ctrl Pts',(15.6927059160382,-11.9593541615401,8.30664743856047));
#11705=CARTESIAN_POINT('Ctrl Pts',(15.5867247540197,-12.0257150925138,8.40914439866259));
#11706=CARTESIAN_POINT('Ctrl Pts',(15.5350561720987,-12.0528593110834,8.4664980536283));
#11707=CARTESIAN_POINT('Ctrl Pts',(15.4151906304064,-12.1035511106068,8.61633950199834));
#11708=CARTESIAN_POINT('Ctrl Pts',(15.321477386928,-12.1333566475149,8.74810396919347));
#11709=CARTESIAN_POINT('Ctrl Pts',(15.0123014953193,-12.1500609334098,9.28010194952675));
#11710=CARTESIAN_POINT('Ctrl Pts',(14.8382414780578,-12.1172364152594,9.62834394361986));
#11711=CARTESIAN_POINT('Ctrl Pts',(14.657256909085,-12.0320954124521,10.0319226693815));
#11712=CARTESIAN_POINT('Origin',(15.8,0.,0.));
#11713=CARTESIAN_POINT('Origin',(15.75,0.,0.));
#11714=CARTESIAN_POINT('',(14.657256909085,-14.5432373377918,5.82280346529581));
#11715=CARTESIAN_POINT('',(15.8,-12.8370600702028,6.62691983743441));
#11716=CARTESIAN_POINT('Ctrl Pts',(14.657256909085,-14.5432373377918,5.82280346529581));
#11717=CARTESIAN_POINT('Ctrl Pts',(14.6761465353606,-14.4460381417986,6.01136314794083));
#11718=CARTESIAN_POINT('Ctrl Pts',(14.7000757634306,-14.327434451706,6.22487692839421));
#11719=CARTESIAN_POINT('Ctrl Pts',(14.7590833374988,-14.1212185208509,6.52955670170803));
#11720=CARTESIAN_POINT('Ctrl Pts',(14.7853594609333,-14.0515166846818,6.61123607956297));
#11721=CARTESIAN_POINT('Ctrl Pts',(14.8353557732886,-13.9438023610692,6.71338564285407));
#11722=CARTESIAN_POINT('Ctrl Pts',(14.860385982392,-13.9003955068115,6.74160774532081));
#11723=CARTESIAN_POINT('Ctrl Pts',(14.9364214749746,-13.7853438836541,6.79250197397384));
#11724=CARTESIAN_POINT('Ctrl Pts',(14.9903198942818,-13.7241905089624,6.78652086266011));
#11725=CARTESIAN_POINT('Ctrl Pts',(15.1263879851336,-13.5477893826419,6.81482359240412));
#11726=CARTESIAN_POINT('Ctrl Pts',(15.167827550926,-13.490735299478,6.82975345957041));
#11727=CARTESIAN_POINT('Ctrl Pts',(15.2552258947255,-13.3766205140743,6.84840112024782));
#11728=CARTESIAN_POINT('Ctrl Pts',(15.3550596759663,-13.2483027641547,6.86492784556322));
#11729=CARTESIAN_POINT('Ctrl Pts',(15.6054597342241,-12.9943902934783,6.7742843727848));
#11730=CARTESIAN_POINT('Ctrl Pts',(15.7019486088055,-12.9097124706701,6.71418615938381));
#11731=CARTESIAN_POINT('Ctrl Pts',(15.8,-12.8370600702028,6.62691983743441));
#11732=CARTESIAN_POINT('',(15.8,-13.8375145813754,4.15082738595568));
#11733=CARTESIAN_POINT('Ctrl Pts',(15.8,-13.8375145813754,4.15082738595568));
#11734=CARTESIAN_POINT('Ctrl Pts',(15.7459792937635,-13.8907855649511,4.17378884824963));
#11735=CARTESIAN_POINT('Ctrl Pts',(15.6927059160365,-13.9409169308122,4.20444749734604));
#11736=CARTESIAN_POINT('Ctrl Pts',(15.5867247540197,-14.0357032291838,4.28142124371689));
#11737=CARTESIAN_POINT('Ctrl Pts',(15.5350561720985,-14.0792421692082,4.3275797861685));
#11738=CARTESIAN_POINT('Ctrl Pts',(15.4151906303655,-14.1737564895079,4.45442284456682));
#11739=CARTESIAN_POINT('Ctrl Pts',(15.3214773868911,-14.2428206992134,4.57052788229435));
#11740=CARTESIAN_POINT('Ctrl Pts',(15.0123014953115,-14.423103836043,5.07132611987859));
#11741=CARTESIAN_POINT('Ctrl Pts',(14.8382414780483,-14.4994985584893,5.41266727155799));
#11742=CARTESIAN_POINT('Ctrl Pts',(14.657256909085,-14.5432373377918,5.82280346529581));
#11743=CARTESIAN_POINT('Origin',(15.8,0.,0.));
#11744=CARTESIAN_POINT('Origin',(15.75,0.,0.));
#11745=CARTESIAN_POINT('',(14.657256909085,-15.6307858638156,1.04370768816965));
#11746=CARTESIAN_POINT('',(15.8,-14.2566004799664,2.33570557485288));
#11747=CARTESIAN_POINT('Ctrl Pts',(14.657256909085,-15.6307858638156,1.04370768816965));
#11748=CARTESIAN_POINT('Ctrl Pts',(14.6761465353606,-15.5966120814789,1.25307480646121));
#11749=CARTESIAN_POINT('Ctrl Pts',(14.7000757634306,-15.549792655853,1.49278903451451));
#11750=CARTESIAN_POINT('Ctrl Pts',(14.7590833374982,-15.4478208788467,1.84628094544931));
#11751=CARTESIAN_POINT('Ctrl Pts',(14.7853594609325,-15.4067708092076,1.94550170192191));
#11752=CARTESIAN_POINT('Ctrl Pts',(14.8353557732886,-15.3358943508614,2.07593726626272));
#11753=CARTESIAN_POINT('Ctrl Pts',(14.860385982392,-15.3033330885469,2.11619153635516));
#11754=CARTESIAN_POINT('Ctrl Pts',(14.9364214749742,-15.2096396742025,2.2001477309434));
#11755=CARTESIAN_POINT('Ctrl Pts',(14.9903198942811,-15.1496310936678,2.2133567880966));
#11756=CARTESIAN_POINT('Ctrl Pts',(15.126387985135,-14.9906096774745,2.29478522950994));
#11757=CARTESIAN_POINT('Ctrl Pts',(15.1678275509263,-14.9409616025796,2.32661505826135));
#11758=CARTESIAN_POINT('Ctrl Pts',(15.2552258947247,-14.8381944363718,2.37961344546068));
#11759=CARTESIAN_POINT('Ctrl Pts',(15.3550596759661,-14.7212640431375,2.43498366067061));
#11760=CARTESIAN_POINT('Ctrl Pts',(15.6054597342239,-14.4517685598143,2.42723986374774));
#11761=CARTESIAN_POINT('Ctrl Pts',(15.7019486088054,-14.3526637953743,2.39624995256956));
#11762=CARTESIAN_POINT('Ctrl Pts',(15.8,-14.2566004799664,2.33570557485288));
#11763=CARTESIAN_POINT('',(15.8,-14.4429346149236,-0.328355732126617));
#11764=CARTESIAN_POINT('Ctrl Pts',(15.8,-14.4429346149236,-0.328355732126619));
#11765=CARTESIAN_POINT('Ctrl Pts',(15.7459792937635,-14.5006938130472,-0.322979723020233));
#11766=CARTESIAN_POINT('Ctrl Pts',(15.6927059160363,-14.5578456188156,-0.309313059018514));
#11767=CARTESIAN_POINT('Ctrl Pts',(15.5867247540198,-14.6717789412865,-0.265397252979746));
#11768=CARTESIAN_POINT('Ctrl Pts',(15.5350561720988,-14.7274507079622,-0.234952142783211));
#11769=CARTESIAN_POINT('Ctrl Pts',(15.4151906304082,-14.8565358287844,-0.143523756763411));
#11770=CARTESIAN_POINT('Ctrl Pts',(15.3214773869296,-14.9580982252633,-0.05444331857987));
#11771=CARTESIAN_POINT('Ctrl Pts',(15.0123014953195,-15.2843128435219,0.366133555585719));
#11772=CARTESIAN_POINT('Ctrl Pts',(14.8382414780523,-15.4624487588682,0.667161014656064));
#11773=CARTESIAN_POINT('Ctrl Pts',(14.657256909085,-15.6307858638156,1.04370768816965));
#11774=CARTESIAN_POINT('Origin',(15.8,0.,0.));
#11775=CARTESIAN_POINT('Origin',(15.75,0.,0.));
#11776=CARTESIAN_POINT('',(14.657256909085,-15.1882841634002,-3.83755346941362));
#11777=CARTESIAN_POINT('',(15.8,-14.2806055031745,-2.18414382321291));
#11778=CARTESIAN_POINT('Ctrl Pts',(14.657256909085,-15.1882841634002,-3.83755346941362));
#11779=CARTESIAN_POINT('Ctrl Pts',(14.6761465353606,-15.2204809626379,-3.62787322776027));
#11780=CARTESIAN_POINT('Ctrl Pts',(14.7000757634307,-15.2500288130692,-3.38542345093602));
#11781=CARTESIAN_POINT('Ctrl Pts',(14.7590833374981,-15.2622828979219,-3.01772165354352));
#11782=CARTESIAN_POINT('Ctrl Pts',(14.7853594609323,-15.2539028616423,-2.91067193740946));
#11783=CARTESIAN_POINT('Ctrl Pts',(14.8353557732889,-15.226802150132,-2.76471831385505));
#11784=CARTESIAN_POINT('Ctrl Pts',(14.8603859823924,-15.2082738029837,-2.7163722445616));
#11785=CARTESIAN_POINT('Ctrl Pts',(14.9364214749744,-15.1451099616484,-2.60757230132212));
#11786=CARTESIAN_POINT('Ctrl Pts',(14.9903198942815,-15.092120233237,-2.5764660702486));
#11787=CARTESIAN_POINT('Ctrl Pts',(15.1263879851341,-14.9660446513593,-2.44988270035873));
#11788=CARTESIAN_POINT('Ctrl Pts',(15.1678275509262,-14.9286624842204,-2.40426863543085));
#11789=CARTESIAN_POINT('Ctrl Pts',(15.2552258947263,-14.8473025034548,-2.32210737310816));
#11790=CARTESIAN_POINT('Ctrl Pts',(15.3550596759668,-14.7532054284993,-2.23331369045709));
#11791=CARTESIAN_POINT('Ctrl Pts',(15.6054597342245,-14.4945070281226,-2.15739979472738));
#11792=CARTESIAN_POINT('Ctrl Pts',(15.7019486088061,-14.3906763868977,-2.15624789525766));
#11793=CARTESIAN_POINT('Ctrl Pts',(15.8,-14.2806055031745,-2.18414382321291));
#11794=CARTESIAN_POINT('',(15.8,-13.6345795785203,-4.77539710335946));
#11795=CARTESIAN_POINT('Ctrl Pts',(15.8,-13.6345795785203,-4.77539710335946));
#11796=CARTESIAN_POINT('Ctrl Pts',(15.7459792937634,-13.6911731184477,-4.78813278866886));
#11797=CARTESIAN_POINT('Ctrl Pts',(15.6927059160361,-13.7497509471749,-4.79279589805564));
#11798=CARTESIAN_POINT('Ctrl Pts',(15.5867247540198,-13.8716787063213,-4.78623681742322));
#11799=CARTESIAN_POINT('Ctrl Pts',(15.5350561720989,-13.9340337592383,-4.77448531899119));
#11800=CARTESIAN_POINT('Ctrl Pts',(15.4151906304075,-14.0850539296022,-4.72742125274744));
#11801=CARTESIAN_POINT('Ctrl Pts',(15.3214773869291,-14.2091728778489,-4.67408522803976));
#11802=CARTESIAN_POINT('Ctrl Pts',(15.0123014953194,-14.6493868178123,-4.3748987121173));
#11803=CARTESIAN_POINT('Ctrl Pts',(14.8382414780541,-14.911826741512,-4.14365161073832));
#11804=CARTESIAN_POINT('Ctrl Pts',(14.657256909085,-15.1882841634002,-3.83755346941362));
#11805=CARTESIAN_POINT('Origin',(15.8,0.,0.));
#11806=CARTESIAN_POINT('Origin',(15.75,0.,0.));
#11807=CARTESIAN_POINT('',(14.657256909085,-13.2590473860729,-8.34316815560344));
#11808=CARTESIAN_POINT('',(15.8,-12.9067253609027,-6.49019400603777));
#11809=CARTESIAN_POINT('Ctrl Pts',(14.657256909085,-13.2590473860729,-8.34316815560344));
#11810=CARTESIAN_POINT('Ctrl Pts',(14.6761465353605,-13.3544631198464,-8.15369975357118));
#11811=CARTESIAN_POINT('Ctrl Pts',(14.7000757634303,-13.4574858968621,-7.93224710138034));
#11812=CARTESIAN_POINT('Ctrl Pts',(14.7590833374966,-13.582766328368,-7.58632863139116));
#11813=CARTESIAN_POINT('Ctrl Pts',(14.7853594609306,-13.6078766217876,-7.48192872766814));
#11814=CARTESIAN_POINT('Ctrl Pts',(14.8353557732881,-13.6272044635792,-7.33474400249002));
#11815=CARTESIAN_POINT('Ctrl Pts',(14.8603859823915,-13.6245227153108,-7.28303858410438));
#11816=CARTESIAN_POINT('Ctrl Pts',(14.936421474974,-13.5980713638627,-7.16004498871016));
#11817=CARTESIAN_POINT('Ctrl Pts',(14.9903198942806,-13.5572874913932,-7.11408647834473));
#11818=CARTESIAN_POINT('Ctrl Pts',(15.1263879851354,-13.4764989002027,-6.95473904217766));
#11819=CARTESIAN_POINT('Ctrl Pts',(15.1678275509263,-13.455041867798,-6.89980576356226));
#11820=CARTESIAN_POINT('Ctrl Pts',(15.2552258947274,-13.4030531542616,-6.7965241429236));
#11821=CARTESIAN_POINT('Ctrl Pts',(15.3550596759675,-13.3410002748933,-6.68299873715091));
#11822=CARTESIAN_POINT('Ctrl Pts',(15.6054597342251,-13.1184221593495,-6.53085812980596));
#11823=CARTESIAN_POINT('Ctrl Pts',(15.7019486088073,-13.0200293079327,-6.49767717563406));
#11824=CARTESIAN_POINT('Ctrl Pts',(15.8,-12.9067253609027,-6.49019400603777));
#11825=CARTESIAN_POINT('',(15.8,-11.4915768952696,-8.7549893339674));
#11826=CARTESIAN_POINT('Ctrl Pts',(15.8,-11.4915768952696,-8.7549893339674));
#11827=CARTESIAN_POINT('Ctrl Pts',(15.7459792937642,-11.5414650070013,-8.78459005607929));
#11828=CARTESIAN_POINT('Ctrl Pts',(15.6927059160377,-11.5957348526747,-8.80712648121812));
#11829=CARTESIAN_POINT('Ctrl Pts',(15.5867247540194,-11.7137219099132,-8.83856617450462));
#11830=CARTESIAN_POINT('Ctrl Pts',(15.5350561720984,-11.7766565020389,-8.84665860638099));
#11831=CARTESIAN_POINT('Ctrl Pts',(15.4151906304178,-11.934828815435,-8.8485658186322));
#11832=CARTESIAN_POINT('Ctrl Pts',(15.321477386938,-12.0693546880067,-8.83619510911733));
#11833=CARTESIAN_POINT('Ctrl Pts',(15.0123014953219,-12.5804767420913,-8.68768541216795));
#11834=CARTESIAN_POINT('Ctrl Pts',(14.8382414780576,-12.9015312258851,-8.54885474595556));
#11835=CARTESIAN_POINT('Ctrl Pts',(14.657256909085,-13.2590473860729,-8.34316815560344));
#11836=CARTESIAN_POINT('Origin',(15.8,0.,0.));
#11837=CARTESIAN_POINT('Origin',(15.75,0.,0.));
#11838=CARTESIAN_POINT('',(14.657256909085,-10.0319226693815,-12.0320954124521));
#11839=CARTESIAN_POINT('',(15.8,-10.2694450138623,-10.160938779711));
#11840=CARTESIAN_POINT('Ctrl Pts',(14.657256909085,-10.0319226693815,-12.0320954124521));
#11841=CARTESIAN_POINT('Ctrl Pts',(14.6761465353604,-10.1812173808683,-11.8813853373348));
#11842=CARTESIAN_POINT('Ctrl Pts',(14.7000757634301,-10.3476304972515,-11.7026071383242));
#11843=CARTESIAN_POINT('Ctrl Pts',(14.7590833374954,-10.5736739538916,-11.412332905736));
#11844=CARTESIAN_POINT('Ctrl Pts',(14.7853594609291,-10.6298166065378,-11.3208022043988));
#11845=CARTESIAN_POINT('Ctrl Pts',(14.8353557732878,-10.693681057814,-11.1867938439937));
#11846=CARTESIAN_POINT('Ctrl Pts',(14.8603859823911,-10.7071084166306,-11.1367903631209));
#11847=CARTESIAN_POINT('Ctrl Pts',(14.9364214749739,-10.7199587976481,-11.0116425856358));
#11848=CARTESIAN_POINT('Ctrl Pts',(14.9903198942828,-10.695372990714,-10.9553305351818));
#11849=CARTESIAN_POINT('Ctrl Pts',(15.126387985135,-10.6677795404067,-10.7788170700337));
#11850=CARTESIAN_POINT('Ctrl Pts',(15.1678275509272,-10.6643480065664,-10.7199418297816));
#11851=CARTESIAN_POINT('Ctrl Pts',(15.2552258947223,-10.6468195777688,-10.6056497754691));
#11852=CARTESIAN_POINT('Ctrl Pts',(15.3550596759653,-10.6228850621681,-10.4785053042643));
#11853=CARTESIAN_POINT('Ctrl Pts',(15.6054597342239,-10.4582147281991,-10.2650305679761));
#11854=CARTESIAN_POINT('Ctrl Pts',(15.701948608806,-10.3748910444315,-10.2030685420807));
#11855=CARTESIAN_POINT('Ctrl Pts',(15.8,-10.2694450138623,-10.160938779711));
#11856=CARTESIAN_POINT('',(15.8,-8.22369859898568,-11.8775822089691));
#11857=CARTESIAN_POINT('Ctrl Pts',(15.8,-8.22369859898568,-11.8775822089691));
#11858=CARTESIAN_POINT('Ctrl Pts',(15.7459792937643,-8.26199788655536,-11.9211504429629));
#11859=CARTESIAN_POINT('Ctrl Pts',(15.6927059160378,-8.30664743856085,-11.9593541615403));
#11860=CARTESIAN_POINT('Ctrl Pts',(15.5867247540195,-8.40914439866277,-12.0257150925139));
#11861=CARTESIAN_POINT('Ctrl Pts',(15.5350561720988,-8.46649805362819,-12.0528593110833));
#11862=CARTESIAN_POINT('Ctrl Pts',(15.4151906304098,-8.616339501994,-12.1035511106053));
#11863=CARTESIAN_POINT('Ctrl Pts',(15.3214773869315,-8.74810396918746,-12.1333566475148));
#11864=CARTESIAN_POINT('Ctrl Pts',(15.0123014953196,-9.28010194952635,-12.1500609334098));
#11865=CARTESIAN_POINT('Ctrl Pts',(14.838241478058,-9.62834394361936,-12.1172364152595));
#11866=CARTESIAN_POINT('Ctrl Pts',(14.657256909085,-10.0319226693815,-12.0320954124521));
#11867=CARTESIAN_POINT('Origin',(15.8,0.,0.));
#11868=CARTESIAN_POINT('Origin',(15.75,0.,0.));
#11869=CARTESIAN_POINT('',(14.657256909085,-5.82280346529581,-14.5432373377918));
#11870=CARTESIAN_POINT('',(15.8,-6.62691983743441,-12.8370600702028));
#11871=CARTESIAN_POINT('Ctrl Pts',(14.657256909085,-5.82280346529581,-14.5432373377918));
#11872=CARTESIAN_POINT('Ctrl Pts',(14.6761465353607,-6.01136314794179,-14.4460381417981));
#11873=CARTESIAN_POINT('Ctrl Pts',(14.700075763431,-6.22487692839756,-14.3274344517042));
#11874=CARTESIAN_POINT('Ctrl Pts',(14.7590833374979,-6.52955670170211,-14.1212185208546));
#11875=CARTESIAN_POINT('Ctrl Pts',(14.7853594609316,-6.61123607955977,-14.0515166846853));
#11876=CARTESIAN_POINT('Ctrl Pts',(14.8353557732899,-6.71338564285629,-13.9438023610667));
#11877=CARTESIAN_POINT('Ctrl Pts',(14.8603859823937,-6.74160774532217,-13.9003955068088));
#11878=CARTESIAN_POINT('Ctrl Pts',(14.9364214749747,-6.79250197397347,-13.7853438836541));
#11879=CARTESIAN_POINT('Ctrl Pts',(14.9903198942808,-6.78652086266014,-13.7241905089635));
#11880=CARTESIAN_POINT('Ctrl Pts',(15.1263879851336,-6.81482359240397,-13.547789382642));
#11881=CARTESIAN_POINT('Ctrl Pts',(15.1678275509249,-6.82975345957013,-13.4907352994794));
#11882=CARTESIAN_POINT('Ctrl Pts',(15.2552258947256,-6.84840112024788,-13.3766205140742));
#11883=CARTESIAN_POINT('Ctrl Pts',(15.3550596759661,-6.8649278455632,-13.248302764155));
#11884=CARTESIAN_POINT('Ctrl Pts',(15.6054597342236,-6.77428437278503,-12.9943902934787));
#11885=CARTESIAN_POINT('Ctrl Pts',(15.7019486088046,-6.71418615938468,-12.9097124706708));
#11886=CARTESIAN_POINT('Ctrl Pts',(15.8,-6.62691983743441,-12.8370600702028));
#11887=CARTESIAN_POINT('',(15.8,-4.15082738595568,-13.8375145813754));
#11888=CARTESIAN_POINT('Ctrl Pts',(15.8,-4.15082738595568,-13.8375145813754));
#11889=CARTESIAN_POINT('Ctrl Pts',(15.7459792937636,-4.17378884824959,-13.890785564951));
#11890=CARTESIAN_POINT('Ctrl Pts',(15.6927059160362,-4.20444749734624,-13.9409169308124));
#11891=CARTESIAN_POINT('Ctrl Pts',(15.5867247540199,-4.28142124371671,-14.0357032291836));
#11892=CARTESIAN_POINT('Ctrl Pts',(15.5350561720989,-4.32757978616817,-14.079242169208));
#11893=CARTESIAN_POINT('Ctrl Pts',(15.415190630367,-4.45442284456523,-14.1737564895067));
#11894=CARTESIAN_POINT('Ctrl Pts',(15.3214773868927,-4.57052788229179,-14.2428206992125));
#11895=CARTESIAN_POINT('Ctrl Pts',(15.0123014953115,-5.07132611987859,-14.423103836043));
#11896=CARTESIAN_POINT('Ctrl Pts',(14.8382414780483,-5.41266727155799,-14.4994985584893));
#11897=CARTESIAN_POINT('Ctrl Pts',(14.657256909085,-5.82280346529581,-14.5432373377918));
#11898=CARTESIAN_POINT('Origin',(15.8,0.,0.));
#11899=CARTESIAN_POINT('Origin',(15.75,0.,0.));
#11900=CARTESIAN_POINT('',(14.657256909085,-1.04370768816965,-15.6307858638156));
#11901=CARTESIAN_POINT('',(15.8,-2.33570557485288,-14.2566004799664));
#11902=CARTESIAN_POINT('Ctrl Pts',(14.657256909085,-1.04370768816965,-15.6307858638156));
#11903=CARTESIAN_POINT('Ctrl Pts',(14.6761465353607,-1.25307480646202,-15.5966120814788));
#11904=CARTESIAN_POINT('Ctrl Pts',(14.7000757634309,-1.49278903451753,-15.5497926558525));
#11905=CARTESIAN_POINT('Ctrl Pts',(14.7590833374979,-1.84628094544666,-15.4478208788472));
#11906=CARTESIAN_POINT('Ctrl Pts',(14.7853594609317,-1.94550170192027,-15.4067708092087));
#11907=CARTESIAN_POINT('Ctrl Pts',(14.8353557732893,-2.07593726626439,-15.3358943508604));
#11908=CARTESIAN_POINT('Ctrl Pts',(14.8603859823929,-2.11619153635627,-15.3033330885458));
#11909=CARTESIAN_POINT('Ctrl Pts',(14.9364214749743,-2.20014773094341,-15.2096396742024));
#11910=CARTESIAN_POINT('Ctrl Pts',(14.9903198942815,-2.21335678809698,-15.1496310936672));
#11911=CARTESIAN_POINT('Ctrl Pts',(15.1263879851342,-2.29478522950942,-14.9906096774754));
#11912=CARTESIAN_POINT('Ctrl Pts',(15.1678275509262,-2.32661505826123,-14.9409616025797));
#11913=CARTESIAN_POINT('Ctrl Pts',(15.2552258947253,-2.37961344546106,-14.8381944363711));
#11914=CARTESIAN_POINT('Ctrl Pts',(15.3550596759663,-2.43498366067057,-14.7212640431373));
#11915=CARTESIAN_POINT('Ctrl Pts',(15.605459734224,-2.42723986374776,-14.4517685598143));
#11916=CARTESIAN_POINT('Ctrl Pts',(15.7019486088054,-2.39624995256959,-14.3526637953744));
#11917=CARTESIAN_POINT('Ctrl Pts',(15.8,-2.33570557485288,-14.2566004799664));
#11918=CARTESIAN_POINT('',(15.8,0.328355732126618,-14.4429346149236));
#11919=CARTESIAN_POINT('Ctrl Pts',(15.8,0.328355732126618,-14.4429346149236));
#11920=CARTESIAN_POINT('Ctrl Pts',(15.7459792937636,0.322979723020245,-14.500693813047));
#11921=CARTESIAN_POINT('Ctrl Pts',(15.6927059160364,0.309313059018548,-14.5578456188156));
#11922=CARTESIAN_POINT('Ctrl Pts',(15.5867247540199,0.265397252979768,-14.6717789412864));
#11923=CARTESIAN_POINT('Ctrl Pts',(15.5350561720989,0.234952142783248,-14.7274507079622));
#11924=CARTESIAN_POINT('Ctrl Pts',(15.4151906303863,0.143523756746709,-14.856535828808));
#11925=CARTESIAN_POINT('Ctrl Pts',(15.32147738691,0.0544433185531652,-14.958098225284));
#11926=CARTESIAN_POINT('Ctrl Pts',(15.0123014953153,-0.366133555591446,
-15.2843128435264));
#11927=CARTESIAN_POINT('Ctrl Pts',(14.8382414780483,-0.667161014664403,
-15.4624487588719));
#11928=CARTESIAN_POINT('Ctrl Pts',(14.657256909085,-1.04370768816965,-15.6307858638156));
#11929=CARTESIAN_POINT('Origin',(15.8,0.,0.));
#11930=CARTESIAN_POINT('Origin',(15.75,0.,0.));
#11931=CARTESIAN_POINT('',(14.657256909085,3.83755346941362,-15.1882841634002));
#11932=CARTESIAN_POINT('',(15.8,2.18414382321291,-14.2806055031745));
#11933=CARTESIAN_POINT('Ctrl Pts',(14.657256909085,3.83755346941362,-15.1882841634002));
#11934=CARTESIAN_POINT('Ctrl Pts',(14.6761465353607,3.62787322775964,-15.220480962638));
#11935=CARTESIAN_POINT('Ctrl Pts',(14.7000757634308,3.38542345093437,-15.2500288130694));
#11936=CARTESIAN_POINT('Ctrl Pts',(14.7590833374975,3.01772165354748,-15.2622828979217));
#11937=CARTESIAN_POINT('Ctrl Pts',(14.7853594609313,2.91067193741214,-15.2539028616428));
#11938=CARTESIAN_POINT('Ctrl Pts',(14.8353557732891,2.76471831385452,-15.2268021501319));
#11939=CARTESIAN_POINT('Ctrl Pts',(14.8603859823926,2.71637224456128,-15.2082738029835));
#11940=CARTESIAN_POINT('Ctrl Pts',(14.9364214749743,2.60757230132218,-15.1451099616485));
#11941=CARTESIAN_POINT('Ctrl Pts',(14.9903198942816,2.57646607024849,-15.0921202332369));
#11942=CARTESIAN_POINT('Ctrl Pts',(15.1263879851343,2.44988270035858,-14.9660446513592));
#11943=CARTESIAN_POINT('Ctrl Pts',(15.1678275509266,2.40426863543051,-14.9286624842201));
#11944=CARTESIAN_POINT('Ctrl Pts',(15.2552258947252,2.32210737310927,-14.8473025034559));
#11945=CARTESIAN_POINT('Ctrl Pts',(15.3550596759663,2.23331369045729,-14.7532054284997));
#11946=CARTESIAN_POINT('Ctrl Pts',(15.6054597342239,2.15739979472752,-14.4945070281232));
#11947=CARTESIAN_POINT('Ctrl Pts',(15.7019486088054,2.15624789525745,-14.3906763868985));
#11948=CARTESIAN_POINT('Ctrl Pts',(15.8,2.18414382321291,-14.2806055031745));
#11949=CARTESIAN_POINT('',(15.8,4.77539710335945,-13.6345795785203));
#11950=CARTESIAN_POINT('Ctrl Pts',(15.8,4.77539710335945,-13.6345795785203));
#11951=CARTESIAN_POINT('Ctrl Pts',(15.7459792937631,4.78813278866893,-13.691173118448));
#11952=CARTESIAN_POINT('Ctrl Pts',(15.6927059160355,4.7927958980556,-13.7497509471755));
#11953=CARTESIAN_POINT('Ctrl Pts',(15.58672475402,4.78623681742324,-13.8716787063212));
#11954=CARTESIAN_POINT('Ctrl Pts',(15.535056172099,4.77448531899122,-13.9340337592382));
#11955=CARTESIAN_POINT('Ctrl Pts',(15.4151906304118,4.7274212527491,-14.0850539295969));
#11956=CARTESIAN_POINT('Ctrl Pts',(15.3214773869328,4.67408522804331,-14.2091728778437));
#11957=CARTESIAN_POINT('Ctrl Pts',(15.0123014953203,4.37489871211817,-14.649386817811));
#11958=CARTESIAN_POINT('Ctrl Pts',(14.8382414780549,4.14365161073977,-14.9118267415107));
#11959=CARTESIAN_POINT('Ctrl Pts',(14.657256909085,3.83755346941362,-15.1882841634002));
#11960=CARTESIAN_POINT('Origin',(15.8,0.,0.));
#11961=CARTESIAN_POINT('Origin',(15.75,0.,0.));
#11962=CARTESIAN_POINT('',(14.657256909085,8.34316815560344,-13.2590473860729));
#11963=CARTESIAN_POINT('',(15.8,6.49019400603777,-12.9067253609027));
#11964=CARTESIAN_POINT('Ctrl Pts',(14.657256909085,8.34316815560344,-13.2590473860729));
#11965=CARTESIAN_POINT('Ctrl Pts',(14.6761465353606,8.15369975356969,-13.3544631198472));
#11966=CARTESIAN_POINT('Ctrl Pts',(14.7000757634305,7.93224710137849,-13.4574858968629));
#11967=CARTESIAN_POINT('Ctrl Pts',(14.7590833374994,7.58632863137506,-13.5827663283737));
#11968=CARTESIAN_POINT('Ctrl Pts',(14.7853594609344,7.48192872765686,-13.6078766217891));
#11969=CARTESIAN_POINT('Ctrl Pts',(14.8353557732885,7.33474400248902,-13.6272044635792));
#11970=CARTESIAN_POINT('Ctrl Pts',(14.860385982392,7.2830385841035,-13.6245227153106));
#11971=CARTESIAN_POINT('Ctrl Pts',(14.936421474974,7.16004498871036,-13.5980713638626));
#11972=CARTESIAN_POINT('Ctrl Pts',(14.99031989428,7.11408647834531,-13.5572874913936));
#11973=CARTESIAN_POINT('Ctrl Pts',(15.1263879851359,6.95473904217717,-13.4764989002024));
#11974=CARTESIAN_POINT('Ctrl Pts',(15.1678275509259,6.89980576356277,-13.4550418677983));
#11975=CARTESIAN_POINT('Ctrl Pts',(15.2552258947264,6.79652414292473,-13.4030531542622));
#11976=CARTESIAN_POINT('Ctrl Pts',(15.3550596759669,6.6829987371513,-13.3410002748937));
#11977=CARTESIAN_POINT('Ctrl Pts',(15.6054597342247,6.5308581298062,-13.1184221593499));
#11978=CARTESIAN_POINT('Ctrl Pts',(15.7019486088066,6.49767717563412,-13.0200293079335));
#11979=CARTESIAN_POINT('Ctrl Pts',(15.8,6.49019400603777,-12.9067253609027));
#11980=CARTESIAN_POINT('',(15.8,8.7549893339674,-11.4915768952696));
#11981=CARTESIAN_POINT('Ctrl Pts',(15.8,8.7549893339674,-11.4915768952696));
#11982=CARTESIAN_POINT('Ctrl Pts',(15.7459792937641,8.78459005607935,-11.5414650070014));
#11983=CARTESIAN_POINT('Ctrl Pts',(15.6927059160371,8.80712648121827,-11.5957348526753));
#11984=CARTESIAN_POINT('Ctrl Pts',(15.5867247540197,8.83856617450453,-11.7137219099129));
#11985=CARTESIAN_POINT('Ctrl Pts',(15.5350561720989,8.84665860638097,-11.7766565020382));
#11986=CARTESIAN_POINT('Ctrl Pts',(15.4151906304187,8.8485658186322,-11.9348288154339));
#11987=CARTESIAN_POINT('Ctrl Pts',(15.3214773869393,8.83619510911792,-12.0693546880046));
#11988=CARTESIAN_POINT('Ctrl Pts',(15.0123014953214,8.6876854121677,-12.5804767420922));
#11989=CARTESIAN_POINT('Ctrl Pts',(14.8382414780552,8.54885474595289,-12.9015312258898));
#11990=CARTESIAN_POINT('Ctrl Pts',(14.657256909085,8.34316815560344,-13.2590473860729));
#11991=CARTESIAN_POINT('Origin',(15.8,0.,0.));
#11992=CARTESIAN_POINT('Origin',(15.75,0.,0.));
#11993=CARTESIAN_POINT('',(14.657256909085,12.0320954124521,-10.0319226693815));
#11994=CARTESIAN_POINT('',(15.8,10.160938779711,-10.2694450138623));
#11995=CARTESIAN_POINT('Ctrl Pts',(14.657256909085,12.0320954124521,-10.0319226693815));
#11996=CARTESIAN_POINT('Ctrl Pts',(14.6761465353605,11.881385337334,-10.181217380869));
#11997=CARTESIAN_POINT('Ctrl Pts',(14.7000757634302,11.7026071383233,-10.3476304972523));
#11998=CARTESIAN_POINT('Ctrl Pts',(14.759083337498,11.4123329057235,-10.5736739539013));
#11999=CARTESIAN_POINT('Ctrl Pts',(14.7853594609327,11.320802204389,-10.6298166065426));
#12000=CARTESIAN_POINT('Ctrl Pts',(14.8353557732875,11.1867938439948,-10.6936810578134));
#12001=CARTESIAN_POINT('Ctrl Pts',(14.8603859823904,11.1367903631218,-10.7071084166307));
#12002=CARTESIAN_POINT('Ctrl Pts',(14.9364214749737,11.0116425856365,-10.7199587976476));
#12003=CARTESIAN_POINT('Ctrl Pts',(14.9903198942803,10.9553305351849,-10.6953729907148));
#12004=CARTESIAN_POINT('Ctrl Pts',(15.1263879851363,10.7788170700321,-10.6677795404063));
#12005=CARTESIAN_POINT('Ctrl Pts',(15.1678275509267,10.7199418297822,-10.6643480065664));
#12006=CARTESIAN_POINT('Ctrl Pts',(15.2552258947248,10.6056497754659,-10.6468195777683));
#12007=CARTESIAN_POINT('Ctrl Pts',(15.3550596759664,10.4785053042635,-10.6228850621674));
#12008=CARTESIAN_POINT('Ctrl Pts',(15.6054597342242,10.2650305679759,-10.4582147281989));
#12009=CARTESIAN_POINT('Ctrl Pts',(15.7019486088058,10.2030685420808,-10.3748910444316));
#12010=CARTESIAN_POINT('Ctrl Pts',(15.8,10.160938779711,-10.2694450138623));
#12011=CARTESIAN_POINT('',(15.8,11.8775822089691,-8.22369859898568));
#12012=CARTESIAN_POINT('Ctrl Pts',(15.8,11.8775822089691,-8.22369859898568));
#12013=CARTESIAN_POINT('Ctrl Pts',(15.7459792937641,11.9211504429631,-8.26199788655548));
#12014=CARTESIAN_POINT('Ctrl Pts',(15.6927059160372,11.9593541615407,-8.30664743856149));
#12015=CARTESIAN_POINT('Ctrl Pts',(15.5867247540198,12.0257150925137,-8.40914439866246));
#12016=CARTESIAN_POINT('Ctrl Pts',(15.535056172099,12.0528593110832,-8.46649805362797));
#12017=CARTESIAN_POINT('Ctrl Pts',(15.4151906304144,12.1035511106034,-8.61633950198822));
#12018=CARTESIAN_POINT('Ctrl Pts',(15.3214773869356,12.1333566475145,-8.74810396918045));
#12019=CARTESIAN_POINT('Ctrl Pts',(15.0123014953203,12.1500609334098,-9.28010194952505));
#12020=CARTESIAN_POINT('Ctrl Pts',(14.8382414780551,12.1172364152582,-9.62834394362577));
#12021=CARTESIAN_POINT('Ctrl Pts',(14.657256909085,12.0320954124521,-10.0319226693815));
#12022=CARTESIAN_POINT('Origin',(15.8,0.,0.));
#12023=CARTESIAN_POINT('Origin',(15.75,0.,0.));
#12024=CARTESIAN_POINT('',(14.657256909085,14.5432373377918,-5.82280346529581));
#12025=CARTESIAN_POINT('',(15.8,12.8370600702028,-6.62691983743441));
#12026=CARTESIAN_POINT('Ctrl Pts',(14.657256909085,14.5432373377918,-5.82280346529581));
#12027=CARTESIAN_POINT('Ctrl Pts',(14.6761465353606,14.4460381417986,-6.01136314794077));
#12028=CARTESIAN_POINT('Ctrl Pts',(14.7000757634307,14.3274344517053,-6.22487692839559));
#12029=CARTESIAN_POINT('Ctrl Pts',(14.7590833374967,14.1212185208583,-6.52955670169685));
#12030=CARTESIAN_POINT('Ctrl Pts',(14.7853594609302,14.0515166846884,-6.6112360795567));
#12031=CARTESIAN_POINT('Ctrl Pts',(14.8353557732895,13.9438023610675,-6.7133856428557));
#12032=CARTESIAN_POINT('Ctrl Pts',(14.8603859823933,13.9003955068096,-6.74160774532172));
#12033=CARTESIAN_POINT('Ctrl Pts',(14.9364214749747,13.7853438836539,-6.7925019739738));
#12034=CARTESIAN_POINT('Ctrl Pts',(14.9903198942819,13.7241905089622,-6.78652086266021));
#12035=CARTESIAN_POINT('Ctrl Pts',(15.1263879851332,13.5477893826425,-6.81482359240399));
#12036=CARTESIAN_POINT('Ctrl Pts',(15.1678275509259,13.4907352994781,-6.82975345957037));
#12037=CARTESIAN_POINT('Ctrl Pts',(15.2552258947254,13.3766205140745,-6.8484011202478));
#12038=CARTESIAN_POINT('Ctrl Pts',(15.3550596759662,13.2483027641548,-6.86492784556321));
#12039=CARTESIAN_POINT('Ctrl Pts',(15.6054597342237,12.9943902934786,-6.77428437278497));
#12040=CARTESIAN_POINT('Ctrl Pts',(15.7019486088047,12.9097124706706,-6.71418615938453));
#12041=CARTESIAN_POINT('Ctrl Pts',(15.8,12.8370600702028,-6.62691983743441));
#12042=CARTESIAN_POINT('',(15.8,13.8375145813754,-4.15082738595569));
#12043=CARTESIAN_POINT('Ctrl Pts',(15.8,13.8375145813754,-4.15082738595568));
#12044=CARTESIAN_POINT('Ctrl Pts',(15.7459792937632,13.8907855649513,-4.17378884824973));
#12045=CARTESIAN_POINT('Ctrl Pts',(15.6927059160362,13.9409169308123,-4.2044474973462));
#12046=CARTESIAN_POINT('Ctrl Pts',(15.5867247540197,14.0357032291838,-4.28142124371687));
#12047=CARTESIAN_POINT('Ctrl Pts',(15.5350561720987,14.0792421692081,-4.32757978616837));
#12048=CARTESIAN_POINT('Ctrl Pts',(15.41519063041,14.1737564894728,-4.45442284451972));
#12049=CARTESIAN_POINT('Ctrl Pts',(15.3214773869312,14.24282069919,-4.57052788222937));
#12050=CARTESIAN_POINT('Ctrl Pts',(15.01230149532,14.423103836038,-5.07132611986488));
#12051=CARTESIAN_POINT('Ctrl Pts',(14.8382414780537,14.499498558488,-5.4126672715457));
#12052=CARTESIAN_POINT('Ctrl Pts',(14.657256909085,14.5432373377918,-5.82280346529581));
#12053=CARTESIAN_POINT('Origin',(15.8,0.,0.));
#12054=CARTESIAN_POINT('Origin',(15.75,0.,0.));
#12055=CARTESIAN_POINT('',(15.8218384638272,-14.4233723052509,1.76635367265361E-15));
#12056=CARTESIAN_POINT('Origin',(15.8218384638272,0.,0.));
#12057=CARTESIAN_POINT('',(19.5,-10.5,-1.28587913910472E-15));
#12058=CARTESIAN_POINT('',(15.75,-14.5,-1.77573785876366E-15));
#12059=CARTESIAN_POINT('Origin',(19.5,0.,0.));
#12060=CARTESIAN_POINT('Origin',(21.25,0.,0.));
#12061=CARTESIAN_POINT('',(21.,-10.5,-1.28587913910472E-15));
#12062=CARTESIAN_POINT('',(21.25,-10.5,-1.28587913910472E-15));
#12063=CARTESIAN_POINT('Origin',(21.,0.,0.));
#12064=CARTESIAN_POINT('Origin',(15.75,0.,0.));
#12065=CARTESIAN_POINT('',(14.657256909085,15.6307858638156,-1.04370768816965));
#12066=CARTESIAN_POINT('',(15.8,14.2566004799664,-2.33570557485288));
#12067=CARTESIAN_POINT('Ctrl Pts',(14.657256909085,15.6307858638156,-1.04370768816965));
#12068=CARTESIAN_POINT('Ctrl Pts',(14.6761465353607,15.5966120814788,-1.25307480646179));
#12069=CARTESIAN_POINT('Ctrl Pts',(14.7000757634308,15.5497926558527,-1.49278903451664));
#12070=CARTESIAN_POINT('Ctrl Pts',(14.7590833374963,15.4478208788501,-1.84628094543702));
#12071=CARTESIAN_POINT('Ctrl Pts',(14.7853594609294,15.406770809212,-1.94550170191398));
#12072=CARTESIAN_POINT('Ctrl Pts',(14.8353557732901,15.3358943508592,-2.07593726626672));
#12073=CARTESIAN_POINT('Ctrl Pts',(14.8603859823943,15.3033330885441,-2.11619153635774));
#12074=CARTESIAN_POINT('Ctrl Pts',(14.9364214749742,15.2096396742025,-2.20014773094342));
#12075=CARTESIAN_POINT('Ctrl Pts',(14.9903198942812,15.1496310936677,-2.2133567880967));
#12076=CARTESIAN_POINT('Ctrl Pts',(15.1263879851347,14.9906096774748,-2.29478522950976));
#12077=CARTESIAN_POINT('Ctrl Pts',(15.1678275509265,14.9409616025794,-2.32661505826142));
#12078=CARTESIAN_POINT('Ctrl Pts',(15.2552258947252,14.8381944363711,-2.37961344546101));
#12079=CARTESIAN_POINT('Ctrl Pts',(15.3550596759664,14.7212640431372,-2.43498366067061));
#12080=CARTESIAN_POINT('Ctrl Pts',(15.6054597342241,14.4517685598141,-2.42723986374772));
#12081=CARTESIAN_POINT('Ctrl Pts',(15.7019486088057,14.352663795374,-2.39624995256937));
#12082=CARTESIAN_POINT('Ctrl Pts',(15.8,14.2566004799664,-2.33570557485288));
#12083=CARTESIAN_POINT('',(15.8,14.4429346149236,0.328355732126616));
#12084=CARTESIAN_POINT('Ctrl Pts',(15.8,14.4429346149236,0.328355732126617));
#12085=CARTESIAN_POINT('Ctrl Pts',(15.7459792937636,14.500693813047,0.322979723020245));
#12086=CARTESIAN_POINT('Ctrl Pts',(15.6927059160366,14.5578456188153,0.309313059018634));
#12087=CARTESIAN_POINT('Ctrl Pts',(15.5867247540197,14.6717789412866,0.265397252979699));
#12088=CARTESIAN_POINT('Ctrl Pts',(15.5350561720988,14.7274507079623,0.234952142783187));
#12089=CARTESIAN_POINT('Ctrl Pts',(15.415190630386,14.8565358288083,0.143523756746544));
#12090=CARTESIAN_POINT('Ctrl Pts',(15.3214773869099,14.9580982252841,0.0544433185530627));
#12091=CARTESIAN_POINT('Ctrl Pts',(15.0123014953152,15.2843128435265,-0.366133555591651));
#12092=CARTESIAN_POINT('Ctrl Pts',(14.8382414780497,15.4624487588706,-0.667161014661462));
#12093=CARTESIAN_POINT('Ctrl Pts',(14.657256909085,15.6307858638156,-1.04370768816965));
#12094=CARTESIAN_POINT('Origin',(15.8,0.,0.));
#12095=CARTESIAN_POINT('Ctrl Pts',(10.0502525316942,9.05620683581208,-1.38781479615277));
#12096=CARTESIAN_POINT('Ctrl Pts',(11.9668350211294,10.8374137839212,-0.817330781359225));
#12097=CARTESIAN_POINT('Ctrl Pts',(13.8834175105647,12.6186207320302,-0.246846766565678));
#12098=CARTESIAN_POINT('Ctrl Pts',(15.8,14.3998276801393,0.323637248227868));
#12099=CARTESIAN_POINT('Ctrl Pts',(10.0502525316942,9.21244502400637,-1.39655842853149));
#12100=CARTESIAN_POINT('Ctrl Pts',(11.9668350211294,11.0233696506194,-0.813302761662289));
#12101=CARTESIAN_POINT('Ctrl Pts',(13.8834175105647,12.8346197703481,-0.230291956370556));
#12102=CARTESIAN_POINT('Ctrl Pts',(15.8,14.6455443969612,0.352963710498642));
#12103=CARTESIAN_POINT('Ctrl Pts',(10.0502525316942,9.51829373400973,-1.46541714813614));
#12104=CARTESIAN_POINT('Ctrl Pts',(11.9668350211295,11.3925515672309,-0.867231464171977));
#12105=CARTESIAN_POINT('Ctrl Pts',(13.8834175105647,13.2668740653714,-0.269566015193986));
#12106=CARTESIAN_POINT('Ctrl Pts',(15.8,15.1411318985925,0.328619668770177));
#12107=CARTESIAN_POINT('Ctrl Pts',(10.0502525316941,10.0083300006652,-1.79039750449509));
#12108=CARTESIAN_POINT('Ctrl Pts',(11.9668350211294,12.0019243797287,-1.20809631886684));
#12109=CARTESIAN_POINT('Ctrl Pts',(13.8834175105647,13.9956114385883,-0.625444427693875));
#12110=CARTESIAN_POINT('Ctrl Pts',(15.7999999999999,15.9892058176519,-0.0431432420656254));
#12111=CARTESIAN_POINT('Ctrl Pts',(10.0502525316942,10.3276659549724,-2.10732113862254));
#12112=CARTESIAN_POINT('Ctrl Pts',(11.9668350211294,12.4074689224609,-1.55295659524518));
#12113=CARTESIAN_POINT('Ctrl Pts',(13.8834175105647,14.4874157824202,-0.999648742962752));
#12114=CARTESIAN_POINT('Ctrl Pts',(15.8,16.5672187499087,-0.445284199585385));
#12115=CARTESIAN_POINT('Ctrl Pts',(10.0502525316942,10.5073910450885,-2.3220627978979));
#12116=CARTESIAN_POINT('Ctrl Pts',(11.9668350211294,12.6387996550358,-1.79024801807933));
#12117=CARTESIAN_POINT('Ctrl Pts',(13.8834175105647,14.7702082649831,-1.25843323826077));
#12118=CARTESIAN_POINT('Ctrl Pts',(15.8,16.9016168749304,-0.726618458442204));
#12119=CARTESIAN_POINT('',(10.0502525316942,10.5073910450885,-2.3220627978979));
#12120=CARTESIAN_POINT('',(15.8,14.3998276801393,0.323637248227868));
#12121=CARTESIAN_POINT('Ctrl Pts',(15.8,14.3998276801393,0.323637248227868));
#12122=CARTESIAN_POINT('Ctrl Pts',(15.5456570571831,14.1695921802544,0.248663394075437));
#12123=CARTESIAN_POINT('Ctrl Pts',(15.2905259507727,13.9381981568648,0.173284602940039));
#12124=CARTESIAN_POINT('Ctrl Pts',(15.0353275664552,13.7061319160866,0.097716587704992));
#12125=CARTESIAN_POINT('Ctrl Pts',(14.7778789011692,13.4720193682894,0.0214822310000918));
#12126=CARTESIAN_POINT('Ctrl Pts',(14.5203617662627,13.2372226466704,-0.0549444640635663));
#12127=CARTESIAN_POINT('Ctrl Pts',(14.2635162858846,13.0022894235192,-0.131318796804586));
#12128=CARTESIAN_POINT('Ctrl Pts',(14.0000820510511,12.7613295522894,-0.209652329779127));
#12129=CARTESIAN_POINT('Ctrl Pts',(13.7373543721026,12.5202260255194,-0.287930509546324));
#12130=CARTESIAN_POINT('Ctrl Pts',(13.4761318051383,12.2796215208074,-0.365868800886744));
#12131=CARTESIAN_POINT('Ctrl Pts',(13.2939592679836,12.1118276981541,-0.420221747647761));
#12132=CARTESIAN_POINT('Ctrl Pts',(13.1125187344709,11.9442776868953,-0.474408950394494));
#12133=CARTESIAN_POINT('Ctrl Pts',(12.9320810503802,11.7772036867065,-0.528329405335829));
#12134=CARTESIAN_POINT('Ctrl Pts',(12.7419408368636,11.6011457516413,-0.585149281223285));
#12135=CARTESIAN_POINT('Ctrl Pts',(12.5505198646271,11.4234544410918,-0.642388101081205));
#12136=CARTESIAN_POINT('Ctrl Pts',(12.3584606652983,11.2445392798298,-0.699829652727959));
#12137=CARTESIAN_POINT('Ctrl Pts',(12.1609507027362,11.0605463915632,-0.758901432444389));
#12138=CARTESIAN_POINT('Ctrl Pts',(11.9627657724266,10.8752590885173,-0.818187336020626));
#12139=CARTESIAN_POINT('Ctrl Pts',(11.7646046796663,10.6891763370134,-0.877435109077808));
#12140=CARTESIAN_POINT('Ctrl Pts',(11.5611733354013,10.4981445670748,-0.938258623673124));
#12141=CARTESIAN_POINT('Ctrl Pts',(11.3577671135037,10.3062745975188,-0.999041534288636));
#12142=CARTESIAN_POINT('Ctrl Pts',(11.1551420711314,10.1141619588695,-1.05949856916707));
#12143=CARTESIAN_POINT('Ctrl Pts',(10.9369470578885,9.90728713607633,-1.12460120096165));
#12144=CARTESIAN_POINT('Ctrl Pts',(10.7196578904059,9.70013097729891,-1.18932539513645));
#12145=CARTESIAN_POINT('Ctrl Pts',(10.5042186507229,9.49350036754279,-1.25330845309519));
#12146=CARTESIAN_POINT('Ctrl Pts',(10.3518600992381,9.34737127591962,-1.29855724827523));
#12147=CARTESIAN_POINT('Ctrl Pts',(10.2004267545904,9.20150648816192,-1.34343522942928));
#12148=CARTESIAN_POINT('Ctrl Pts',(10.0502525316942,9.05620683581208,-1.38781479615277));
#12149=CARTESIAN_POINT('Ctrl Pts',(15.8,14.3998276801393,0.323637248227868));
#12150=CARTESIAN_POINT('Ctrl Pts',(15.8,14.4084472574799,0.324666000821255));
#12151=CARTESIAN_POINT('Ctrl Pts',(15.8,14.4170677396245,0.325652230376826));
#12152=CARTESIAN_POINT('Ctrl Pts',(15.8,14.4256891265865,0.326595936941114));
#12153=CARTESIAN_POINT('Ctrl Pts',(15.8,14.434311418564,0.327497110819206));
#12154=CARTESIAN_POINT('Ctrl Pts',(15.8,14.4429346149236,0.328355732126616));
#12155=CARTESIAN_POINT('Ctrl Pts',(10.0502525316942,8.18410616705958,-4.11841212213243));
#12156=CARTESIAN_POINT('Ctrl Pts',(11.9668350211294,10.0544238975194,-4.12627279988524));
#12157=CARTESIAN_POINT('Ctrl Pts',(13.8834175105647,11.9247416279792,-4.13413347763806));
#12158=CARTESIAN_POINT('Ctrl Pts',(15.8,13.795059358439,-4.14199415539088));
#12159=CARTESIAN_POINT('Ctrl Pts',(10.0502525316942,8.32999558303832,-4.17500806600468));
#12160=CARTESIAN_POINT('Ctrl Pts',(11.9668350211294,10.2325231628261,-4.17990544851819));
#12161=CARTESIAN_POINT('Ctrl Pts',(13.8834175105647,12.1352846385738,-4.18513629113481));
#12162=CARTESIAN_POINT('Ctrl Pts',(15.8,14.0378122183616,-4.19003367364832));
#12163=CARTESIAN_POINT('Ctrl Pts',(10.0502525316942,8.59959242261693,-4.33502367302148));
#12164=CARTESIAN_POINT('Ctrl Pts',(11.9668350211294,10.5669670902559,-4.34529280263859));
#12165=CARTESIAN_POINT('Ctrl Pts',(13.8834175105647,12.5342444956752,-4.35608887336511));
#12166=CARTESIAN_POINT('Ctrl Pts',(15.8,14.5016191633141,-4.36635800298221));
#12167=CARTESIAN_POINT('Ctrl Pts',(10.0502525316941,8.9652188127798,-4.79552866926094));
#12168=CARTESIAN_POINT('Ctrl Pts',(11.9668350211294,11.0411807000414,-4.85778187524381));
#12169=CARTESIAN_POINT('Ctrl Pts',(13.8834175105647,13.1173407686982,-4.91974349130657));
#12170=CARTESIAN_POINT('Ctrl Pts',(15.7999999999999,15.1933026559598,-4.98199669728944));
#12171=CARTESIAN_POINT('Ctrl Pts',(10.0502525316942,9.17099596015618,-5.19560579312752));
#12172=CARTESIAN_POINT('Ctrl Pts',(11.9668350211294,11.3203141899786,-5.31106824365088));
#12173=CARTESIAN_POINT('Ctrl Pts',(13.8834175105647,13.469442734167,-5.42758013234469));
#12174=CARTESIAN_POINT('Ctrl Pts',(15.8,15.6187609639894,-5.54304258286805));
#12175=CARTESIAN_POINT('Ctrl Pts',(10.0502525316942,9.2755658561365,-5.45537535466284));
#12176=CARTESIAN_POINT('Ctrl Pts',(11.9668350211294,11.4669957083382,-5.60823092528513));
#12177=CARTESIAN_POINT('Ctrl Pts',(13.8834175105647,13.6584255605399,-5.76108649590741));
#12178=CARTESIAN_POINT('Ctrl Pts',(15.8,15.8498554127416,-5.91394206652969));
#12179=CARTESIAN_POINT('',(10.0502525316942,9.2755658561365,-5.45537535466284));
#12180=CARTESIAN_POINT('',(15.8,13.795059358439,-4.14199415539088));
#12181=CARTESIAN_POINT('Ctrl Pts',(15.8,13.795059358439,-4.14199415539088));
#12182=CARTESIAN_POINT('Ctrl Pts',(15.5456574794168,13.5529245928917,-4.14215184549968));
#12183=CARTESIAN_POINT('Ctrl Pts',(15.290526797857,13.3095628770617,-4.14233665870497));
#12184=CARTESIAN_POINT('Ctrl Pts',(15.0353288374168,13.0655033718493,-4.14249371366664));
#12185=CARTESIAN_POINT('Ctrl Pts',(14.7778805061944,12.8192917162879,-4.1426521535606));
#12186=CARTESIAN_POINT('Ctrl Pts',(14.5203637043112,12.5723699372145,-4.14278210218064));
#12187=CARTESIAN_POINT('Ctrl Pts',(14.263518553037,12.3253345162712,-4.14282007025482));
#12188=CARTESIAN_POINT('Ctrl Pts',(14.0000848089524,12.0719621417578,-4.14285901228618));
#12189=CARTESIAN_POINT('Ctrl Pts',(13.7373576158079,11.8184702457672,-4.14280091850188));
#12190=CARTESIAN_POINT('Ctrl Pts',(13.4761355252029,11.5655579735774,-4.14257377376942));
#12191=CARTESIAN_POINT('Ctrl Pts',(13.2939617380614,11.3891793743071,-4.14241536520586));
#12192=CARTESIAN_POINT('Ctrl Pts',(13.1125199626835,11.2130838733106,-4.14217466317553));
#12193=CARTESIAN_POINT('Ctrl Pts',(12.9320810503802,11.0375235228707,-4.14182735974364));
#12194=CARTESIAN_POINT('Ctrl Pts',(12.7419408575526,10.8525241873095,-4.14146138357661));
#12195=CARTESIAN_POINT('Ctrl Pts',(12.5505199062838,10.6658419590985,-4.14098910290385));
#12196=CARTESIAN_POINT('Ctrl Pts',(12.3584607279918,10.4779331330927,-4.14033143664814));
#12197=CARTESIAN_POINT('Ctrl Pts',(12.1609502835644,10.2846908414914,-4.13965510367823));
#12198=CARTESIAN_POINT('Ctrl Pts',(11.9627648680213,10.0901513147852,-4.13878241284077));
#12199=CARTESIAN_POINT('Ctrl Pts',(11.7646032917752,9.89486705365802,-4.13762764472381));
#12200=CARTESIAN_POINT('Ctrl Pts',(11.5611710263525,9.69438863400127,-4.1364421621569));
#12201=CARTESIAN_POINT('Ctrl Pts',(11.3577638852442,9.4931255822132,-4.13495903745938));
#12202=CARTESIAN_POINT('Ctrl Pts',(11.1551379358798,9.29173244419996,-4.13309099161787));
#12203=CARTESIAN_POINT('Ctrl Pts',(10.9369434970433,9.07486553809952,-4.13107941701262));
#12204=CARTESIAN_POINT('Ctrl Pts',(10.7196549052569,8.85784801697106,-4.1286209883191));
#12205=CARTESIAN_POINT('Ctrl Pts',(10.5042162352524,8.64155934492939,-4.1256201089363));
#12206=CARTESIAN_POINT('Ctrl Pts',(10.3518584987032,8.4886004888762,-4.1234978938743));
#12207=CARTESIAN_POINT('Ctrl Pts',(10.2004259609769,8.33600758581753,-4.12110469363328));
#12208=CARTESIAN_POINT('Ctrl Pts',(10.0502525316942,8.18410616705958,-4.11841212213243));
#12209=CARTESIAN_POINT('Ctrl Pts',(15.8,13.795059358439,-4.14199415539088));
#12210=CARTESIAN_POINT('Ctrl Pts',(15.8,13.8035749656708,-4.14367934941586));
#12211=CARTESIAN_POINT('Ctrl Pts',(15.8,13.8120782930811,-4.14540526485286));
#12212=CARTESIAN_POINT('Ctrl Pts',(15.8,13.8205693406969,-4.14717190166177));
#12213=CARTESIAN_POINT('Ctrl Pts',(15.8,13.8290481057107,-4.14897926912419));
#12214=CARTESIAN_POINT('Ctrl Pts',(15.8,13.8375145813754,-4.15082738595568));
#12215=CARTESIAN_POINT('Ctrl Pts',(10.0502525316942,6.51088816465465,-6.44587057493322));
#12216=CARTESIAN_POINT('Ctrl Pts',(11.9668350211294,8.28723694673789,-7.03130648732539));
#12217=CARTESIAN_POINT('Ctrl Pts',(13.8834175105647,10.0635857288211,-7.61674239971757));
#12218=CARTESIAN_POINT('Ctrl Pts',(15.8,11.8399345109044,-8.20217831210975));
#12219=CARTESIAN_POINT('Ctrl Pts',(10.0502525316942,6.63214813591051,-6.54477882498566));
#12220=CARTESIAN_POINT('Ctrl Pts',(11.9668350211294,8.4400460136743,-7.13734986695939));
#12221=CARTESIAN_POINT('Ctrl Pts',(13.8834175105647,10.2480632948761,-7.73031032616364));
#12222=CARTESIAN_POINT('Ctrl Pts',(15.8,12.0559611726399,-8.32288136813736));
#12223=CARTESIAN_POINT('Ctrl Pts',(10.0502525316942,6.83909882511011,-6.78027814405441));
#12224=CARTESIAN_POINT('Ctrl Pts',(11.9668350211295,8.70700998719299,-7.39799687329663));
#12225=CARTESIAN_POINT('Ctrl Pts',(13.8834175105647,10.5746650104356,-8.0161919374395));
#12226=CARTESIAN_POINT('Ctrl Pts',(15.8,12.4425761725185,-8.63391066668172));
#12227=CARTESIAN_POINT('Ctrl Pts',(10.0502525316941,7.04452561799898,-7.33122941665118));
#12228=CARTESIAN_POINT('Ctrl Pts',(11.9668350211294,8.99964539985649,-8.03194323669998));
#12229=CARTESIAN_POINT('Ctrl Pts',(13.8834175105647,10.9550426722923,-8.73244671395171));
#12230=CARTESIAN_POINT('Ctrl Pts',(15.8,12.9101624541498,-9.43316053400051));
#12231=CARTESIAN_POINT('Ctrl Pts',(10.0502525316942,7.11660498267375,-7.77530835268703));
#12232=CARTESIAN_POINT('Ctrl Pts',(11.9668350211294,9.12504823131445,-8.54929552797968));
#12233=CARTESIAN_POINT('Ctrl Pts',(13.8834175105647,11.1329867839676,-9.32422216219827));
#12234=CARTESIAN_POINT('Ctrl Pts',(15.8,13.1414300326083,-10.0982093374909));
#12235=CARTESIAN_POINT('Ctrl Pts',(10.0502525316942,7.13578365451837,-8.05467776187827));
#12236=CARTESIAN_POINT('Ctrl Pts',(11.9668350211294,9.17272232645135,-8.8772411146815));
#12237=CARTESIAN_POINT('Ctrl Pts',(13.8834175105647,11.2096609983843,-9.69980446748474));
#12238=CARTESIAN_POINT('Ctrl Pts',(15.8,13.2465996703173,-10.522367820288));
#12239=CARTESIAN_POINT('',(10.0502525316942,7.13578365451837,-8.05467776187827));
#12240=CARTESIAN_POINT('',(15.8,11.8399345109044,-8.20217831210975));
#12241=CARTESIAN_POINT('Ctrl Pts',(15.8,11.8399345109044,-8.20217831210975));
#12242=CARTESIAN_POINT('Ctrl Pts',(15.5456576615067,11.6096021002861,-8.12750458029291));
#12243=CARTESIAN_POINT('Ctrl Pts',(15.2905271631653,11.3780944093848,-8.05247749955188));
#12244=CARTESIAN_POINT('Ctrl Pts',(15.0353293855237,11.1459316587091,-7.97720839274425));
#12245=CARTESIAN_POINT('Ctrl Pts',(14.7778811978195,10.9117216277039,-7.90127554051952));
#12246=CARTESIAN_POINT('Ctrl Pts',(14.5203645390055,10.6768450327867,-7.82509615349673));
#12247=CARTESIAN_POINT('Ctrl Pts',(14.2635195291145,10.4418887807062,-7.748794170348));
#12248=CARTESIAN_POINT('Ctrl Pts',(14.0000859949211,10.2009054892938,-7.67053490770798));
#12249=CARTESIAN_POINT('Ctrl Pts',(13.7373590095462,9.95983851106089,-7.59214642417434));
#12250=CARTESIAN_POINT('Ctrl Pts',(13.4761371226647,9.71937502567175,-7.51377627479589));
#12251=CARTESIAN_POINT('Ctrl Pts',(13.2939627987566,9.5516774663351,-7.45912147864526));
#12252=CARTESIAN_POINT('Ctrl Pts',(13.1125204900998,9.38427458086322,-7.404475897828));
#12253=CARTESIAN_POINT('Ctrl Pts',(12.9320810503802,9.21741359915303,-7.34989430276011));
#12254=CARTESIAN_POINT('Ctrl Pts',(12.7419408661181,9.0415818749035,-7.29237830426415));
#12255=CARTESIAN_POINT('Ctrl Pts',(12.5505199235302,8.8641824751674,-7.23424116054649));
#12256=CARTESIAN_POINT('Ctrl Pts',(12.3584607539476,8.68567379986616,-7.17554866346896));
#12257=CARTESIAN_POINT('Ctrl Pts',(12.1609501017811,8.5020982645104,-7.11519021559973));
#12258=CARTESIAN_POINT('Ctrl Pts',(11.9627644770481,8.31734966162794,-7.0542441495787));
#12259=CARTESIAN_POINT('Ctrl Pts',(11.7646026923668,8.13197994128604,-6.99279967398786));
#12260=CARTESIAN_POINT('Ctrl Pts',(11.5611700299521,7.9416795975498,-6.92972084534173));
#12261=CARTESIAN_POINT('Ctrl Pts',(11.3577624926924,7.75072500004993,-6.86611647390364));
#12262=CARTESIAN_POINT('Ctrl Pts',(11.1551361524442,7.55976563308339,-6.80210582000275));
#12263=CARTESIAN_POINT('Ctrl Pts',(10.9369419552394,7.35413478704945,-6.73317720379544));
#12264=CARTESIAN_POINT('Ctrl Pts',(10.7196536056915,7.1484987864115,-6.66377706212351));
#12265=CARTESIAN_POINT('Ctrl Pts',(10.5042151754601,6.94372358733477,-6.5940862490785));
#12266=CARTESIAN_POINT('Ctrl Pts',(10.3518577964654,6.79890721181192,-6.54480112569479));
#12267=CARTESIAN_POINT('Ctrl Pts',(10.2004256127774,6.65452261540791,-6.49537136769534));
#12268=CARTESIAN_POINT('Ctrl Pts',(10.0502525316942,6.51088816465465,-6.44587057493322));
#12269=CARTESIAN_POINT('Ctrl Pts',(15.8,11.8399345109044,-8.20217831210975));
#12270=CARTESIAN_POINT('Ctrl Pts',(15.8,11.8475125810599,-8.20641249422049));
#12271=CARTESIAN_POINT('Ctrl Pts',(15.8,11.8550663888027,-8.21068161002192));
#12272=CARTESIAN_POINT('Ctrl Pts',(15.8,11.862595934171,-8.21498565948429));
#12273=CARTESIAN_POINT('Ctrl Pts',(15.8,11.8701012116266,-8.21932465056733));
#12274=CARTESIAN_POINT('Ctrl Pts',(15.8,11.8775822089691,-8.22369859898568));
#12275=CARTESIAN_POINT('Ctrl Pts',(10.0502525316942,4.20033906466803,-8.14236230483842));
#12276=CARTESIAN_POINT('Ctrl Pts',(11.9668350211294,5.70883750303466,-9.24806690579316));
#12277=CARTESIAN_POINT('Ctrl Pts',(13.8834175105647,7.21733594140129,-10.3537715067479));
#12278=CARTESIAN_POINT('Ctrl Pts',(15.8,8.72583437976793,-11.4594761077026));
#12279=CARTESIAN_POINT('Ctrl Pts',(10.0502525316942,4.28509982034658,-8.27390103242161));
#12280=CARTESIAN_POINT('Ctrl Pts',(11.9668350211294,5.82139835544565,-9.39614075158194));
#12281=CARTESIAN_POINT('Ctrl Pts',(13.8834175105647,7.35769011342039,-10.5187877262285));
#12282=CARTESIAN_POINT('Ctrl Pts',(15.8,8.89398864851946,-11.6410274453888));
#12283=CARTESIAN_POINT('Ctrl Pts',(10.0502525316942,4.40914912230233,-8.56182484570056));
#12284=CARTESIAN_POINT('Ctrl Pts',(11.9668350211295,5.99475261978217,-9.7265265614502));
#12285=CARTESIAN_POINT('Ctrl Pts',(13.8834175105647,7.57996568930601,-10.8916014121612));
#12286=CARTESIAN_POINT('Ctrl Pts',(15.8,9.16556918678585,-12.0563031279108));
#12287=CARTESIAN_POINT('Ctrl Pts',(10.0502525316941,4.43426842278353,-9.14929101108337));
#12288=CARTESIAN_POINT('Ctrl Pts',(11.9668350211294,6.0771653528682,-10.4198746943315));
#12289=CARTESIAN_POINT('Ctrl Pts',(13.8834175105647,7.7203916302128,-11.6903432820695));
#12290=CARTESIAN_POINT('Ctrl Pts',(15.7999999999999,9.36328856029747,-12.9609269653176));
#12291=CARTESIAN_POINT('Ctrl Pts',(10.0502525316942,4.36559112518463,-9.59390955692677));
#12292=CARTESIAN_POINT('Ctrl Pts',(11.9668350211294,6.03655897381968,-10.9506581995853));
#12293=CARTESIAN_POINT('Ctrl Pts',(13.8834175105647,7.70675651927341,-12.30814436114));
#12294=CARTESIAN_POINT('Ctrl Pts',(15.8,9.37772436790846,-13.6648930037986));
#12295=CARTESIAN_POINT('Ctrl Pts',(10.0502525316942,4.29750123086779,-9.86553218952114));
#12296=CARTESIAN_POINT('Ctrl Pts',(11.9668350211294,5.98055897313701,-11.2772850923971));
#12297=CARTESIAN_POINT('Ctrl Pts',(13.8834175105647,7.66361671540623,-12.689037995273));
#12298=CARTESIAN_POINT('Ctrl Pts',(15.8,9.34667445767544,-14.1007908981489));
#12299=CARTESIAN_POINT('',(10.0502525316942,4.29750123086779,-9.86553218952114));
#12300=CARTESIAN_POINT('',(15.8,8.72583437976793,-11.4594761077026));
#12301=CARTESIAN_POINT('Ctrl Pts',(15.8,8.72583437976793,-11.4594761077026));
#12302=CARTESIAN_POINT('Ctrl Pts',(15.5456576332001,8.52985067008859,-11.3172805234003));
#12303=CARTESIAN_POINT('Ctrl Pts',(15.2905271063766,8.3328583934094,-11.1743857021214));
#12304=CARTESIAN_POINT('Ctrl Pts',(15.0353293003182,8.13531790820428,-11.0310582754415));
#12305=CARTESIAN_POINT('Ctrl Pts',(14.7778810903251,7.93603545706285,-10.8864669483781));
#12306=CARTESIAN_POINT('Ctrl Pts',(14.5203644092919,7.73619524960907,-10.7414351729092));
#12307=CARTESIAN_POINT('Ctrl Pts',(14.2635193774437,7.536317168099,-10.5962621862442));
#12308=CARTESIAN_POINT('Ctrl Pts',(14.0000858106901,7.33131185594966,-10.4473652525631));
#12309=CARTESIAN_POINT('Ctrl Pts',(13.7373587930845,7.12626688447453,-10.2983195619273));
#12310=CARTESIAN_POINT('Ctrl Pts',(13.4761368746002,6.92179020337864,-10.1494777980995));
#12311=CARTESIAN_POINT('Ctrl Pts',(13.2939626340448,6.77918967312429,-10.045676649078));
#12312=CARTESIAN_POINT('Ctrl Pts',(13.1125204081991,6.6368665464255,-9.94197532369119));
#12313=CARTESIAN_POINT('Ctrl Pts',(12.9320810503802,6.49503902755748,-9.83850230979698));
#12314=CARTESIAN_POINT('Ctrl Pts',(12.7419408648007,6.34558654067317,-9.72946635277447));
#12315=CARTESIAN_POINT('Ctrl Pts',(12.5505199208776,6.1948350500801,-9.61935521332116));
#12316=CARTESIAN_POINT('Ctrl Pts',(12.3584607499554,6.04320018913792,-9.5083731166294));
#12317=CARTESIAN_POINT('Ctrl Pts',(12.1609501300797,5.88726129158026,-9.39424088015544));
#12318=CARTESIAN_POINT('Ctrl Pts',(11.9627645378629,5.73038832458546,-9.27918728832953));
#12319=CARTESIAN_POINT('Ctrl Pts',(11.7646027855806,5.57307865663086,-9.16346774534082));
#12320=CARTESIAN_POINT('Ctrl Pts',(11.5611701848689,5.41158475328924,-9.04467021094167));
#12321=CARTESIAN_POINT('Ctrl Pts',(11.3577627091815,5.24963101923089,-8.9251706806875));
#12322=CARTESIAN_POINT('Ctrl Pts',(11.1551364296869,5.08779829683645,-8.80528327914596));
#12323=CARTESIAN_POINT('Ctrl Pts',(10.9369421951535,4.91353182422793,-8.6761848232359));
#12324=CARTESIAN_POINT('Ctrl Pts',(10.7196538081806,4.73940615822496,-8.54663632684921));
#12325=CARTESIAN_POINT('Ctrl Pts',(10.5042153409026,4.5661889859333,-8.41707738748313));
#12326=CARTESIAN_POINT('Ctrl Pts',(10.3518579060906,4.44369032369729,-8.32545369600329));
#12327=CARTESIAN_POINT('Ctrl Pts',(10.2004256671343,4.32164700273164,-8.23382587572336));
#12328=CARTESIAN_POINT('Ctrl Pts',(10.0502525316942,4.20033906466803,-8.14236230483842));
#12329=CARTESIAN_POINT('Ctrl Pts',(15.8,8.72583437976793,-11.4594761077026));
#12330=CARTESIAN_POINT('Ctrl Pts',(15.8,8.73173311854078,-11.4658448066529));
#12331=CARTESIAN_POINT('Ctrl Pts',(15.8,8.73759798728384,-11.4722392320194));
#12332=CARTESIAN_POINT('Ctrl Pts',(15.8,8.74342898604263,-11.4786593837858));
#12333=CARTESIAN_POINT('Ctrl Pts',(15.8,8.7492261070902,-11.4851052678107));
#12334=CARTESIAN_POINT('Ctrl Pts',(15.8,8.7549893339674,-11.4915768952696));
#12335=CARTESIAN_POINT('Ctrl Pts',(10.0502525316942,1.47863151154858,-9.041822881172));
#12336=CARTESIAN_POINT('Ctrl Pts',(11.9668350211294,2.57161726872464,-10.5595621004509));
#12337=CARTESIAN_POINT('Ctrl Pts',(13.8834175105647,3.66460302590071,-12.0773013197298));
#12338=CARTESIAN_POINT('Ctrl Pts',(15.8,4.75758878307678,-13.5950405390087));
#12339=CARTESIAN_POINT('Ctrl Pts',(10.0502525316942,1.5185960783211,-9.19311615914592));
#12340=CARTESIAN_POINT('Ctrl Pts',(11.9668350211294,2.63291166611866,-10.7351719126775));
#12341=CARTESIAN_POINT('Ctrl Pts',(13.8834175105647,3.74709495962167,-12.2776128949465));
#12342=CARTESIAN_POINT('Ctrl Pts',(15.8,4.86141054741923,-13.8196686484781));
#12343=CARTESIAN_POINT('Ctrl Pts',(10.0502525316942,1.54760878347554,-9.50527827631687));
#12344=CARTESIAN_POINT('Ctrl Pts',(11.9668350211294,2.69569469846983,-11.1029538596823));
#12345=CARTESIAN_POINT('Ctrl Pts',(13.8834175105647,3.84329897549065,-12.7008586295609));
#12346=CARTESIAN_POINT('Ctrl Pts',(15.8,4.99138489048493,-14.2985342129264));
#12347=CARTESIAN_POINT('Ctrl Pts',(10.0502525316941,1.3899625395975,-10.0717544060046));
#12348=CARTESIAN_POINT('Ctrl Pts',(11.9668350211294,2.55981841965666,-11.7878343688586));
#12349=CARTESIAN_POINT('Ctrl Pts',(13.8834175105647,3.73002877331941,-13.5039013178588));
#12350=CARTESIAN_POINT('Ctrl Pts',(15.7999999999999,4.89988465337857,-15.2199812807128));
#12351=CARTESIAN_POINT('Ctrl Pts',(10.0502525316942,1.18724279150055,-10.473392049036));
#12352=CARTESIAN_POINT('Ctrl Pts',(11.9668350211294,2.35716926478797,-12.2800941488934));
#12353=CARTESIAN_POINT('Ctrl Pts',(13.8834175105647,3.52613523034269,-14.0872596341291));
#12354=CARTESIAN_POINT('Ctrl Pts',(15.8,4.6960617036301,-15.8939617339865));
#12355=CARTESIAN_POINT('Ctrl Pts',(10.0502525316942,1.03854944428814,-10.7106795892491));
#12356=CARTESIAN_POINT('Ctrl Pts',(11.9668350211294,2.20297683852746,-12.5734298318033));
#12357=CARTESIAN_POINT('Ctrl Pts',(13.8834175105647,3.36740423276678,-14.4361800743576));
#12358=CARTESIAN_POINT('Ctrl Pts',(15.8,4.5318316270061,-16.2989303169119));
#12359=CARTESIAN_POINT('',(10.0502525316942,1.03854944428814,-10.7106795892491));
#12360=CARTESIAN_POINT('',(15.8,4.75758878307678,-13.5950405390087));
#12361=CARTESIAN_POINT('Ctrl Pts',(15.8,4.75758878307678,-13.5950405390087));
#12362=CARTESIAN_POINT('Ctrl Pts',(15.5456573899561,4.61513791473822,-13.3992420178035));
#12363=CARTESIAN_POINT('Ctrl Pts',(15.2905266183811,4.47194392111085,-13.2024668138655));
#12364=CARTESIAN_POINT('Ctrl Pts',(15.0353285681319,4.32836223491289,-13.0051107697458));
#12365=CARTESIAN_POINT('Ctrl Pts',(14.7778801662808,4.18351443685701,-12.8060144282783));
#12366=CARTESIAN_POINT('Ctrl Pts',(14.5203632939894,4.03827228948957,-12.6063268373508));
#12367=CARTESIAN_POINT('Ctrl Pts',(14.2635180731361,3.89303775923336,-12.4064932437269));
#12368=CARTESIAN_POINT('Ctrl Pts',(14.0000842255548,3.74407765407761,-12.2015334929889));
#12369=CARTESIAN_POINT('Ctrl Pts',(13.7373569299582,3.59512579987268,-11.9964200114428));
#12370=CARTESIAN_POINT('Ctrl Pts',(13.4761347388948,3.44665140507618,-11.7916760912323));
#12371=CARTESIAN_POINT('Ctrl Pts',(13.2939612159623,3.34310697244114,-11.6488899018511));
#12372=CARTESIAN_POINT('Ctrl Pts',(13.1125197030769,3.23979551676097,-11.5062843729551));
#12373=CARTESIAN_POINT('Ctrl Pts',(12.9320810503802,3.13688485529761,-11.3640491305165));
#12374=CARTESIAN_POINT('Ctrl Pts',(12.7419408532675,3.02844105368857,-11.2141664051166));
#12375=CARTESIAN_POINT('Ctrl Pts',(12.5505198976557,2.91909407414949,-11.0628597070359));
#12376=CARTESIAN_POINT('Ctrl Pts',(12.3584607150065,2.8091760977475,-10.9104517039517));
#12377=CARTESIAN_POINT('Ctrl Pts',(12.1609503726549,2.69613835151592,-10.7537179490172));
#12378=CARTESIAN_POINT('Ctrl Pts',(11.9627650599008,2.58249696621073,-10.5958192942301));
#12379=CARTESIAN_POINT('Ctrl Pts',(11.7646035860731,2.46864604141747,-10.4371523366742));
#12380=CARTESIAN_POINT('Ctrl Pts',(11.5611715157473,2.3517669685492,-10.2742652373587));
#12381=CARTESIAN_POINT('Ctrl Pts',(11.3577645693232,2.23466749726821,-10.110568409322));
#12382=CARTESIAN_POINT('Ctrl Pts',(11.1551388120548,2.11780296935792,-9.94654008829837));
#12383=CARTESIAN_POINT('Ctrl Pts',(10.936944253188,1.99195912572073,-9.76990860950771));
#12384=CARTESIAN_POINT('Ctrl Pts',(10.7196555410841,1.86638826421828,-9.59289262515089));
#12385=CARTESIAN_POINT('Ctrl Pts',(10.5042167520016,1.7416846628415,-9.41614744679623));
#12386=CARTESIAN_POINT('Ctrl Pts',(10.3518588411106,1.65349450791511,-9.29115358543616));
#12387=CARTESIAN_POINT('Ctrl Pts',(10.2004261307571,1.56573868767392,-9.16629650496067));
#12388=CARTESIAN_POINT('Ctrl Pts',(10.0502525316942,1.47863151154858,-9.041822881172));
#12389=CARTESIAN_POINT('Ctrl Pts',(15.8,4.75758878307678,-13.5950405390087));
#12390=CARTESIAN_POINT('Ctrl Pts',(15.8,4.76123078081695,-13.6029203421718));
#12391=CARTESIAN_POINT('Ctrl Pts',(15.8,4.76483261634472,-13.610814146196));
#12392=CARTESIAN_POINT('Ctrl Pts',(15.8,4.7683942897085,-13.6187219510797));
#12393=CARTESIAN_POINT('Ctrl Pts',(15.8,4.77191579174907,-13.626643760007));
#12394=CARTESIAN_POINT('Ctrl Pts',(15.8,4.77539710335945,-13.6345795785203));
#12395=CARTESIAN_POINT('Ctrl Pts',(10.0502525316942,-1.38781479615277,-9.05620683581208));
#12396=CARTESIAN_POINT('Ctrl Pts',(11.9668350211294,-0.817330781359224,
-10.8374137839212));
#12397=CARTESIAN_POINT('Ctrl Pts',(13.8834175105647,-0.246846766565677,
-12.6186207320302));
#12398=CARTESIAN_POINT('Ctrl Pts',(15.8,0.32363724822787,-14.3998276801393));
#12399=CARTESIAN_POINT('Ctrl Pts',(10.0502525316942,-1.39655842853148,-9.21244502400637));
#12400=CARTESIAN_POINT('Ctrl Pts',(11.9668350211294,-0.813302761662288,
-11.0233696506194));
#12401=CARTESIAN_POINT('Ctrl Pts',(13.8834175105647,-0.230291956370554,
-12.8346197703481));
#12402=CARTESIAN_POINT('Ctrl Pts',(15.8,0.352963710498643,-14.6455443969611));
#12403=CARTESIAN_POINT('Ctrl Pts',(10.0502525316942,-1.46541714813614,-9.51829373400973));
#12404=CARTESIAN_POINT('Ctrl Pts',(11.9668350211295,-0.867231464171971,
-11.3925515672309));
#12405=CARTESIAN_POINT('Ctrl Pts',(13.8834175105647,-0.269566015193986,
-13.2668740653714));
#12406=CARTESIAN_POINT('Ctrl Pts',(15.8,0.328619668770179,-15.1411318985925));
#12407=CARTESIAN_POINT('Ctrl Pts',(10.0502525316941,-1.7903975044951,-10.0083300006652));
#12408=CARTESIAN_POINT('Ctrl Pts',(11.9668350211294,-1.20809631886685,-12.0019243797287));
#12409=CARTESIAN_POINT('Ctrl Pts',(13.8834175105647,-0.625444427693872,
-13.9956114385883));
#12410=CARTESIAN_POINT('Ctrl Pts',(15.8,-0.0431432420656229,-15.9892058176518));
#12411=CARTESIAN_POINT('Ctrl Pts',(10.0502525316942,-2.10732113862255,-10.3276659549724));
#12412=CARTESIAN_POINT('Ctrl Pts',(11.9668350211294,-1.55295659524519,-12.4074689224609));
#12413=CARTESIAN_POINT('Ctrl Pts',(13.8834175105647,-0.999648742962751,
-14.4874157824203));
#12414=CARTESIAN_POINT('Ctrl Pts',(15.8,-0.445284199585383,-16.5672187499088));
#12415=CARTESIAN_POINT('Ctrl Pts',(10.0502525316942,-2.32206279789789,-10.5073910450885));
#12416=CARTESIAN_POINT('Ctrl Pts',(11.9668350211294,-1.79024801807933,-12.6387996550358));
#12417=CARTESIAN_POINT('Ctrl Pts',(13.8834175105647,-1.25843323826077,-14.7702082649831));
#12418=CARTESIAN_POINT('Ctrl Pts',(15.8,-0.726618458442201,-16.9016168749304));
#12419=CARTESIAN_POINT('',(10.0502525316942,-2.32206279789789,-10.5073910450885));
#12420=CARTESIAN_POINT('',(15.8,0.32363724822787,-14.3998276801393));
#12421=CARTESIAN_POINT('Ctrl Pts',(15.8,0.32363724822787,-14.3998276801393));
#12422=CARTESIAN_POINT('Ctrl Pts',(15.5456570571815,0.248663394074979,-14.169592180253));
#12423=CARTESIAN_POINT('Ctrl Pts',(15.2905259507696,0.173284602939125,-13.938198156862));
#12424=CARTESIAN_POINT('Ctrl Pts',(15.0353275664506,0.0977165877036246,
-13.7061319160824));
#12425=CARTESIAN_POINT('Ctrl Pts',(14.7778789011639,0.0214822309985085,
-13.4720193682845));
#12426=CARTESIAN_POINT('Ctrl Pts',(14.5203617662566,-0.0549444640653608,
-13.2372226466649));
#12427=CARTESIAN_POINT('Ctrl Pts',(14.2635162858779,-0.131318796806587,
-13.002289423513));
#12428=CARTESIAN_POINT('Ctrl Pts',(14.0000820510449,-0.209652329780965,
-12.7613295522838));
#12429=CARTESIAN_POINT('Ctrl Pts',(13.7373543720969,-0.287930509547997,
-12.5202260255142));
#12430=CARTESIAN_POINT('Ctrl Pts',(13.4761318051332,-0.365868800888249,
-12.2796215208027));
#12431=CARTESIAN_POINT('Ctrl Pts',(13.2939592679802,-0.420221747648761,
-12.111827698151));
#12432=CARTESIAN_POINT('Ctrl Pts',(13.1125187344693,-0.47440895039499,-11.9442776868938));
#12433=CARTESIAN_POINT('Ctrl Pts',(12.9320810503802,-0.528329405335827,
-11.7772036867065));
#12434=CARTESIAN_POINT('Ctrl Pts',(12.7419408368629,-0.585149281223488,
-11.6011457516407));
#12435=CARTESIAN_POINT('Ctrl Pts',(12.5505198646257,-0.642388101081619,
-11.4234544410905));
#12436=CARTESIAN_POINT('Ctrl Pts',(12.3584606652962,-0.699829652728586,
-11.2445392798278));
#12437=CARTESIAN_POINT('Ctrl Pts',(12.1609507027341,-0.758901432445018,
-11.0605463915612));
#12438=CARTESIAN_POINT('Ctrl Pts',(11.9627657724245,-0.818187336021259,
-10.8752590885153));
#12439=CARTESIAN_POINT('Ctrl Pts',(11.7646046796641,-0.877435109078444,
-10.6891763370114));
#12440=CARTESIAN_POINT('Ctrl Pts',(11.5611733353989,-0.938258623673827,
-10.4981445670725));
#12441=CARTESIAN_POINT('Ctrl Pts',(11.3577671135011,-0.999041534289407,
-10.3062745975164));
#12442=CARTESIAN_POINT('Ctrl Pts',(11.1551420711286,-1.05949856916791,-10.1141619588668));
#12443=CARTESIAN_POINT('Ctrl Pts',(10.9369470578857,-1.12460120096249,-9.90728713607363));
#12444=CARTESIAN_POINT('Ctrl Pts',(10.719657890403,-1.1893253951373,-9.70013097729617));
#12445=CARTESIAN_POINT('Ctrl Pts',(10.50421865072,-1.25330845309604,-9.49350036754002));
#12446=CARTESIAN_POINT('Ctrl Pts',(10.3518600992362,-1.2985572482758,-9.34737127591778));
#12447=CARTESIAN_POINT('Ctrl Pts',(10.2004267545894,-1.34343522942956,-9.201506488161));
#12448=CARTESIAN_POINT('Ctrl Pts',(10.0502525316942,-1.38781479615277,-9.05620683581208));
#12449=CARTESIAN_POINT('Ctrl Pts',(15.8,0.32363724822787,-14.3998276801393));
#12450=CARTESIAN_POINT('Ctrl Pts',(15.8,0.324666000821257,-14.4084472574799));
#12451=CARTESIAN_POINT('Ctrl Pts',(15.8,0.325652230376828,-14.4170677396245));
#12452=CARTESIAN_POINT('Ctrl Pts',(15.8,0.326595936941116,-14.4256891265865));
#12453=CARTESIAN_POINT('Ctrl Pts',(15.8,0.327497110819208,-14.434311418564));
#12454=CARTESIAN_POINT('Ctrl Pts',(15.8,0.328355732126618,-14.4429346149236));
#12455=CARTESIAN_POINT('Ctrl Pts',(10.0502525316942,-4.11841212213242,-8.18410616705958));
#12456=CARTESIAN_POINT('Ctrl Pts',(11.9668350211294,-4.12627279988524,-10.0544238975194));
#12457=CARTESIAN_POINT('Ctrl Pts',(13.8834175105647,-4.13413347763806,-11.9247416279792));
#12458=CARTESIAN_POINT('Ctrl Pts',(15.8,-4.14199415539088,-13.795059358439));
#12459=CARTESIAN_POINT('Ctrl Pts',(10.0502525316942,-4.17500806600467,-8.32999558303832));
#12460=CARTESIAN_POINT('Ctrl Pts',(11.9668350211294,-4.17990544851818,-10.2325231628261));
#12461=CARTESIAN_POINT('Ctrl Pts',(13.8834175105647,-4.18513629113482,-12.1352846385738));
#12462=CARTESIAN_POINT('Ctrl Pts',(15.8,-4.19003367364834,-14.0378122183616));
#12463=CARTESIAN_POINT('Ctrl Pts',(10.0502525316942,-4.33502367302149,-8.59959242261694));
#12464=CARTESIAN_POINT('Ctrl Pts',(11.9668350211295,-4.34529280263859,-10.5669670902559));
#12465=CARTESIAN_POINT('Ctrl Pts',(13.8834175105647,-4.3560888733651,-12.5342444956751));
#12466=CARTESIAN_POINT('Ctrl Pts',(15.8,-4.36635800298221,-14.5016191633141));
#12467=CARTESIAN_POINT('Ctrl Pts',(10.0502525316941,-4.79552866926091,-8.9652188127798));
#12468=CARTESIAN_POINT('Ctrl Pts',(11.9668350211294,-4.85778187524378,-11.0411807000414));
#12469=CARTESIAN_POINT('Ctrl Pts',(13.8834175105647,-4.91974349130655,-13.1173407686982));
#12470=CARTESIAN_POINT('Ctrl Pts',(15.8,-4.98199669728942,-15.1933026559598));
#12471=CARTESIAN_POINT('Ctrl Pts',(10.0502525316942,-5.19560579312754,-9.17099596015618));
#12472=CARTESIAN_POINT('Ctrl Pts',(11.9668350211294,-5.3110682436509,-11.3203141899786));
#12473=CARTESIAN_POINT('Ctrl Pts',(13.8834175105647,-5.42758013234469,-13.4694427341669));
#12474=CARTESIAN_POINT('Ctrl Pts',(15.8,-5.54304258286804,-15.6187609639894));
#12475=CARTESIAN_POINT('Ctrl Pts',(10.0502525316942,-5.45537535466284,-9.2755658561365));
#12476=CARTESIAN_POINT('Ctrl Pts',(11.9668350211294,-5.60823092528512,-11.4669957083382));
#12477=CARTESIAN_POINT('Ctrl Pts',(13.8834175105647,-5.76108649590741,-13.6584255605399));
#12478=CARTESIAN_POINT('Ctrl Pts',(15.8,-5.91394206652969,-15.8498554127416));
#12479=CARTESIAN_POINT('',(10.0502525316942,-5.45537535466284,-9.2755658561365));
#12480=CARTESIAN_POINT('',(15.8,-4.14199415539088,-13.795059358439));
#12481=CARTESIAN_POINT('Ctrl Pts',(15.8,-4.14199415539088,-13.795059358439));
#12482=CARTESIAN_POINT('Ctrl Pts',(15.5456574794166,-4.14215184549968,-13.5529245928915));
#12483=CARTESIAN_POINT('Ctrl Pts',(15.2905267978566,-4.14233665870497,-13.3095628770613));
#12484=CARTESIAN_POINT('Ctrl Pts',(15.0353288374161,-4.14249371366664,-13.0655033718487));
#12485=CARTESIAN_POINT('Ctrl Pts',(14.7778805061951,-4.1426521535606,-12.8192917162886));
#12486=CARTESIAN_POINT('Ctrl Pts',(14.5203637043132,-4.14278210218064,-12.5723699372164));
#12487=CARTESIAN_POINT('Ctrl Pts',(14.2635185530402,-4.14282007025482,-12.3253345162743));
#12488=CARTESIAN_POINT('Ctrl Pts',(14.0000848089565,-4.14285901228618,-12.0719621417617));
#12489=CARTESIAN_POINT('Ctrl Pts',(13.7373576158128,-4.14280091850188,-11.818470245772));
#12490=CARTESIAN_POINT('Ctrl Pts',(13.4761355252086,-4.14257377376942,-11.565557973583));
#12491=CARTESIAN_POINT('Ctrl Pts',(13.2939617380651,-4.14241536520587,-11.3891793743108));
#12492=CARTESIAN_POINT('Ctrl Pts',(13.1125199626854,-4.14217466317553,-11.2130838733124));
#12493=CARTESIAN_POINT('Ctrl Pts',(12.9320810503802,-4.14182735974364,-11.0375235228707));
#12494=CARTESIAN_POINT('Ctrl Pts',(12.7419408575527,-4.14146138357661,-10.8525241873096));
#12495=CARTESIAN_POINT('Ctrl Pts',(12.5505199062839,-4.14098910290385,-10.6658419590986));
#12496=CARTESIAN_POINT('Ctrl Pts',(12.3584607279919,-4.14033143664814,-10.4779331330928));
#12497=CARTESIAN_POINT('Ctrl Pts',(12.1609502835647,-4.13965510367823,-10.2846908414917));
#12498=CARTESIAN_POINT('Ctrl Pts',(11.9627648680217,-4.13878241284077,-10.0901513147856));
#12499=CARTESIAN_POINT('Ctrl Pts',(11.7646032917758,-4.13762764472381,-9.89486705365855));
#12500=CARTESIAN_POINT('Ctrl Pts',(11.5611710263533,-4.13644216215691,-9.69438863400203));
#12501=CARTESIAN_POINT('Ctrl Pts',(11.3577638852452,-4.13495903745938,-9.49312558221419));
#12502=CARTESIAN_POINT('Ctrl Pts',(11.155137935881,-4.13309099161788,-9.29173244420118));
#12503=CARTESIAN_POINT('Ctrl Pts',(10.9369434970446,-4.13107941701263,-9.07486553810084));
#12504=CARTESIAN_POINT('Ctrl Pts',(10.7196549052583,-4.12862098831911,-8.85784801697248));
#12505=CARTESIAN_POINT('Ctrl Pts',(10.5042162352539,-4.12562010893632,-8.64155934493092));
#12506=CARTESIAN_POINT('Ctrl Pts',(10.3518584987042,-4.12349789387431,-8.48860048887722));
#12507=CARTESIAN_POINT('Ctrl Pts',(10.2004259609774,-4.12110469363328,-8.33600758581804));
#12508=CARTESIAN_POINT('Ctrl Pts',(10.0502525316942,-4.11841212213242,-8.18410616705958));
#12509=CARTESIAN_POINT('Ctrl Pts',(15.8,-4.14199415539088,-13.795059358439));
#12510=CARTESIAN_POINT('Ctrl Pts',(15.8,-4.14367934941586,-13.8035749656708));
#12511=CARTESIAN_POINT('Ctrl Pts',(15.8,-4.14540526485286,-13.8120782930811));
#12512=CARTESIAN_POINT('Ctrl Pts',(15.8,-4.14717190166177,-13.8205693406969));
#12513=CARTESIAN_POINT('Ctrl Pts',(15.8,-4.14897926912419,-13.8290481057107));
#12514=CARTESIAN_POINT('Ctrl Pts',(15.8,-4.15082738595568,-13.8375145813754));
#12515=CARTESIAN_POINT('Ctrl Pts',(10.0502525316942,-6.44587057493322,-6.51088816465466));
#12516=CARTESIAN_POINT('Ctrl Pts',(11.9668350211294,-7.03130648732539,-8.28723694673789));
#12517=CARTESIAN_POINT('Ctrl Pts',(13.8834175105647,-7.61674239971757,-10.0635857288211));
#12518=CARTESIAN_POINT('Ctrl Pts',(15.8,-8.20217831210975,-11.8399345109044));
#12519=CARTESIAN_POINT('Ctrl Pts',(10.0502525316942,-6.54477882498566,-6.63214813591052));
#12520=CARTESIAN_POINT('Ctrl Pts',(11.9668350211294,-7.13734986695939,-8.4400460136743));
#12521=CARTESIAN_POINT('Ctrl Pts',(13.8834175105647,-7.73031032616364,-10.2480632948761));
#12522=CARTESIAN_POINT('Ctrl Pts',(15.8,-8.32288136813736,-12.0559611726399));
#12523=CARTESIAN_POINT('Ctrl Pts',(10.0502525316942,-6.78027814405441,-6.83909882511009));
#12524=CARTESIAN_POINT('Ctrl Pts',(11.9668350211295,-7.39799687329663,-8.70700998719297));
#12525=CARTESIAN_POINT('Ctrl Pts',(13.8834175105647,-8.01619193743949,-10.5746650104356));
#12526=CARTESIAN_POINT('Ctrl Pts',(15.8,-8.6339106666817,-12.4425761725185));
#12527=CARTESIAN_POINT('Ctrl Pts',(10.0502525316941,-7.33122941665115,-7.04452561799895));
#12528=CARTESIAN_POINT('Ctrl Pts',(11.9668350211294,-8.03194323669995,-8.99964539985646));
#12529=CARTESIAN_POINT('Ctrl Pts',(13.8834175105647,-8.73244671395173,-10.9550426722922));
#12530=CARTESIAN_POINT('Ctrl Pts',(15.8,-9.43316053400054,-12.9101624541497));
#12531=CARTESIAN_POINT('Ctrl Pts',(10.0502525316942,-7.77530835268703,-7.11660498267375));
#12532=CARTESIAN_POINT('Ctrl Pts',(11.9668350211294,-8.54929552797968,-9.12504823131445));
#12533=CARTESIAN_POINT('Ctrl Pts',(13.8834175105647,-9.32422216219831,-11.1329867839675));
#12534=CARTESIAN_POINT('Ctrl Pts',(15.8,-10.098209337491,-13.1414300326082));
#12535=CARTESIAN_POINT('Ctrl Pts',(10.0502525316942,-8.05467776187827,-7.13578365451838));
#12536=CARTESIAN_POINT('Ctrl Pts',(11.9668350211294,-8.8772411146815,-9.17272232645135));
#12537=CARTESIAN_POINT('Ctrl Pts',(13.8834175105647,-9.69980446748474,-11.2096609983843));
#12538=CARTESIAN_POINT('Ctrl Pts',(15.8,-10.522367820288,-13.2465996703173));
#12539=CARTESIAN_POINT('',(10.0502525316942,-8.05467776187827,-7.13578365451838));
#12540=CARTESIAN_POINT('',(15.8,-8.20217831210975,-11.8399345109044));
#12541=CARTESIAN_POINT('Ctrl Pts',(15.8,-8.20217831210975,-11.8399345109044));
#12542=CARTESIAN_POINT('Ctrl Pts',(15.5456576615063,-8.12750458029281,-11.6096021002858));
#12543=CARTESIAN_POINT('Ctrl Pts',(15.2905271631646,-8.05247749955168,-11.3780944093842));
#12544=CARTESIAN_POINT('Ctrl Pts',(15.0353293855227,-7.97720839274395,-11.1459316587082));
#12545=CARTESIAN_POINT('Ctrl Pts',(14.7778811978172,-7.90127554051884,-10.9117216277018));
#12546=CARTESIAN_POINT('Ctrl Pts',(14.5203645390018,-7.82509615349566,-10.6768450327834));
#12547=CARTESIAN_POINT('Ctrl Pts',(14.2635195291096,-7.74879417034655,-10.4418887807018));
#12548=CARTESIAN_POINT('Ctrl Pts',(14.0000859949164,-7.6705349077066,-10.2009054892895));
#12549=CARTESIAN_POINT('Ctrl Pts',(13.7373590095418,-7.59214642417304,-9.95983851105689));
#12550=CARTESIAN_POINT('Ctrl Pts',(13.4761371226606,-7.51377627479466,-9.71937502566798));
#12551=CARTESIAN_POINT('Ctrl Pts',(13.2939627987539,-7.45912147864444,-9.55167746633259));
#12552=CARTESIAN_POINT('Ctrl Pts',(13.1125204900985,-7.40447589782759,-9.38427458086197));
#12553=CARTESIAN_POINT('Ctrl Pts',(12.9320810503802,-7.34989430276011,-9.21741359915303));
#12554=CARTESIAN_POINT('Ctrl Pts',(12.7419408661185,-7.29237830426427,-9.04158187490387));
#12555=CARTESIAN_POINT('Ctrl Pts',(12.550519923531,-7.23424116054673,-8.86418247516815));
#12556=CARTESIAN_POINT('Ctrl Pts',(12.3584607539488,-7.17554866346933,-8.68567379986729));
#12557=CARTESIAN_POINT('Ctrl Pts',(12.1609501017824,-7.11519021560012,-8.50209826451157));
#12558=CARTESIAN_POINT('Ctrl Pts',(11.9627644770494,-7.0542441495791,-8.31734966162915));
#12559=CARTESIAN_POINT('Ctrl Pts',(11.7646026923681,-6.99279967398827,-8.13197994128727));
#12560=CARTESIAN_POINT('Ctrl Pts',(11.5611700299535,-6.92972084534216,-7.9416795975511));
#12561=CARTESIAN_POINT('Ctrl Pts',(11.3577624926939,-6.8661164739041,-7.7507250000513));
#12562=CARTESIAN_POINT('Ctrl Pts',(11.1551361524457,-6.80210582000323,-7.55976563308483));
#12563=CARTESIAN_POINT('Ctrl Pts',(10.9369419552413,-6.73317720379604,-7.35413478705123));
#12564=CARTESIAN_POINT('Ctrl Pts',(10.7196536056938,-6.66377706212423,-7.14849878641362));
#12565=CARTESIAN_POINT('Ctrl Pts',(10.5042151754627,-6.59408624907933,-6.94372358733722));
#12566=CARTESIAN_POINT('Ctrl Pts',(10.3518577964671,-6.54480112569535,-6.79890721181355));
#12567=CARTESIAN_POINT('Ctrl Pts',(10.2004256127783,-6.49537136769562,-6.65452261540872));
#12568=CARTESIAN_POINT('Ctrl Pts',(10.0502525316942,-6.44587057493322,-6.51088816465466));
#12569=CARTESIAN_POINT('Ctrl Pts',(15.8,-8.20217831210975,-11.8399345109044));
#12570=CARTESIAN_POINT('Ctrl Pts',(15.8,-8.20641249422049,-11.8475125810599));
#12571=CARTESIAN_POINT('Ctrl Pts',(15.8,-8.21068161002192,-11.8550663888027));
#12572=CARTESIAN_POINT('Ctrl Pts',(15.8,-8.21498565948429,-11.862595934171));
#12573=CARTESIAN_POINT('Ctrl Pts',(15.8,-8.21932465056734,-11.8701012116266));
#12574=CARTESIAN_POINT('Ctrl Pts',(15.8,-8.22369859898568,-11.8775822089691));
#12575=CARTESIAN_POINT('Ctrl Pts',(10.0502525316942,-8.14236230483842,-4.20033906466803));
#12576=CARTESIAN_POINT('Ctrl Pts',(11.9668350211294,-9.24806690579316,-5.70883750303466));
#12577=CARTESIAN_POINT('Ctrl Pts',(13.8834175105647,-10.3537715067479,-7.21733594140129));
#12578=CARTESIAN_POINT('Ctrl Pts',(15.8,-11.4594761077026,-8.72583437976793));
#12579=CARTESIAN_POINT('Ctrl Pts',(10.0502525316942,-8.27390103242161,-4.28509982034658));
#12580=CARTESIAN_POINT('Ctrl Pts',(11.9668350211294,-9.39614075158194,-5.82139835544565));
#12581=CARTESIAN_POINT('Ctrl Pts',(13.8834175105647,-10.5187877262285,-7.35769011342039));
#12582=CARTESIAN_POINT('Ctrl Pts',(15.8,-11.6410274453888,-8.89398864851946));
#12583=CARTESIAN_POINT('Ctrl Pts',(10.0502525316942,-8.56182484570057,-4.40914912230233));
#12584=CARTESIAN_POINT('Ctrl Pts',(11.9668350211295,-9.72652656145021,-5.99475261978216));
#12585=CARTESIAN_POINT('Ctrl Pts',(13.8834175105647,-10.8916014121611,-7.57996568930606));
#12586=CARTESIAN_POINT('Ctrl Pts',(15.8,-12.0563031279108,-9.1655691867859));
#12587=CARTESIAN_POINT('Ctrl Pts',(10.0502525316941,-9.14929101108337,-4.43426842278354));
#12588=CARTESIAN_POINT('Ctrl Pts',(11.9668350211294,-10.4198746943315,-6.07716535286821));
#12589=CARTESIAN_POINT('Ctrl Pts',(13.8834175105647,-11.6903432820695,-7.72039163021283));
#12590=CARTESIAN_POINT('Ctrl Pts',(15.7999999999999,-12.9609269653176,-9.36328856029751));
#12591=CARTESIAN_POINT('Ctrl Pts',(10.0502525316942,-9.59390955692679,-4.36559112518464));
#12592=CARTESIAN_POINT('Ctrl Pts',(11.9668350211294,-10.9506581995854,-6.03655897381969));
#12593=CARTESIAN_POINT('Ctrl Pts',(13.8834175105647,-12.30814436114,-7.70675651927339));
#12594=CARTESIAN_POINT('Ctrl Pts',(15.8,-13.6648930037986,-9.37772436790844));
#12595=CARTESIAN_POINT('Ctrl Pts',(10.0502525316942,-9.86553218952113,-4.29750123086779));
#12596=CARTESIAN_POINT('Ctrl Pts',(11.9668350211294,-11.2772850923971,-5.98055897313701));
#12597=CARTESIAN_POINT('Ctrl Pts',(13.8834175105647,-12.689037995273,-7.66361671540623));
#12598=CARTESIAN_POINT('Ctrl Pts',(15.8,-14.1007908981489,-9.34667445767544));
#12599=CARTESIAN_POINT('',(10.0502525316942,-9.86553218952113,-4.29750123086779));
#12600=CARTESIAN_POINT('',(15.8,-11.4594761077026,-8.72583437976793));
#12601=CARTESIAN_POINT('Ctrl Pts',(15.8,-11.4594761077026,-8.72583437976793));
#12602=CARTESIAN_POINT('Ctrl Pts',(15.5456576332011,-11.3172805234009,-8.52985067008938));
#12603=CARTESIAN_POINT('Ctrl Pts',(15.2905271063787,-11.1743857021226,-8.33285839341101));
#12604=CARTESIAN_POINT('Ctrl Pts',(15.0353293003213,-11.0310582754433,-8.13531790820672));
#12605=CARTESIAN_POINT('Ctrl Pts',(14.777881090327,-10.8864669483792,-7.93603545706437));
#12606=CARTESIAN_POINT('Ctrl Pts',(14.5203644092926,-10.7414351729097,-7.73619524960966));
#12607=CARTESIAN_POINT('Ctrl Pts',(14.2635193774432,-10.596262186244,-7.53631716809867));
#12608=CARTESIAN_POINT('Ctrl Pts',(14.000085810689,-10.4473652525625,-7.33131185594875));
#12609=CARTESIAN_POINT('Ctrl Pts',(13.7373587930826,-10.2983195619262,-7.12626688447304));
#12610=CARTESIAN_POINT('Ctrl Pts',(13.4761368745975,-10.149477798098,-6.92179020337659));
#12611=CARTESIAN_POINT('Ctrl Pts',(13.293962634043,-10.0456766490771,-6.77918967312293));
#12612=CARTESIAN_POINT('Ctrl Pts',(13.1125204081982,-9.94197532369069,-6.63686654642483));
#12613=CARTESIAN_POINT('Ctrl Pts',(12.9320810503802,-9.83850230979698,-6.49503902755748));
#12614=CARTESIAN_POINT('Ctrl Pts',(12.7419408648011,-9.72946635277469,-6.34558654067346));
#12615=CARTESIAN_POINT('Ctrl Pts',(12.5505199208783,-9.61935521332159,-6.19483505008069));
#12616=CARTESIAN_POINT('Ctrl Pts',(12.3584607499565,-9.50837311663005,-6.0432001891388));
#12617=CARTESIAN_POINT('Ctrl Pts',(12.1609501300809,-9.39424088015611,-5.88726129158117));
#12618=CARTESIAN_POINT('Ctrl Pts',(11.9627645378641,-9.27918728833022,-5.73038832458639));
#12619=CARTESIAN_POINT('Ctrl Pts',(11.7646027855818,-9.16346774534153,-5.57307865663182));
#12620=CARTESIAN_POINT('Ctrl Pts',(11.56117018487,-9.0446702109423,-5.41158475329009));
#12621=CARTESIAN_POINT('Ctrl Pts',(11.3577627091825,-8.92517068068805,-5.24963101923163));
#12622=CARTESIAN_POINT('Ctrl Pts',(11.1551364296877,-8.80528327914643,-5.08779829683707));
#12623=CARTESIAN_POINT('Ctrl Pts',(10.9369421951543,-8.67618482323638,-4.91353182422858));
#12624=CARTESIAN_POINT('Ctrl Pts',(10.7196538081815,-8.54663632684971,-4.73940615822563));
#12625=CARTESIAN_POINT('Ctrl Pts',(10.5042153409034,-8.41707738748364,-4.56618898593399));
#12626=CARTESIAN_POINT('Ctrl Pts',(10.3518579060912,-8.32545369600363,-4.44369032369775));
#12627=CARTESIAN_POINT('Ctrl Pts',(10.2004256671345,-8.23382587572353,-4.32164700273186));
#12628=CARTESIAN_POINT('Ctrl Pts',(10.0502525316942,-8.14236230483842,-4.20033906466803));
#12629=CARTESIAN_POINT('Ctrl Pts',(15.8,-11.4594761077026,-8.72583437976793));
#12630=CARTESIAN_POINT('Ctrl Pts',(15.8,-11.4658448066529,-8.73173311854078));
#12631=CARTESIAN_POINT('Ctrl Pts',(15.8,-11.4722392320194,-8.73759798728384));
#12632=CARTESIAN_POINT('Ctrl Pts',(15.8,-11.4786593837858,-8.74342898604263));
#12633=CARTESIAN_POINT('Ctrl Pts',(15.8,-11.4851052678107,-8.74922610709021));
#12634=CARTESIAN_POINT('Ctrl Pts',(15.8,-11.4915768952696,-8.7549893339674));
#12635=CARTESIAN_POINT('Ctrl Pts',(10.0502525316942,-9.041822881172,-1.47863151154858));
#12636=CARTESIAN_POINT('Ctrl Pts',(11.9668350211294,-10.5595621004509,-2.57161726872464));
#12637=CARTESIAN_POINT('Ctrl Pts',(13.8834175105647,-12.0773013197298,-3.66460302590071));
#12638=CARTESIAN_POINT('Ctrl Pts',(15.8,-13.5950405390087,-4.75758878307678));
#12639=CARTESIAN_POINT('Ctrl Pts',(10.0502525316942,-9.19311615914592,-1.5185960783211));
#12640=CARTESIAN_POINT('Ctrl Pts',(11.9668350211294,-10.7351719126775,-2.63291166611866));
#12641=CARTESIAN_POINT('Ctrl Pts',(13.8834175105647,-12.2776128949465,-3.74709495962168));
#12642=CARTESIAN_POINT('Ctrl Pts',(15.8,-13.8196686484781,-4.86141054741924));
#12643=CARTESIAN_POINT('Ctrl Pts',(10.0502525316942,-9.50527827631687,-1.54760878347554));
#12644=CARTESIAN_POINT('Ctrl Pts',(11.9668350211294,-11.1029538596823,-2.69569469846983));
#12645=CARTESIAN_POINT('Ctrl Pts',(13.8834175105647,-12.7008586295609,-3.84329897549064));
#12646=CARTESIAN_POINT('Ctrl Pts',(15.8,-14.2985342129264,-4.99138489048493));
#12647=CARTESIAN_POINT('Ctrl Pts',(10.0502525316941,-10.0717544060046,-1.38996253959751));
#12648=CARTESIAN_POINT('Ctrl Pts',(11.9668350211294,-11.7878343688586,-2.55981841965666));
#12649=CARTESIAN_POINT('Ctrl Pts',(13.8834175105647,-13.5039013178588,-3.73002877331942));
#12650=CARTESIAN_POINT('Ctrl Pts',(15.7999999999999,-15.2199812807128,-4.89988465337858));
#12651=CARTESIAN_POINT('Ctrl Pts',(10.0502525316942,-10.473392049036,-1.18724279150055));
#12652=CARTESIAN_POINT('Ctrl Pts',(11.9668350211294,-12.2800941488934,-2.35716926478797));
#12653=CARTESIAN_POINT('Ctrl Pts',(13.8834175105647,-14.0872596341291,-3.52613523034269));
#12654=CARTESIAN_POINT('Ctrl Pts',(15.8,-15.8939617339865,-4.6960617036301));
#12655=CARTESIAN_POINT('Ctrl Pts',(10.0502525316942,-10.7106795892491,-1.03854944428814));
#12656=CARTESIAN_POINT('Ctrl Pts',(11.9668350211294,-12.5734298318033,-2.20297683852746));
#12657=CARTESIAN_POINT('Ctrl Pts',(13.8834175105647,-14.4361800743576,-3.36740423276678));
#12658=CARTESIAN_POINT('Ctrl Pts',(15.8,-16.2989303169119,-4.5318316270061));
#12659=CARTESIAN_POINT('',(10.0502525316942,-10.7106795892491,-1.03854944428814));
#12660=CARTESIAN_POINT('',(15.8,-13.5950405390087,-4.75758878307678));
#12661=CARTESIAN_POINT('Ctrl Pts',(15.8,-13.5950405390087,-4.75758878307678));
#12662=CARTESIAN_POINT('Ctrl Pts',(15.5456573899571,-13.3992420178043,-4.61513791473879));
#12663=CARTESIAN_POINT('Ctrl Pts',(15.2905266183831,-13.202466813867,-4.47194392111198));
#12664=CARTESIAN_POINT('Ctrl Pts',(15.0353285681349,-13.0051107697481,-4.32836223491455));
#12665=CARTESIAN_POINT('Ctrl Pts',(14.7778801662826,-12.8060144282797,-4.18351443685803));
#12666=CARTESIAN_POINT('Ctrl Pts',(14.52036329399,-12.6063268373513,-4.03827228948993));
#12667=CARTESIAN_POINT('Ctrl Pts',(14.2635180731355,-12.4064932437265,-3.89303775923306));
#12668=CARTESIAN_POINT('Ctrl Pts',(14.0000842255552,-12.2015334929893,-3.74407765407785));
#12669=CARTESIAN_POINT('Ctrl Pts',(13.7373569299596,-11.9964200114439,-3.59512579987346));
#12670=CARTESIAN_POINT('Ctrl Pts',(13.4761347388971,-11.7916760912341,-3.44665140507749));
#12671=CARTESIAN_POINT('Ctrl Pts',(13.2939612159639,-11.6488899018523,-3.34310697244201));
#12672=CARTESIAN_POINT('Ctrl Pts',(13.1125197030777,-11.5062843729557,-3.2397955167614));
#12673=CARTESIAN_POINT('Ctrl Pts',(12.9320810503802,-11.3640491305165,-3.13688485529761));
#12674=CARTESIAN_POINT('Ctrl Pts',(12.7419408532673,-11.2141664051165,-3.02844105368848));
#12675=CARTESIAN_POINT('Ctrl Pts',(12.5505198976554,-11.0628597070356,-2.91909407414931));
#12676=CARTESIAN_POINT('Ctrl Pts',(12.358460715006,-10.9104517039513,-2.80917609774724));
#12677=CARTESIAN_POINT('Ctrl Pts',(12.1609503726544,-10.7537179490168,-2.69613835151564));
#12678=CARTESIAN_POINT('Ctrl Pts',(11.9627650599002,-10.5958192942297,-2.58249696621042));
#12679=CARTESIAN_POINT('Ctrl Pts',(11.7646035860725,-10.4371523366737,-2.46864604141714));
#12680=CARTESIAN_POINT('Ctrl Pts',(11.5611715157468,-10.2742652373582,-2.35176696854891));
#12681=CARTESIAN_POINT('Ctrl Pts',(11.3577645693228,-10.1105684093216,-2.23466749726794));
#12682=CARTESIAN_POINT('Ctrl Pts',(11.1551388120544,-9.94654008829804,-2.11780296935768));
#12683=CARTESIAN_POINT('Ctrl Pts',(10.9369442531875,-9.7699086095073,-1.99195912572045));
#12684=CARTESIAN_POINT('Ctrl Pts',(10.7196555410835,-9.59289262515041,-1.86638826421794));
#12685=CARTESIAN_POINT('Ctrl Pts',(10.5042167520009,-9.41614744679567,-1.74168466284111));
#12686=CARTESIAN_POINT('Ctrl Pts',(10.3518588411102,-9.29115358543579,-1.65349450791485));
#12687=CARTESIAN_POINT('Ctrl Pts',(10.2004261307569,-9.16629650496048,-1.56573868767379));
#12688=CARTESIAN_POINT('Ctrl Pts',(10.0502525316942,-9.041822881172,-1.47863151154858));
#12689=CARTESIAN_POINT('Ctrl Pts',(15.8,-13.5950405390087,-4.75758878307678));
#12690=CARTESIAN_POINT('Ctrl Pts',(15.8,-13.6029203421718,-4.76123078081695));
#12691=CARTESIAN_POINT('Ctrl Pts',(15.8,-13.610814146196,-4.76483261634472));
#12692=CARTESIAN_POINT('Ctrl Pts',(15.8,-13.6187219510797,-4.7683942897085));
#12693=CARTESIAN_POINT('Ctrl Pts',(15.8,-13.626643760007,-4.77191579174908));
#12694=CARTESIAN_POINT('Ctrl Pts',(15.8,-13.6345795785203,-4.77539710335946));
#12695=CARTESIAN_POINT('Ctrl Pts',(10.0502525316942,-9.05620683581208,1.38781479615277));
#12696=CARTESIAN_POINT('Ctrl Pts',(11.9668350211294,-10.8374137839212,0.817330781359223));
#12697=CARTESIAN_POINT('Ctrl Pts',(13.8834175105647,-12.6186207320302,0.246846766565676));
#12698=CARTESIAN_POINT('Ctrl Pts',(15.8,-14.3998276801393,-0.32363724822787));
#12699=CARTESIAN_POINT('Ctrl Pts',(10.0502525316942,-9.21244502400637,1.39655842853148));
#12700=CARTESIAN_POINT('Ctrl Pts',(11.9668350211294,-11.0233696506194,0.813302761662288));
#12701=CARTESIAN_POINT('Ctrl Pts',(13.8834175105647,-12.8346197703481,0.230291956370553));
#12702=CARTESIAN_POINT('Ctrl Pts',(15.8,-14.6455443969611,-0.352963710498644));
#12703=CARTESIAN_POINT('Ctrl Pts',(10.0502525316942,-9.51829373400973,1.46541714813614));
#12704=CARTESIAN_POINT('Ctrl Pts',(11.9668350211295,-11.3925515672309,0.867231464171976));
#12705=CARTESIAN_POINT('Ctrl Pts',(13.8834175105647,-13.2668740653714,0.269566015193986));
#12706=CARTESIAN_POINT('Ctrl Pts',(15.8,-15.1411318985925,-0.32861966877018));
#12707=CARTESIAN_POINT('Ctrl Pts',(10.0502525316941,-10.0083300006652,1.79039750449509));
#12708=CARTESIAN_POINT('Ctrl Pts',(11.9668350211294,-12.0019243797287,1.20809631886684));
#12709=CARTESIAN_POINT('Ctrl Pts',(13.8834175105647,-13.9956114385882,0.625444427693871));
#12710=CARTESIAN_POINT('Ctrl Pts',(15.8,-15.9892058176518,0.0431432420656217));
#12711=CARTESIAN_POINT('Ctrl Pts',(10.0502525316942,-10.3276659549724,2.10732113862255));
#12712=CARTESIAN_POINT('Ctrl Pts',(11.9668350211294,-12.4074689224609,1.55295659524519));
#12713=CARTESIAN_POINT('Ctrl Pts',(13.8834175105647,-14.4874157824203,0.999648742962749));
#12714=CARTESIAN_POINT('Ctrl Pts',(15.8,-16.5672187499088,0.445284199585382));
#12715=CARTESIAN_POINT('Ctrl Pts',(10.0502525316942,-10.5073910450885,2.32206279789789));
#12716=CARTESIAN_POINT('Ctrl Pts',(11.9668350211294,-12.6387996550358,1.79024801807933));
#12717=CARTESIAN_POINT('Ctrl Pts',(13.8834175105647,-14.7702082649831,1.25843323826077));
#12718=CARTESIAN_POINT('Ctrl Pts',(15.8,-16.9016168749304,0.7266184584422));
#12719=CARTESIAN_POINT('',(10.0502525316942,-10.5073910450885,2.32206279789789));
#12720=CARTESIAN_POINT('',(15.8,-14.3998276801393,-0.32363724822787));
#12721=CARTESIAN_POINT('Ctrl Pts',(15.8,-14.3998276801393,-0.32363724822787));
#12722=CARTESIAN_POINT('Ctrl Pts',(15.4361339239126,-14.0704500021455,-0.216378749849824));
#12723=CARTESIAN_POINT('Ctrl Pts',(15.0706551397176,-13.7385848339403,-0.108278411513937));
#12724=CARTESIAN_POINT('Ctrl Pts',(14.7056733117528,-13.405863146671,8.83803447093712E-12));
#12725=CARTESIAN_POINT('Ctrl Pts',(15.8,-14.3998276801393,-0.32363724822787));
#12726=CARTESIAN_POINT('Ctrl Pts',(15.8,-14.4084472574799,-0.324666000821258));
#12727=CARTESIAN_POINT('Ctrl Pts',(15.8,-14.4170677396245,-0.325652230376828));
#12728=CARTESIAN_POINT('Ctrl Pts',(15.8,-14.4256891265865,-0.326595936941116));
#12729=CARTESIAN_POINT('Ctrl Pts',(15.8,-14.434311418564,-0.327497110819208));
#12730=CARTESIAN_POINT('Ctrl Pts',(15.8,-14.4429346149236,-0.328355732126618));
#12731=CARTESIAN_POINT('Ctrl Pts',(10.0502525316942,-8.18410616705958,4.11841212213242));
#12732=CARTESIAN_POINT('Ctrl Pts',(11.9668350211294,-10.0544238975194,4.12627279988524));
#12733=CARTESIAN_POINT('Ctrl Pts',(13.8834175105647,-11.9247416279792,4.13413347763806));
#12734=CARTESIAN_POINT('Ctrl Pts',(15.8,-13.795059358439,4.14199415539088));
#12735=CARTESIAN_POINT('Ctrl Pts',(10.0502525316942,-8.32999558303832,4.17500806600467));
#12736=CARTESIAN_POINT('Ctrl Pts',(11.9668350211294,-10.2325231628261,4.17990544851818));
#12737=CARTESIAN_POINT('Ctrl Pts',(13.8834175105647,-12.1352846385738,4.18513629113482));
#12738=CARTESIAN_POINT('Ctrl Pts',(15.8,-14.0378122183616,4.19003367364834));
#12739=CARTESIAN_POINT('Ctrl Pts',(10.0502525316942,-8.59959242261694,4.33502367302149));
#12740=CARTESIAN_POINT('Ctrl Pts',(11.9668350211295,-10.5669670902559,4.34529280263859));
#12741=CARTESIAN_POINT('Ctrl Pts',(13.8834175105647,-12.5342444956751,4.3560888733651));
#12742=CARTESIAN_POINT('Ctrl Pts',(15.8,-14.5016191633141,4.36635800298221));
#12743=CARTESIAN_POINT('Ctrl Pts',(10.0502525316941,-8.9652188127798,4.79552866926091));
#12744=CARTESIAN_POINT('Ctrl Pts',(11.9668350211294,-11.0411807000414,4.85778187524378));
#12745=CARTESIAN_POINT('Ctrl Pts',(13.8834175105647,-13.1173407686982,4.91974349130655));
#12746=CARTESIAN_POINT('Ctrl Pts',(15.8,-15.1933026559598,4.98199669728942));
#12747=CARTESIAN_POINT('Ctrl Pts',(10.0502525316942,-9.17099596015618,5.19560579312754));
#12748=CARTESIAN_POINT('Ctrl Pts',(11.9668350211294,-11.3203141899786,5.3110682436509));
#12749=CARTESIAN_POINT('Ctrl Pts',(13.8834175105647,-13.4694427341669,5.42758013234469));
#12750=CARTESIAN_POINT('Ctrl Pts',(15.8,-15.6187609639894,5.54304258286804));
#12751=CARTESIAN_POINT('Ctrl Pts',(10.0502525316942,-9.2755658561365,5.45537535466284));
#12752=CARTESIAN_POINT('Ctrl Pts',(11.9668350211294,-11.4669957083382,5.60823092528512));
#12753=CARTESIAN_POINT('Ctrl Pts',(13.8834175105647,-13.6584255605399,5.76108649590741));
#12754=CARTESIAN_POINT('Ctrl Pts',(15.8,-15.8498554127416,5.91394206652969));
#12755=CARTESIAN_POINT('',(10.0502525316942,-9.2755658561365,5.45537535466284));
#12756=CARTESIAN_POINT('',(15.8,-13.795059358439,4.14199415539088));
#12757=CARTESIAN_POINT('Ctrl Pts',(15.8,-13.795059358439,4.14199415539088));
#12758=CARTESIAN_POINT('Ctrl Pts',(15.5456574794164,-13.5529245928913,4.14215184549968));
#12759=CARTESIAN_POINT('Ctrl Pts',(15.2905267978562,-13.3095628770609,4.14233665870497));
#12760=CARTESIAN_POINT('Ctrl Pts',(15.0353288374156,-13.0655033718482,4.14249371366664));
#12761=CARTESIAN_POINT('Ctrl Pts',(14.7778805061931,-12.8192917162866,4.1426521535606));
#12762=CARTESIAN_POINT('Ctrl Pts',(14.5203637043096,-12.572369937213,4.14278210218064));
#12763=CARTESIAN_POINT('Ctrl Pts',(14.2635185530351,-12.3253345162694,4.14282007025482));
#12764=CARTESIAN_POINT('Ctrl Pts',(14.0000848089512,-12.0719621417566,4.14285901228618));
#12765=CARTESIAN_POINT('Ctrl Pts',(13.7373576158074,-11.8184702457667,4.14280091850188));
#12766=CARTESIAN_POINT('Ctrl Pts',(13.476135525203,-11.5655579735775,4.14257377376942));
#12767=CARTESIAN_POINT('Ctrl Pts',(13.2939617380614,-11.3891793743072,4.14241536520586));
#12768=CARTESIAN_POINT('Ctrl Pts',(13.1125199626836,-11.2130838733106,4.14217466317553));
#12769=CARTESIAN_POINT('Ctrl Pts',(12.9320810503802,-11.0375235228707,4.14182735974364));
#12770=CARTESIAN_POINT('Ctrl Pts',(12.7419408575533,-10.8525241873102,4.14146138357661));
#12771=CARTESIAN_POINT('Ctrl Pts',(12.5505199062851,-10.6658419590997,4.14098910290386));
#12772=CARTESIAN_POINT('Ctrl Pts',(12.3584607279937,-10.4779331330946,4.14033143664814));
#12773=CARTESIAN_POINT('Ctrl Pts',(12.1609502835666,-10.2846908414935,4.13965510367824));
#12774=CARTESIAN_POINT('Ctrl Pts',(11.9627648680236,-10.0901513147874,4.13878241284078));
#12775=CARTESIAN_POINT('Ctrl Pts',(11.7646032917777,-9.89486705366043,4.13762764472382));
#12776=CARTESIAN_POINT('Ctrl Pts',(11.5611710263552,-9.69438863400392,4.13644216215692));
#12777=CARTESIAN_POINT('Ctrl Pts',(11.3577638852471,-9.49312558221608,4.1349590374594));
#12778=CARTESIAN_POINT('Ctrl Pts',(11.1551379358829,-9.29173244420307,4.1330909916179));
#12779=CARTESIAN_POINT('Ctrl Pts',(10.9369434970465,-9.07486553810268,4.13107941701265));
#12780=CARTESIAN_POINT('Ctrl Pts',(10.7196549052601,-8.85784801697426,4.12862098831913));
#12781=CARTESIAN_POINT('Ctrl Pts',(10.5042162352556,-8.64155934493263,4.12562010893634));
#12782=CARTESIAN_POINT('Ctrl Pts',(10.3518584987053,-8.48860048887835,4.12349789387433));
#12783=CARTESIAN_POINT('Ctrl Pts',(10.2004259609779,-8.3360075858186,4.1211046936333));
#12784=CARTESIAN_POINT('Ctrl Pts',(10.0502525316942,-8.18410616705958,4.11841212213242));
#12785=CARTESIAN_POINT('Ctrl Pts',(15.8,-13.795059358439,4.14199415539088));
#12786=CARTESIAN_POINT('Ctrl Pts',(15.8,-13.8035749656708,4.14367934941586));
#12787=CARTESIAN_POINT('Ctrl Pts',(15.8,-13.8120782930811,4.14540526485286));
#12788=CARTESIAN_POINT('Ctrl Pts',(15.8,-13.8205693406969,4.14717190166177));
#12789=CARTESIAN_POINT('Ctrl Pts',(15.8,-13.8290481057107,4.14897926912419));
#12790=CARTESIAN_POINT('Ctrl Pts',(15.8,-13.8375145813754,4.15082738595568));
#12791=CARTESIAN_POINT('Ctrl Pts',(10.0502525316942,-6.51088816465466,6.44587057493322));
#12792=CARTESIAN_POINT('Ctrl Pts',(11.9668350211294,-8.28723694673789,7.03130648732539));
#12793=CARTESIAN_POINT('Ctrl Pts',(13.8834175105647,-10.0635857288211,7.61674239971757));
#12794=CARTESIAN_POINT('Ctrl Pts',(15.8,-11.8399345109044,8.20217831210975));
#12795=CARTESIAN_POINT('Ctrl Pts',(10.0502525316942,-6.63214813591052,6.54477882498566));
#12796=CARTESIAN_POINT('Ctrl Pts',(11.9668350211294,-8.4400460136743,7.13734986695939));
#12797=CARTESIAN_POINT('Ctrl Pts',(13.8834175105647,-10.2480632948761,7.73031032616364));
#12798=CARTESIAN_POINT('Ctrl Pts',(15.8,-12.0559611726399,8.32288136813736));
#12799=CARTESIAN_POINT('Ctrl Pts',(10.0502525316942,-6.83909882511009,6.78027814405441));
#12800=CARTESIAN_POINT('Ctrl Pts',(11.9668350211295,-8.70700998719297,7.39799687329663));
#12801=CARTESIAN_POINT('Ctrl Pts',(13.8834175105647,-10.5746650104356,8.01619193743949));
#12802=CARTESIAN_POINT('Ctrl Pts',(15.8,-12.4425761725185,8.6339106666817));
#12803=CARTESIAN_POINT('Ctrl Pts',(10.0502525316941,-7.04452561799895,7.33122941665115));
#12804=CARTESIAN_POINT('Ctrl Pts',(11.9668350211294,-8.99964539985646,8.03194323669995));
#12805=CARTESIAN_POINT('Ctrl Pts',(13.8834175105647,-10.9550426722922,8.73244671395173));
#12806=CARTESIAN_POINT('Ctrl Pts',(15.8,-12.9101624541497,9.43316053400054));
#12807=CARTESIAN_POINT('Ctrl Pts',(10.0502525316942,-7.11660498267375,7.77530835268703));
#12808=CARTESIAN_POINT('Ctrl Pts',(11.9668350211294,-9.12504823131445,8.54929552797968));
#12809=CARTESIAN_POINT('Ctrl Pts',(13.8834175105647,-11.1329867839675,9.32422216219831));
#12810=CARTESIAN_POINT('Ctrl Pts',(15.8,-13.1414300326082,10.098209337491));
#12811=CARTESIAN_POINT('Ctrl Pts',(10.0502525316942,-7.13578365451838,8.05467776187827));
#12812=CARTESIAN_POINT('Ctrl Pts',(11.9668350211294,-9.17272232645135,8.8772411146815));
#12813=CARTESIAN_POINT('Ctrl Pts',(13.8834175105647,-11.2096609983843,9.69980446748474));
#12814=CARTESIAN_POINT('Ctrl Pts',(15.8,-13.2465996703173,10.522367820288));
#12815=CARTESIAN_POINT('',(10.0502525316942,-7.13578365451838,8.05467776187827));
#12816=CARTESIAN_POINT('',(15.8,-11.8399345109044,8.20217831210975));
#12817=CARTESIAN_POINT('Ctrl Pts',(15.8,-11.8399345109044,8.20217831210975));
#12818=CARTESIAN_POINT('Ctrl Pts',(15.5456576615071,-11.6096021002865,8.12750458029304));
#12819=CARTESIAN_POINT('Ctrl Pts',(15.2905271631662,-11.3780944093856,8.05247749955213));
#12820=CARTESIAN_POINT('Ctrl Pts',(15.035329385525,-11.1459316587103,7.97720839274464));
#12821=CARTESIAN_POINT('Ctrl Pts',(14.77788119782,-10.9117216277044,7.90127554051966));
#12822=CARTESIAN_POINT('Ctrl Pts',(14.5203645390051,-10.6768450327863,7.82509615349662));
#12823=CARTESIAN_POINT('Ctrl Pts',(14.2635195291132,-10.4418887807051,7.74879417034763));
#12824=CARTESIAN_POINT('Ctrl Pts',(14.0000859949203,-10.2009054892931,7.67053490770775));
#12825=CARTESIAN_POINT('Ctrl Pts',(13.7373590095459,-9.95983851106062,7.59214642417425));
#12826=CARTESIAN_POINT('Ctrl Pts',(13.4761371226649,-9.71937502567191,7.51377627479595));
#12827=CARTESIAN_POINT('Ctrl Pts',(13.2939627987567,-9.5516774663352,7.45912147864529));
#12828=CARTESIAN_POINT('Ctrl Pts',(13.1125204900999,-9.38427458086327,7.40447589782802));
#12829=CARTESIAN_POINT('Ctrl Pts',(12.9320810503802,-9.21741359915303,7.34989430276011));
#12830=CARTESIAN_POINT('Ctrl Pts',(12.7419408661181,-9.04158187490351,7.29237830426415));
#12831=CARTESIAN_POINT('Ctrl Pts',(12.5505199235302,-8.86418247516742,7.23424116054649));
#12832=CARTESIAN_POINT('Ctrl Pts',(12.3584607539476,-8.68567379986618,7.17554866346896));
#12833=CARTESIAN_POINT('Ctrl Pts',(12.1609501017812,-8.50209826451042,7.11519021559974));
#12834=CARTESIAN_POINT('Ctrl Pts',(11.9627644770481,-8.31734966162796,7.0542441495787));
#12835=CARTESIAN_POINT('Ctrl Pts',(11.7646026923668,-8.13197994128604,6.99279967398786));
#12836=CARTESIAN_POINT('Ctrl Pts',(11.5611700299521,-7.94167959754981,6.92972084534173));
#12837=CARTESIAN_POINT('Ctrl Pts',(11.3577624926924,-7.75072500004995,6.86611647390365));
#12838=CARTESIAN_POINT('Ctrl Pts',(11.1551361524442,-7.55976563308342,6.80210582000276));
#12839=CARTESIAN_POINT('Ctrl Pts',(10.9369419552397,-7.35413478704973,6.73317720379554));
#12840=CARTESIAN_POINT('Ctrl Pts',(10.7196536056921,-7.14849878641203,6.66377706212369));
#12841=CARTESIAN_POINT('Ctrl Pts',(10.5042151754609,-6.94372358733556,6.59408624907876));
#12842=CARTESIAN_POINT('Ctrl Pts',(10.3518577964659,-6.79890721181244,6.54480112569497));
#12843=CARTESIAN_POINT('Ctrl Pts',(10.2004256127777,-6.65452261540817,6.49537136769543));
#12844=CARTESIAN_POINT('Ctrl Pts',(10.0502525316942,-6.51088816465466,6.44587057493322));
#12845=CARTESIAN_POINT('Ctrl Pts',(15.8,-11.8399345109044,8.20217831210975));
#12846=CARTESIAN_POINT('Ctrl Pts',(15.8,-11.8475125810599,8.20641249422049));
#12847=CARTESIAN_POINT('Ctrl Pts',(15.8,-11.8550663888027,8.21068161002192));
#12848=CARTESIAN_POINT('Ctrl Pts',(15.8,-11.862595934171,8.21498565948429));
#12849=CARTESIAN_POINT('Ctrl Pts',(15.8,-11.8701012116266,8.21932465056734));
#12850=CARTESIAN_POINT('Ctrl Pts',(15.8,-11.8775822089691,8.22369859898568));
#12851=CARTESIAN_POINT('Ctrl Pts',(10.0502525316942,-4.20033906466803,8.14236230483842));
#12852=CARTESIAN_POINT('Ctrl Pts',(11.9668350211294,-5.70883750303466,9.24806690579316));
#12853=CARTESIAN_POINT('Ctrl Pts',(13.8834175105647,-7.21733594140129,10.3537715067479));
#12854=CARTESIAN_POINT('Ctrl Pts',(15.8,-8.72583437976793,11.4594761077026));
#12855=CARTESIAN_POINT('Ctrl Pts',(10.0502525316942,-4.28509982034658,8.27390103242161));
#12856=CARTESIAN_POINT('Ctrl Pts',(11.9668350211294,-5.82139835544565,9.39614075158194));
#12857=CARTESIAN_POINT('Ctrl Pts',(13.8834175105647,-7.35769011342039,10.5187877262285));
#12858=CARTESIAN_POINT('Ctrl Pts',(15.8,-8.89398864851946,11.6410274453888));
#12859=CARTESIAN_POINT('Ctrl Pts',(10.0502525316942,-4.40914912230232,8.56182484570054));
#12860=CARTESIAN_POINT('Ctrl Pts',(11.9668350211295,-5.99475261978216,9.72652656145018));
#12861=CARTESIAN_POINT('Ctrl Pts',(13.8834175105647,-7.57996568930604,10.8916014121611));
#12862=CARTESIAN_POINT('Ctrl Pts',(15.8,-9.16556918678588,12.0563031279108));
#12863=CARTESIAN_POINT('Ctrl Pts',(10.0502525316941,-4.43426842278354,9.14929101108337));
#12864=CARTESIAN_POINT('Ctrl Pts',(11.9668350211294,-6.07716535286821,10.4198746943315));
#12865=CARTESIAN_POINT('Ctrl Pts',(13.8834175105647,-7.72039163021281,11.6903432820695));
#12866=CARTESIAN_POINT('Ctrl Pts',(15.8,-9.36328856029748,12.9609269653176));
#12867=CARTESIAN_POINT('Ctrl Pts',(10.0502525316942,-4.36559112518463,9.59390955692677));
#12868=CARTESIAN_POINT('Ctrl Pts',(11.9668350211294,-6.03655897381968,10.9506581995853));
#12869=CARTESIAN_POINT('Ctrl Pts',(13.8834175105647,-7.70675651927341,12.30814436114));
#12870=CARTESIAN_POINT('Ctrl Pts',(15.8,-9.37772436790846,13.6648930037986));
#12871=CARTESIAN_POINT('Ctrl Pts',(10.0502525316942,-4.29750123086779,9.86553218952113));
#12872=CARTESIAN_POINT('Ctrl Pts',(11.9668350211294,-5.98055897313701,11.2772850923971));
#12873=CARTESIAN_POINT('Ctrl Pts',(13.8834175105647,-7.66361671540623,12.689037995273));
#12874=CARTESIAN_POINT('Ctrl Pts',(15.8,-9.34667445767544,14.1007908981489));
#12875=CARTESIAN_POINT('',(10.0502525316942,-4.29750123086779,9.86553218952113));
#12876=CARTESIAN_POINT('',(15.8,-8.72583437976793,11.4594761077026));
#12877=CARTESIAN_POINT('Ctrl Pts',(15.8,-8.72583437976793,11.4594761077026));
#12878=CARTESIAN_POINT('Ctrl Pts',(15.5456576332007,-8.5298506700891,11.3172805234007));
#12879=CARTESIAN_POINT('Ctrl Pts',(15.2905271063779,-8.33285839341041,11.1743857021221));
#12880=CARTESIAN_POINT('Ctrl Pts',(15.0353293003201,-8.13531790820579,11.0310582754426));
#12881=CARTESIAN_POINT('Ctrl Pts',(14.7778810903262,-7.93603545706372,10.8864669483788));
#12882=CARTESIAN_POINT('Ctrl Pts',(14.5203644092921,-7.73619524960928,10.7414351729094));
#12883=CARTESIAN_POINT('Ctrl Pts',(14.2635193774431,-7.53631716809856,10.5962621862439));
#12884=CARTESIAN_POINT('Ctrl Pts',(14.0000858106901,-7.33131185594961,10.4473652525631));
#12885=CARTESIAN_POINT('Ctrl Pts',(13.7373587930849,-7.12626688447486,10.2983195619276));
#12886=CARTESIAN_POINT('Ctrl Pts',(13.4761368746011,-6.92179020337937,10.1494777981));
#12887=CARTESIAN_POINT('Ctrl Pts',(13.2939626340454,-6.77918967312477,10.0456766490784));
#12888=CARTESIAN_POINT('Ctrl Pts',(13.1125204081994,-6.63686654642574,9.94197532369136));
#12889=CARTESIAN_POINT('Ctrl Pts',(12.9320810503802,-6.49503902755748,9.83850230979699));
#12890=CARTESIAN_POINT('Ctrl Pts',(12.7419408648006,-6.34558654067311,9.72946635277443));
#12891=CARTESIAN_POINT('Ctrl Pts',(12.5505199208774,-6.19483505007998,9.61935521332108));
#12892=CARTESIAN_POINT('Ctrl Pts',(12.3584607499551,-6.04320018913773,9.50837311662927));
#12893=CARTESIAN_POINT('Ctrl Pts',(12.1609501300796,-5.88726129158013,9.39424088015534));
#12894=CARTESIAN_POINT('Ctrl Pts',(11.9627645378628,-5.73038832458536,9.27918728832947));
#12895=CARTESIAN_POINT('Ctrl Pts',(11.7646027855805,-5.57307865663081,9.16346774534079));
#12896=CARTESIAN_POINT('Ctrl Pts',(11.5611701848687,-5.41158475328911,9.04467021094158));
#12897=CARTESIAN_POINT('Ctrl Pts',(11.3577627091813,-5.24963101923067,8.92517068068734));
#12898=CARTESIAN_POINT('Ctrl Pts',(11.1551364296865,-5.08779829683614,8.80528327914573));
#12899=CARTESIAN_POINT('Ctrl Pts',(10.9369421951531,-4.91353182422761,8.67618482323567));
#12900=CARTESIAN_POINT('Ctrl Pts',(10.7196538081802,-4.73940615822464,8.54663632684897));
#12901=CARTESIAN_POINT('Ctrl Pts',(10.5042153409022,-4.56618898593296,8.41707738748288));
#12902=CARTESIAN_POINT('Ctrl Pts',(10.3518579060903,-4.44369032369707,8.32545369600313));
#12903=CARTESIAN_POINT('Ctrl Pts',(10.2004256671341,-4.32164700273153,8.23382587572327));
#12904=CARTESIAN_POINT('Ctrl Pts',(10.0502525316942,-4.20033906466803,8.14236230483842));
#12905=CARTESIAN_POINT('Ctrl Pts',(15.8,-8.72583437976793,11.4594761077026));
#12906=CARTESIAN_POINT('Ctrl Pts',(15.8,-8.73173311854078,11.4658448066529));
#12907=CARTESIAN_POINT('Ctrl Pts',(15.8,-8.73759798728384,11.4722392320194));
#12908=CARTESIAN_POINT('Ctrl Pts',(15.8,-8.74342898604263,11.4786593837858));
#12909=CARTESIAN_POINT('Ctrl Pts',(15.8,-8.7492261070902,11.4851052678107));
#12910=CARTESIAN_POINT('Ctrl Pts',(15.8,-8.7549893339674,11.4915768952696));
#12911=CARTESIAN_POINT('Ctrl Pts',(10.0502525316942,-1.47863151154858,9.041822881172));
#12912=CARTESIAN_POINT('Ctrl Pts',(11.9668350211294,-2.57161726872465,10.5595621004509));
#12913=CARTESIAN_POINT('Ctrl Pts',(13.8834175105647,-3.66460302590071,12.0773013197298));
#12914=CARTESIAN_POINT('Ctrl Pts',(15.8,-4.75758878307678,13.5950405390087));
#12915=CARTESIAN_POINT('Ctrl Pts',(10.0502525316942,-1.5185960783211,9.19311615914592));
#12916=CARTESIAN_POINT('Ctrl Pts',(11.9668350211294,-2.63291166611866,10.7351719126775));
#12917=CARTESIAN_POINT('Ctrl Pts',(13.8834175105647,-3.74709495962167,12.2776128949465));
#12918=CARTESIAN_POINT('Ctrl Pts',(15.8,-4.86141054741923,13.8196686484781));
#12919=CARTESIAN_POINT('Ctrl Pts',(10.0502525316942,-1.54760878347554,9.50527827631687));
#12920=CARTESIAN_POINT('Ctrl Pts',(11.9668350211295,-2.69569469846983,11.1029538596823));
#12921=CARTESIAN_POINT('Ctrl Pts',(13.8834175105647,-3.84329897549064,12.7008586295609));
#12922=CARTESIAN_POINT('Ctrl Pts',(15.8,-4.99138489048493,14.2985342129264));
#12923=CARTESIAN_POINT('Ctrl Pts',(10.0502525316941,-1.38996253959751,10.0717544060046));
#12924=CARTESIAN_POINT('Ctrl Pts',(11.9668350211294,-2.55981841965666,11.7878343688586));
#12925=CARTESIAN_POINT('Ctrl Pts',(13.8834175105647,-3.73002877331942,13.5039013178589));
#12926=CARTESIAN_POINT('Ctrl Pts',(15.8,-4.89988465337857,15.2199812807128));
#12927=CARTESIAN_POINT('Ctrl Pts',(10.0502525316942,-1.18724279150055,10.473392049036));
#12928=CARTESIAN_POINT('Ctrl Pts',(11.9668350211294,-2.35716926478797,12.2800941488934));
#12929=CARTESIAN_POINT('Ctrl Pts',(13.8834175105647,-3.52613523034269,14.0872596341291));
#12930=CARTESIAN_POINT('Ctrl Pts',(15.8,-4.69606170363011,15.8939617339865));
#12931=CARTESIAN_POINT('Ctrl Pts',(10.0502525316942,-1.03854944428814,10.7106795892491));
#12932=CARTESIAN_POINT('Ctrl Pts',(11.9668350211294,-2.20297683852746,12.5734298318033));
#12933=CARTESIAN_POINT('Ctrl Pts',(13.8834175105647,-3.36740423276678,14.4361800743576));
#12934=CARTESIAN_POINT('Ctrl Pts',(15.8,-4.5318316270061,16.2989303169119));
#12935=CARTESIAN_POINT('',(10.0502525316942,-1.03854944428814,10.7106795892491));
#12936=CARTESIAN_POINT('',(15.8,-4.75758878307678,13.5950405390087));
#12937=CARTESIAN_POINT('Ctrl Pts',(15.8,-4.75758878307678,13.5950405390087));
#12938=CARTESIAN_POINT('Ctrl Pts',(15.5456573899559,-4.61513791473816,13.3992420178034));
#12939=CARTESIAN_POINT('Ctrl Pts',(15.2905266183809,-4.47194392111073,13.2024668138653));
#12940=CARTESIAN_POINT('Ctrl Pts',(15.0353285681316,-4.32836223491271,13.0051107697455));
#12941=CARTESIAN_POINT('Ctrl Pts',(14.7778801662812,-4.18351443685719,12.8060144282785));
#12942=CARTESIAN_POINT('Ctrl Pts',(14.5203632939904,-4.03827228949013,12.6063268373516));
#12943=CARTESIAN_POINT('Ctrl Pts',(14.2635180731377,-3.89303775923429,12.4064932437282));
#12944=CARTESIAN_POINT('Ctrl Pts',(14.0000842255574,-3.74407765407913,12.201533492991));
#12945=CARTESIAN_POINT('Ctrl Pts',(13.7373569299619,-3.59512579987478,11.9964200114457));
#12946=CARTESIAN_POINT('Ctrl Pts',(13.4761347388995,-3.44665140507887,11.791676091236));
#12947=CARTESIAN_POINT('Ctrl Pts',(13.2939612159655,-3.34310697244292,11.6488899018536));
#12948=CARTESIAN_POINT('Ctrl Pts',(13.1125197030785,-3.23979551676186,11.5062843729564));
#12949=CARTESIAN_POINT('Ctrl Pts',(12.9320810503802,-3.13688485529761,11.3640491305165));
#12950=CARTESIAN_POINT('Ctrl Pts',(12.7419408532674,-3.02844105368856,11.2141664051166));
#12951=CARTESIAN_POINT('Ctrl Pts',(12.5505198976557,-2.91909407414947,11.0628597070358));
#12952=CARTESIAN_POINT('Ctrl Pts',(12.3584607150064,-2.80917609774746,10.9104517039517));
#12953=CARTESIAN_POINT('Ctrl Pts',(12.1609503726549,-2.69613835151589,10.7537179490171));
#12954=CARTESIAN_POINT('Ctrl Pts',(11.9627650599007,-2.5824969662107,10.5958192942301));
#12955=CARTESIAN_POINT('Ctrl Pts',(11.764603586073,-2.46864604141743,10.4371523366741));
#12956=CARTESIAN_POINT('Ctrl Pts',(11.5611715157472,-2.35176696854911,10.2742652373585));
#12957=CARTESIAN_POINT('Ctrl Pts',(11.357764569323,-2.23466749726805,10.1105684093218));
#12958=CARTESIAN_POINT('Ctrl Pts',(11.1551388120544,-2.1178029693577,9.94654008829807));
#12959=CARTESIAN_POINT('Ctrl Pts',(10.9369442531874,-1.99195912572037,9.76990860950719));
#12960=CARTESIAN_POINT('Ctrl Pts',(10.7196555410832,-1.86638826421775,9.59289262515015));
#12961=CARTESIAN_POINT('Ctrl Pts',(10.5042167520004,-1.74168466284082,9.41614744679526));
#12962=CARTESIAN_POINT('Ctrl Pts',(10.3518588411099,-1.65349450791466,9.29115358543552));
#12963=CARTESIAN_POINT('Ctrl Pts',(10.2004261307567,-1.5657386876737,9.16629650496035));
#12964=CARTESIAN_POINT('Ctrl Pts',(10.0502525316942,-1.47863151154858,9.041822881172));
#12965=CARTESIAN_POINT('Ctrl Pts',(15.8,-4.75758878307678,13.5950405390087));
#12966=CARTESIAN_POINT('Ctrl Pts',(15.8,-4.76123078081695,13.6029203421718));
#12967=CARTESIAN_POINT('Ctrl Pts',(15.8,-4.76483261634472,13.610814146196));
#12968=CARTESIAN_POINT('Ctrl Pts',(15.8,-4.7683942897085,13.6187219510797));
#12969=CARTESIAN_POINT('Ctrl Pts',(15.8,-4.77191579174908,13.626643760007));
#12970=CARTESIAN_POINT('Ctrl Pts',(15.8,-4.77539710335946,13.6345795785203));
#12971=CARTESIAN_POINT('Ctrl Pts',(10.0502525316942,1.38781479615277,9.05620683581208));
#12972=CARTESIAN_POINT('Ctrl Pts',(11.9668350211294,0.817330781359223,10.8374137839212));
#12973=CARTESIAN_POINT('Ctrl Pts',(13.8834175105647,0.246846766565676,12.6186207320303));
#12974=CARTESIAN_POINT('Ctrl Pts',(15.8,-0.323637248227871,14.3998276801393));
#12975=CARTESIAN_POINT('Ctrl Pts',(10.0502525316942,1.39655842853148,9.21244502400635));
#12976=CARTESIAN_POINT('Ctrl Pts',(11.9668350211294,0.813302761662287,11.0233696506194));
#12977=CARTESIAN_POINT('Ctrl Pts',(13.8834175105647,0.230291956370553,12.8346197703481));
#12978=CARTESIAN_POINT('Ctrl Pts',(15.8,-0.352963710498644,14.6455443969611));
#12979=CARTESIAN_POINT('Ctrl Pts',(10.0502525316942,1.46541714813613,9.51829373400972));
#12980=CARTESIAN_POINT('Ctrl Pts',(11.9668350211295,0.867231464171969,11.3925515672309));
#12981=CARTESIAN_POINT('Ctrl Pts',(13.8834175105647,0.269566015193983,13.2668740653713));
#12982=CARTESIAN_POINT('Ctrl Pts',(15.8,-0.328619668770181,15.1411318985925));
#12983=CARTESIAN_POINT('Ctrl Pts',(10.0502525316941,1.79039750449509,10.0083300006651));
#12984=CARTESIAN_POINT('Ctrl Pts',(11.9668350211294,1.20809631886684,12.0019243797287));
#12985=CARTESIAN_POINT('Ctrl Pts',(13.8834175105647,0.625444427693873,13.9956114385883));
#12986=CARTESIAN_POINT('Ctrl Pts',(15.7999999999999,0.043143242065623,15.9892058176518));
#12987=CARTESIAN_POINT('Ctrl Pts',(10.0502525316942,2.10732113862255,10.3276659549724));
#12988=CARTESIAN_POINT('Ctrl Pts',(11.9668350211294,1.55295659524519,12.4074689224609));
#12989=CARTESIAN_POINT('Ctrl Pts',(13.8834175105647,0.999648742962748,14.4874157824202));
#12990=CARTESIAN_POINT('Ctrl Pts',(15.8,0.445284199585382,16.5672187499087));
#12991=CARTESIAN_POINT('Ctrl Pts',(10.0502525316942,2.32206279789789,10.5073910450885));
#12992=CARTESIAN_POINT('Ctrl Pts',(11.9668350211294,1.79024801807933,12.6387996550358));
#12993=CARTESIAN_POINT('Ctrl Pts',(13.8834175105647,1.25843323826076,14.7702082649831));
#12994=CARTESIAN_POINT('Ctrl Pts',(15.8,0.7266184584422,16.9016168749304));
#12995=CARTESIAN_POINT('',(10.0502525316942,2.32206279789789,10.5073910450885));
#12996=CARTESIAN_POINT('',(15.8,-0.323637248227871,14.3998276801393));
#12997=CARTESIAN_POINT('Ctrl Pts',(15.8,-0.323637248227871,14.3998276801393));
#12998=CARTESIAN_POINT('Ctrl Pts',(15.5456570571827,-0.248663394075326,
14.1695921802541));
#12999=CARTESIAN_POINT('Ctrl Pts',(15.290525950772,-0.173284602939826,13.9381981568641));
#13000=CARTESIAN_POINT('Ctrl Pts',(15.0353275664542,-0.0977165877046862,
13.7061319160856));
#13001=CARTESIAN_POINT('Ctrl Pts',(14.7778789011685,-0.0214822309998696,
13.4720193682887));
#13002=CARTESIAN_POINT('Ctrl Pts',(14.5203617662622,0.0549444640636946,
13.23722264667));
#13003=CARTESIAN_POINT('Ctrl Pts',(14.2635162858845,0.131318796804616,13.0022894235191));
#13004=CARTESIAN_POINT('Ctrl Pts',(14.0000820510512,0.209652329779073,12.7613295522896));
#13005=CARTESIAN_POINT('Ctrl Pts',(13.737354372103,0.287930509546182,12.5202260255198));
#13006=CARTESIAN_POINT('Ctrl Pts',(13.4761318051391,0.365868800886513,12.2796215208081));
#13007=CARTESIAN_POINT('Ctrl Pts',(13.2939592679841,0.420221747647607,12.1118276981546));
#13008=CARTESIAN_POINT('Ctrl Pts',(13.1125187344712,0.474408950394415,11.9442776868956));
#13009=CARTESIAN_POINT('Ctrl Pts',(12.9320810503802,0.528329405335826,11.7772036867065));
#13010=CARTESIAN_POINT('Ctrl Pts',(12.7419408368634,0.58514928122335,11.6011457516411));
#13011=CARTESIAN_POINT('Ctrl Pts',(12.5505198646266,0.642388101081342,11.4234544410913));
#13012=CARTESIAN_POINT('Ctrl Pts',(12.3584606652976,0.69982965272817,11.2445392798291));
#13013=CARTESIAN_POINT('Ctrl Pts',(12.1609507027355,0.758901432444593,11.0605463915626));
#13014=CARTESIAN_POINT('Ctrl Pts',(11.9627657724259,0.818187336020824,10.8752590885166));
#13015=CARTESIAN_POINT('Ctrl Pts',(11.7646046796656,0.877435109078001,10.6891763370127));
#13016=CARTESIAN_POINT('Ctrl Pts',(11.5611733354004,0.938258623673378,10.498144567074));
#13017=CARTESIAN_POINT('Ctrl Pts',(11.3577671135027,0.999041534288953,10.3062745975178));
#13018=CARTESIAN_POINT('Ctrl Pts',(11.1551420711301,1.05949856916745,10.1141619588682));
#13019=CARTESIAN_POINT('Ctrl Pts',(10.9369470578872,1.12460120096202,9.90728713607513));
#13020=CARTESIAN_POINT('Ctrl Pts',(10.7196578904047,1.18932539513682,9.70013097729772));
#13021=CARTESIAN_POINT('Ctrl Pts',(10.5042186507217,1.25330845309555,9.49350036754161));
#13022=CARTESIAN_POINT('Ctrl Pts',(10.3518600992373,1.29855724827547,9.34737127591884));
#13023=CARTESIAN_POINT('Ctrl Pts',(10.20042675459,1.3434352294294,9.20150648816153));
#13024=CARTESIAN_POINT('Ctrl Pts',(10.0502525316942,1.38781479615277,9.05620683581208));
#13025=CARTESIAN_POINT('Ctrl Pts',(15.8,-0.323637248227871,14.3998276801393));
#13026=CARTESIAN_POINT('Ctrl Pts',(15.8,-0.324666000821258,14.4084472574799));
#13027=CARTESIAN_POINT('Ctrl Pts',(15.8,-0.325652230376828,14.4170677396245));
#13028=CARTESIAN_POINT('Ctrl Pts',(15.8,-0.326595936941117,14.4256891265865));
#13029=CARTESIAN_POINT('Ctrl Pts',(15.8,-0.327497110819209,14.434311418564));
#13030=CARTESIAN_POINT('Ctrl Pts',(15.8,-0.328355732126619,14.4429346149236));
#13031=CARTESIAN_POINT('Ctrl Pts',(10.0502525316942,4.11841212213242,8.18410616705958));
#13032=CARTESIAN_POINT('Ctrl Pts',(11.9668350211294,4.12627279988524,10.0544238975194));
#13033=CARTESIAN_POINT('Ctrl Pts',(13.8834175105647,4.13413347763806,11.9247416279792));
#13034=CARTESIAN_POINT('Ctrl Pts',(15.8,4.14199415539088,13.795059358439));
#13035=CARTESIAN_POINT('Ctrl Pts',(10.0502525316942,4.17500806600467,8.3299955830383));
#13036=CARTESIAN_POINT('Ctrl Pts',(11.9668350211294,4.17990544851818,10.2325231628261));
#13037=CARTESIAN_POINT('Ctrl Pts',(13.8834175105647,4.18513629113481,12.1352846385738));
#13038=CARTESIAN_POINT('Ctrl Pts',(15.8,4.19003367364832,14.0378122183616));
#13039=CARTESIAN_POINT('Ctrl Pts',(10.0502525316942,4.3350236730215,8.59959242261694));
#13040=CARTESIAN_POINT('Ctrl Pts',(11.9668350211295,4.34529280263861,10.5669670902559));
#13041=CARTESIAN_POINT('Ctrl Pts',(13.8834175105647,4.35608887336509,12.5342444956751));
#13042=CARTESIAN_POINT('Ctrl Pts',(15.8,4.36635800298219,14.501619163314));
#13043=CARTESIAN_POINT('Ctrl Pts',(10.0502525316941,4.79552866926089,8.96521881277978));
#13044=CARTESIAN_POINT('Ctrl Pts',(11.9668350211294,4.85778187524376,11.0411807000414));
#13045=CARTESIAN_POINT('Ctrl Pts',(13.8834175105647,4.91974349130654,13.1173407686982));
#13046=CARTESIAN_POINT('Ctrl Pts',(15.8,4.98199669728941,15.1933026559598));
#13047=CARTESIAN_POINT('Ctrl Pts',(10.0502525316942,5.19560579312754,9.17099596015618));
#13048=CARTESIAN_POINT('Ctrl Pts',(11.9668350211294,5.3110682436509,11.3203141899786));
#13049=CARTESIAN_POINT('Ctrl Pts',(13.8834175105647,5.42758013234466,13.4694427341669));
#13050=CARTESIAN_POINT('Ctrl Pts',(15.8,5.54304258286802,15.6187609639894));
#13051=CARTESIAN_POINT('Ctrl Pts',(10.0502525316942,5.45537535466284,9.2755658561365));
#13052=CARTESIAN_POINT('Ctrl Pts',(11.9668350211294,5.60823092528512,11.4669957083382));
#13053=CARTESIAN_POINT('Ctrl Pts',(13.8834175105647,5.76108649590741,13.6584255605399));
#13054=CARTESIAN_POINT('Ctrl Pts',(15.8,5.91394206652969,15.8498554127416));
#13055=CARTESIAN_POINT('',(10.0502525316942,5.45537535466284,9.2755658561365));
#13056=CARTESIAN_POINT('',(15.8,4.14199415539088,13.795059358439));
#13057=CARTESIAN_POINT('Ctrl Pts',(15.8,4.14199415539088,13.795059358439));
#13058=CARTESIAN_POINT('Ctrl Pts',(15.5456574794166,4.14215184549968,13.5529245928915));
#13059=CARTESIAN_POINT('Ctrl Pts',(15.2905267978567,4.14233665870497,13.3095628770614));
#13060=CARTESIAN_POINT('Ctrl Pts',(15.0353288374163,4.14249371366664,13.0655033718489));
#13061=CARTESIAN_POINT('Ctrl Pts',(14.7778805061933,4.1426521535606,12.8192917162869));
#13062=CARTESIAN_POINT('Ctrl Pts',(14.5203637043094,4.14278210218064,12.5723699372128));
#13063=CARTESIAN_POINT('Ctrl Pts',(14.2635185530345,4.14282007025482,12.3253345162688));
#13064=CARTESIAN_POINT('Ctrl Pts',(14.0000848089498,4.14285901228618,12.0719621417552));
#13065=CARTESIAN_POINT('Ctrl Pts',(13.7373576158051,4.14280091850188,11.8184702457645));
#13066=CARTESIAN_POINT('Ctrl Pts',(13.4761355251999,4.14257377376941,11.5655579735746));
#13067=CARTESIAN_POINT('Ctrl Pts',(13.2939617380594,4.14241536520585,11.3891793743052));
#13068=CARTESIAN_POINT('Ctrl Pts',(13.1125199626826,4.14217466317552,11.2130838733096));
#13069=CARTESIAN_POINT('Ctrl Pts',(12.9320810503802,4.14182735974364,11.0375235228707));
#13070=CARTESIAN_POINT('Ctrl Pts',(12.7419408575531,4.14146138357661,10.85252418731));
#13071=CARTESIAN_POINT('Ctrl Pts',(12.5505199062848,4.14098910290385,10.6658419590994));
#13072=CARTESIAN_POINT('Ctrl Pts',(12.3584607279933,4.14033143664814,10.4779331330941));
#13073=CARTESIAN_POINT('Ctrl Pts',(12.160950283566,4.13965510367824,10.2846908414929));
#13074=CARTESIAN_POINT('Ctrl Pts',(11.962764868023,4.13878241284077,10.0901513147869));
#13075=CARTESIAN_POINT('Ctrl Pts',(11.7646032917771,4.13762764472382,9.89486705365981));
#13076=CARTESIAN_POINT('Ctrl Pts',(11.5611710263546,4.13644216215692,9.69438863400336));
#13077=CARTESIAN_POINT('Ctrl Pts',(11.3577638852466,4.13495903745939,9.49312558221559));
#13078=CARTESIAN_POINT('Ctrl Pts',(11.1551379358825,4.1330909916179,9.29173244420265));
#13079=CARTESIAN_POINT('Ctrl Pts',(10.9369434970461,4.13107941701264,9.07486553810229));
#13080=CARTESIAN_POINT('Ctrl Pts',(10.7196549052597,4.12862098831913,8.85784801697389));
#13081=CARTESIAN_POINT('Ctrl Pts',(10.5042162352553,4.12562010893634,8.6415593449323));
#13082=CARTESIAN_POINT('Ctrl Pts',(10.3518584987051,4.12349789387433,8.48860048887813));
#13083=CARTESIAN_POINT('Ctrl Pts',(10.2004259609778,4.12110469363329,8.33600758581849));
#13084=CARTESIAN_POINT('Ctrl Pts',(10.0502525316942,4.11841212213242,8.18410616705958));
#13085=CARTESIAN_POINT('Ctrl Pts',(15.8,4.14199415539088,13.795059358439));
#13086=CARTESIAN_POINT('Ctrl Pts',(15.8,4.14367934941586,13.8035749656708));
#13087=CARTESIAN_POINT('Ctrl Pts',(15.8,4.14540526485285,13.8120782930811));
#13088=CARTESIAN_POINT('Ctrl Pts',(15.8,4.14717190166176,13.8205693406969));
#13089=CARTESIAN_POINT('Ctrl Pts',(15.8,4.14897926912419,13.8290481057107));
#13090=CARTESIAN_POINT('Ctrl Pts',(15.8,4.15082738595568,13.8375145813754));
#13091=CARTESIAN_POINT('Ctrl Pts',(10.0502525316942,6.44587057493322,6.51088816465466));
#13092=CARTESIAN_POINT('Ctrl Pts',(11.9668350211294,7.03130648732539,8.28723694673789));
#13093=CARTESIAN_POINT('Ctrl Pts',(13.8834175105647,7.61674239971757,10.0635857288211));
#13094=CARTESIAN_POINT('Ctrl Pts',(15.8,8.20217831210975,11.8399345109044));
#13095=CARTESIAN_POINT('Ctrl Pts',(10.0502525316942,6.54477882498566,6.6321481359105));
#13096=CARTESIAN_POINT('Ctrl Pts',(11.9668350211294,7.13734986695938,8.44004601367429));
#13097=CARTESIAN_POINT('Ctrl Pts',(13.8834175105647,7.73031032616364,10.2480632948761));
#13098=CARTESIAN_POINT('Ctrl Pts',(15.8,8.32288136813736,12.0559611726399));
#13099=CARTESIAN_POINT('Ctrl Pts',(10.0502525316942,6.78027814405439,6.83909882511009));
#13100=CARTESIAN_POINT('Ctrl Pts',(11.9668350211295,7.39799687329661,8.70700998719296));
#13101=CARTESIAN_POINT('Ctrl Pts',(13.8834175105647,8.01619193743947,10.5746650104356));
#13102=CARTESIAN_POINT('Ctrl Pts',(15.8,8.63391066668169,12.4425761725185));
#13103=CARTESIAN_POINT('Ctrl Pts',(10.0502525316941,7.33122941665113,7.04452561799896));
#13104=CARTESIAN_POINT('Ctrl Pts',(11.9668350211294,8.03194323669993,8.99964539985647));
#13105=CARTESIAN_POINT('Ctrl Pts',(13.8834175105647,8.73244671395173,10.9550426722922));
#13106=CARTESIAN_POINT('Ctrl Pts',(15.8,9.43316053400053,12.9101624541498));
#13107=CARTESIAN_POINT('Ctrl Pts',(10.0502525316942,7.77530835268703,7.11660498267373));
#13108=CARTESIAN_POINT('Ctrl Pts',(11.9668350211294,8.54929552797968,9.12504823131443));
#13109=CARTESIAN_POINT('Ctrl Pts',(13.8834175105647,9.32422216219826,11.1329867839676));
#13110=CARTESIAN_POINT('Ctrl Pts',(15.8,10.0982093374909,13.1414300326083));
#13111=CARTESIAN_POINT('Ctrl Pts',(10.0502525316942,8.05467776187827,7.13578365451838));
#13112=CARTESIAN_POINT('Ctrl Pts',(11.9668350211294,8.8772411146815,9.17272232645135));
#13113=CARTESIAN_POINT('Ctrl Pts',(13.8834175105647,9.69980446748474,11.2096609983843));
#13114=CARTESIAN_POINT('Ctrl Pts',(15.8,10.522367820288,13.2465996703173));
#13115=CARTESIAN_POINT('',(10.0502525316942,8.05467776187827,7.13578365451838));
#13116=CARTESIAN_POINT('',(15.8,8.20217831210975,11.8399345109044));
#13117=CARTESIAN_POINT('Ctrl Pts',(15.8,8.20217831210975,11.8399345109044));
#13118=CARTESIAN_POINT('Ctrl Pts',(15.5456576615066,8.1275045802929,11.6096021002861));
#13119=CARTESIAN_POINT('Ctrl Pts',(15.2905271631652,8.05247749955186,11.3780944093847));
#13120=CARTESIAN_POINT('Ctrl Pts',(15.0353293855237,7.97720839274424,11.1459316587091));
#13121=CARTESIAN_POINT('Ctrl Pts',(14.7778811978186,7.90127554051927,10.9117216277032));
#13122=CARTESIAN_POINT('Ctrl Pts',(14.5203645390038,7.82509615349623,10.6768450327852));
#13123=CARTESIAN_POINT('Ctrl Pts',(14.263519529112,7.74879417034726,10.441888780704));
#13124=CARTESIAN_POINT('Ctrl Pts',(14.0000859949182,7.67053490770714,10.2009054892912));
#13125=CARTESIAN_POINT('Ctrl Pts',(13.7373590095431,7.5921464241734,9.959838511058));
#13126=CARTESIAN_POINT('Ctrl Pts',(13.4761371226612,7.51377627479485,9.71937502566857));
#13127=CARTESIAN_POINT('Ctrl Pts',(13.2939627987543,7.45912147864456,9.55167746633298));
#13128=CARTESIAN_POINT('Ctrl Pts',(13.1125204900987,7.40447589782765,9.38427458086216));
#13129=CARTESIAN_POINT('Ctrl Pts',(12.9320810503802,7.3498943027601,9.21741359915303));
#13130=CARTESIAN_POINT('Ctrl Pts',(12.7419408661186,7.29237830426429,9.04158187490393));
#13131=CARTESIAN_POINT('Ctrl Pts',(12.5505199235311,7.23424116054677,8.86418247516826));
#13132=CARTESIAN_POINT('Ctrl Pts',(12.3584607539489,7.17554866346938,8.68567379986745));
#13133=CARTESIAN_POINT('Ctrl Pts',(12.1609501017825,7.11519021560016,8.5020982645117));
#13134=CARTESIAN_POINT('Ctrl Pts',(11.9627644770495,7.05424414957912,8.31734966162925));
#13135=CARTESIAN_POINT('Ctrl Pts',(11.7646026923682,6.99279967398829,8.13197994128733));
#13136=CARTESIAN_POINT('Ctrl Pts',(11.5611700299535,6.92972084534216,7.94167959755111));
#13137=CARTESIAN_POINT('Ctrl Pts',(11.3577624926938,6.86611647390408,7.75072500005124));
#13138=CARTESIAN_POINT('Ctrl Pts',(11.1551361524456,6.80210582000319,7.55976563308471));
#13139=CARTESIAN_POINT('Ctrl Pts',(10.9369419552409,6.73317720379591,7.35413478705085));
#13140=CARTESIAN_POINT('Ctrl Pts',(10.7196536056931,6.66377706212401,7.14849878641298));
#13141=CARTESIAN_POINT('Ctrl Pts',(10.5042151754617,6.59408624907902,6.94372358733632));
#13142=CARTESIAN_POINT('Ctrl Pts',(10.3518577964665,6.54480112569514,6.79890721181295));
#13143=CARTESIAN_POINT('Ctrl Pts',(10.2004256127779,6.49537136769551,6.65452261540843));
#13144=CARTESIAN_POINT('Ctrl Pts',(10.0502525316942,6.44587057493322,6.51088816465466));
#13145=CARTESIAN_POINT('Ctrl Pts',(15.8,8.20217831210975,11.8399345109044));
#13146=CARTESIAN_POINT('Ctrl Pts',(15.8,8.20641249422049,11.8475125810599));
#13147=CARTESIAN_POINT('Ctrl Pts',(15.8,8.21068161002192,11.8550663888027));
#13148=CARTESIAN_POINT('Ctrl Pts',(15.8,8.21498565948429,11.862595934171));
#13149=CARTESIAN_POINT('Ctrl Pts',(15.8,8.21932465056733,11.8701012116266));
#13150=CARTESIAN_POINT('Ctrl Pts',(15.8,8.22369859898568,11.8775822089691));
#13151=CARTESIAN_POINT('Ctrl Pts',(10.0502525316942,8.14236230483842,4.20033906466803));
#13152=CARTESIAN_POINT('Ctrl Pts',(11.9668350211294,9.24806690579316,5.70883750303466));
#13153=CARTESIAN_POINT('Ctrl Pts',(13.8834175105647,10.3537715067479,7.2173359414013));
#13154=CARTESIAN_POINT('Ctrl Pts',(15.8,11.4594761077026,8.72583437976793));
#13155=CARTESIAN_POINT('Ctrl Pts',(10.0502525316942,8.27390103242162,4.28509982034658));
#13156=CARTESIAN_POINT('Ctrl Pts',(11.9668350211294,9.39614075158195,5.82139835544565));
#13157=CARTESIAN_POINT('Ctrl Pts',(13.8834175105647,10.5187877262285,7.35769011342039));
#13158=CARTESIAN_POINT('Ctrl Pts',(15.8,11.6410274453888,8.89398864851946));
#13159=CARTESIAN_POINT('Ctrl Pts',(10.0502525316942,8.56182484570054,4.40914912230233));
#13160=CARTESIAN_POINT('Ctrl Pts',(11.9668350211295,9.72652656145018,5.99475261978217));
#13161=CARTESIAN_POINT('Ctrl Pts',(13.8834175105647,10.8916014121612,7.57996568930602));
#13162=CARTESIAN_POINT('Ctrl Pts',(15.8,12.0563031279108,9.16556918678585));
#13163=CARTESIAN_POINT('Ctrl Pts',(10.0502525316941,9.14929101108338,4.43426842278356));
#13164=CARTESIAN_POINT('Ctrl Pts',(11.9668350211294,10.4198746943315,6.07716535286823));
#13165=CARTESIAN_POINT('Ctrl Pts',(13.8834175105647,11.6903432820694,7.72039163021277));
#13166=CARTESIAN_POINT('Ctrl Pts',(15.8,12.9609269653175,9.36328856029745));
#13167=CARTESIAN_POINT('Ctrl Pts',(10.0502525316942,9.59390955692677,4.36559112518463));
#13168=CARTESIAN_POINT('Ctrl Pts',(11.9668350211294,10.9506581995853,6.03655897381968));
#13169=CARTESIAN_POINT('Ctrl Pts',(13.8834175105647,12.30814436114,7.70675651927344));
#13170=CARTESIAN_POINT('Ctrl Pts',(15.8,13.6648930037986,9.37772436790849));
#13171=CARTESIAN_POINT('Ctrl Pts',(10.0502525316942,9.86553218952113,4.2975012308678));
#13172=CARTESIAN_POINT('Ctrl Pts',(11.9668350211294,11.2772850923971,5.98055897313701));
#13173=CARTESIAN_POINT('Ctrl Pts',(13.8834175105647,12.689037995273,7.66361671540623));
#13174=CARTESIAN_POINT('Ctrl Pts',(15.8,14.1007908981489,9.34667445767544));
#13175=CARTESIAN_POINT('',(10.0502525316942,9.86553218952113,4.2975012308678));
#13176=CARTESIAN_POINT('',(15.8,11.4594761077026,8.72583437976793));
#13177=CARTESIAN_POINT('Ctrl Pts',(15.8,11.4594761077026,8.72583437976793));
#13178=CARTESIAN_POINT('Ctrl Pts',(15.5456576332005,11.3172805234006,8.52985067008894));
#13179=CARTESIAN_POINT('Ctrl Pts',(15.2905271063775,11.1743857021219,8.33285839341008));
#13180=CARTESIAN_POINT('Ctrl Pts',(15.0353293003195,11.0310582754423,8.13531790820529));
#13181=CARTESIAN_POINT('Ctrl Pts',(14.7778810903258,10.8864669483786,7.93603545706342));
#13182=CARTESIAN_POINT('Ctrl Pts',(14.520364409292,10.7414351729093,7.73619524960918));
#13183=CARTESIAN_POINT('Ctrl Pts',(14.2635193774432,10.596262186244,7.53631716809864));
#13184=CARTESIAN_POINT('Ctrl Pts',(14.0000858106889,10.4473652525624,7.3313118559487));
#13185=CARTESIAN_POINT('Ctrl Pts',(13.7373587930825,10.2983195619262,7.12626688447295));
#13186=CARTESIAN_POINT('Ctrl Pts',(13.4761368745974,10.1494777980979,6.92179020337647));
#13187=CARTESIAN_POINT('Ctrl Pts',(13.2939626340429,10.045676649077,6.77918967312285));
#13188=CARTESIAN_POINT('Ctrl Pts',(13.1125204081982,9.94197532369066,6.63686654642478));
#13189=CARTESIAN_POINT('Ctrl Pts',(12.9320810503802,9.83850230979699,6.49503902755748));
#13190=CARTESIAN_POINT('Ctrl Pts',(12.7419408648006,9.72946635277444,6.34558654067312));
#13191=CARTESIAN_POINT('Ctrl Pts',(12.5505199208775,9.6193552133211,6.19483505008001));
#13192=CARTESIAN_POINT('Ctrl Pts',(12.3584607499552,9.50837311662931,6.04320018913779));
#13193=CARTESIAN_POINT('Ctrl Pts',(12.1609501300795,9.39424088015531,5.88726129158008));
#13194=CARTESIAN_POINT('Ctrl Pts',(11.9627645378627,9.27918728832936,5.73038832458522));
#13195=CARTESIAN_POINT('Ctrl Pts',(11.7646027855802,9.16346774534062,5.57307865663058));
#13196=CARTESIAN_POINT('Ctrl Pts',(11.5611701848685,9.04467021094143,5.4115847532889));
#13197=CARTESIAN_POINT('Ctrl Pts',(11.3577627091811,8.92517068068721,5.2496310192305));
#13198=CARTESIAN_POINT('Ctrl Pts',(11.1551364296864,8.80528327914564,5.087798296836));
#13199=CARTESIAN_POINT('Ctrl Pts',(10.9369421951531,8.67618482323568,4.91353182422764));
#13200=CARTESIAN_POINT('Ctrl Pts',(10.7196538081805,8.5466363268491,4.73940615822481));
#13201=CARTESIAN_POINT('Ctrl Pts',(10.5042153409026,8.41707738748313,4.5661889859333));
#13202=CARTESIAN_POINT('Ctrl Pts',(10.3518579060906,8.32545369600329,4.44369032369729));
#13203=CARTESIAN_POINT('Ctrl Pts',(10.2004256671343,8.23382587572336,4.32164700273164));
#13204=CARTESIAN_POINT('Ctrl Pts',(10.0502525316942,8.14236230483842,4.20033906466803));
#13205=CARTESIAN_POINT('Ctrl Pts',(15.8,11.4594761077026,8.72583437976793));
#13206=CARTESIAN_POINT('Ctrl Pts',(15.8,11.4658448066529,8.73173311854078));
#13207=CARTESIAN_POINT('Ctrl Pts',(15.8,11.4722392320194,8.73759798728384));
#13208=CARTESIAN_POINT('Ctrl Pts',(15.8,11.4786593837858,8.74342898604263));
#13209=CARTESIAN_POINT('Ctrl Pts',(15.8,11.4851052678107,8.74922610709021));
#13210=CARTESIAN_POINT('Ctrl Pts',(15.8,11.4915768952696,8.7549893339674));
#13211=CARTESIAN_POINT('Ctrl Pts',(10.0502525316942,9.041822881172,1.47863151154858));
#13212=CARTESIAN_POINT('Ctrl Pts',(11.9668350211294,10.5595621004509,2.57161726872465));
#13213=CARTESIAN_POINT('Ctrl Pts',(13.8834175105647,12.0773013197298,3.66460302590071));
#13214=CARTESIAN_POINT('Ctrl Pts',(15.8,13.5950405390087,4.75758878307678));
#13215=CARTESIAN_POINT('Ctrl Pts',(10.0502525316942,9.19311615914592,1.5185960783211));
#13216=CARTESIAN_POINT('Ctrl Pts',(11.9668350211294,10.7351719126775,2.63291166611866));
#13217=CARTESIAN_POINT('Ctrl Pts',(13.8834175105647,12.2776128949465,3.74709495962168));
#13218=CARTESIAN_POINT('Ctrl Pts',(15.8,13.8196686484781,4.86141054741924));
#13219=CARTESIAN_POINT('Ctrl Pts',(10.0502525316942,9.50527827631687,1.54760878347554));
#13220=CARTESIAN_POINT('Ctrl Pts',(11.9668350211295,11.1029538596823,2.69569469846983));
#13221=CARTESIAN_POINT('Ctrl Pts',(13.8834175105647,12.7008586295609,3.84329897549064));
#13222=CARTESIAN_POINT('Ctrl Pts',(15.8,14.2985342129264,4.99138489048493));
#13223=CARTESIAN_POINT('Ctrl Pts',(10.0502525316941,10.0717544060046,1.38996253959751));
#13224=CARTESIAN_POINT('Ctrl Pts',(11.9668350211294,11.7878343688586,2.55981841965666));
#13225=CARTESIAN_POINT('Ctrl Pts',(13.8834175105647,13.5039013178589,3.73002877331941));
#13226=CARTESIAN_POINT('Ctrl Pts',(15.8,15.2199812807128,4.89988465337857));
#13227=CARTESIAN_POINT('Ctrl Pts',(10.0502525316942,10.473392049036,1.18724279150055));
#13228=CARTESIAN_POINT('Ctrl Pts',(11.9668350211294,12.2800941488934,2.35716926478797));
#13229=CARTESIAN_POINT('Ctrl Pts',(13.8834175105647,14.0872596341291,3.52613523034269));
#13230=CARTESIAN_POINT('Ctrl Pts',(15.8,15.8939617339865,4.69606170363011));
#13231=CARTESIAN_POINT('Ctrl Pts',(10.0502525316942,10.7106795892491,1.03854944428815));
#13232=CARTESIAN_POINT('Ctrl Pts',(11.9668350211294,12.5734298318033,2.20297683852746));
#13233=CARTESIAN_POINT('Ctrl Pts',(13.8834175105647,14.4361800743576,3.36740423276678));
#13234=CARTESIAN_POINT('Ctrl Pts',(15.8,16.2989303169119,4.5318316270061));
#13235=CARTESIAN_POINT('',(10.0502525316942,10.7106795892491,1.03854944428815));
#13236=CARTESIAN_POINT('',(15.8,13.5950405390087,4.75758878307678));
#13237=CARTESIAN_POINT('Ctrl Pts',(15.8,13.5950405390087,4.75758878307678));
#13238=CARTESIAN_POINT('Ctrl Pts',(15.5456573899564,13.3992420178037,4.61513791473842));
#13239=CARTESIAN_POINT('Ctrl Pts',(15.2905266183818,13.202466813866,4.47194392111128));
#13240=CARTESIAN_POINT('Ctrl Pts',(15.0353285681331,13.0051107697467,4.32836223491354));
#13241=CARTESIAN_POINT('Ctrl Pts',(14.7778801662818,12.806014428279,4.18351443685758));
#13242=CARTESIAN_POINT('Ctrl Pts',(14.5203632939903,12.6063268373515,4.03827228949007));
#13243=CARTESIAN_POINT('Ctrl Pts',(14.2635180731369,12.4064932437275,3.8930377592338));
#13244=CARTESIAN_POINT('Ctrl Pts',(14.000084225555,12.2015334929891,3.74407765407776));
#13245=CARTESIAN_POINT('Ctrl Pts',(13.7373569299579,11.9964200114426,3.59512579987254));
#13246=CARTESIAN_POINT('Ctrl Pts',(13.476134738894,11.7916760912317,3.44665140507575));
#13247=CARTESIAN_POINT('Ctrl Pts',(13.2939612159618,11.6488899018507,3.34310697244085));
#13248=CARTESIAN_POINT('Ctrl Pts',(13.1125197030766,11.5062843729549,3.23979551676083));
#13249=CARTESIAN_POINT('Ctrl Pts',(12.9320810503802,11.3640491305165,3.13688485529761));
#13250=CARTESIAN_POINT('Ctrl Pts',(12.7419408532675,11.2141664051166,3.02844105368859));
#13251=CARTESIAN_POINT('Ctrl Pts',(12.5505198976558,11.0628597070359,2.91909407414952));
#13252=CARTESIAN_POINT('Ctrl Pts',(12.3584607150066,10.9104517039518,2.80917609774754));
#13253=CARTESIAN_POINT('Ctrl Pts',(12.160950372655,10.7537179490173,2.696138351516));
#13254=CARTESIAN_POINT('Ctrl Pts',(11.9627650599009,10.5958192942303,2.58249696621083));
#13255=CARTESIAN_POINT('Ctrl Pts',(11.7646035860733,10.4371523366744,2.46864604141759));
#13256=CARTESIAN_POINT('Ctrl Pts',(11.5611715157476,10.2742652373588,2.35176696854934));
#13257=CARTESIAN_POINT('Ctrl Pts',(11.3577645693235,10.1105684093222,2.23466749726835));
#13258=CARTESIAN_POINT('Ctrl Pts',(11.155138812055,9.94654008829857,2.11780296935806));
#13259=CARTESIAN_POINT('Ctrl Pts',(10.9369442531883,9.76990860950791,1.99195912572088));
#13260=CARTESIAN_POINT('Ctrl Pts',(10.7196555410844,9.59289262515108,1.86638826421842));
#13261=CARTESIAN_POINT('Ctrl Pts',(10.5042167520018,9.41614744679641,1.74168466284163));
#13262=CARTESIAN_POINT('Ctrl Pts',(10.3518588411108,9.29115358543629,1.6534945079152));
#13263=CARTESIAN_POINT('Ctrl Pts',(10.2004261307572,9.16629650496073,1.56573868767396));
#13264=CARTESIAN_POINT('Ctrl Pts',(10.0502525316942,9.041822881172,1.47863151154858));
#13265=CARTESIAN_POINT('Ctrl Pts',(15.8,13.5950405390087,4.75758878307678));
#13266=CARTESIAN_POINT('Ctrl Pts',(15.8,13.6029203421718,4.76123078081695));
#13267=CARTESIAN_POINT('Ctrl Pts',(15.8,13.610814146196,4.76483261634472));
#13268=CARTESIAN_POINT('Ctrl Pts',(15.8,13.6187219510797,4.76839428970851));
#13269=CARTESIAN_POINT('Ctrl Pts',(15.8,13.626643760007,4.77191579174908));
#13270=CARTESIAN_POINT('Ctrl Pts',(15.8,13.6345795785203,4.77539710335946));
#13271=CARTESIAN_POINT('Ctrl Pts',(10.0502525316942,10.5073910450885,-2.3220627978979));
#13272=CARTESIAN_POINT('Ctrl Pts',(11.1454425256572,11.7253388222013,-2.01816863800157));
#13273=CARTESIAN_POINT('Ctrl Pts',(12.3775312688656,13.0955300714531,-1.67628770811821));
#13274=CARTESIAN_POINT('Ctrl Pts',(13.7465187613193,14.617964792844,-1.29642000824781));
#13275=CARTESIAN_POINT('Ctrl Pts',(14.2941137583008,15.2269386814004,-1.14447292829965));
#13276=CARTESIAN_POINT('Ctrl Pts',(14.8417087552824,15.8359125699568,-0.992525848351485));
#13277=CARTESIAN_POINT('Ctrl Pts',(15.3208543776412,16.3687647224436,-0.859572153396845));
#13278=CARTESIAN_POINT('Ctrl Pts',(15.5946518761319,16.6732516667218,-0.783598613422764));
#13279=CARTESIAN_POINT('Ctrl Pts',(15.7315506253773,16.8254951388609,-0.745611843435724));
#13280=CARTESIAN_POINT('Ctrl Pts',(15.8,16.9016168749304,-0.726618458442204));
#13281=CARTESIAN_POINT('Ctrl Pts',(10.0502525316942,10.3973886408451,-2.57345271232945));
#13282=CARTESIAN_POINT('Ctrl Pts',(11.1454425256572,11.618687280661,-2.29815463811992));
#13283=CARTESIAN_POINT('Ctrl Pts',(12.3775312688656,12.9928273987101,-1.98887116228557));
#13284=CARTESIAN_POINT('Ctrl Pts',(13.7465187613193,14.519468077176,-1.64478997784958));
#13285=CARTESIAN_POINT('Ctrl Pts',(14.2941137583008,15.1301263986154,-1.50716238874916));
#13286=CARTESIAN_POINT('Ctrl Pts',(14.8417087552824,15.740805777741,-1.36958497392712));
#13287=CARTESIAN_POINT('Ctrl Pts',(15.3208543776412,16.2751437253593,-1.24918922664557));
#13288=CARTESIAN_POINT('Ctrl Pts',(15.5946518761319,16.5804716520035,-1.18037249165619));
#13289=CARTESIAN_POINT('Ctrl Pts',(15.7315506253773,16.7331376997671,-1.14596909077303));
#13290=CARTESIAN_POINT('Ctrl Pts',(15.8,16.8094688647556,-1.12876296113493));
#13291=CARTESIAN_POINT('Ctrl Pts',(10.0502525316942,10.189368118401,-2.93870070814821));
#13292=CARTESIAN_POINT('Ctrl Pts',(11.1454425256572,11.4106316171747,-2.70946206711306));
#13293=CARTESIAN_POINT('Ctrl Pts',(12.3775312688656,12.7843360022416,-2.45105312324518));
#13294=CARTESIAN_POINT('Ctrl Pts',(13.7465187613194,14.310894320163,-2.16445481731473));
#13295=CARTESIAN_POINT('Ctrl Pts',(14.2941137583009,14.9215151635443,-2.04980959621707));
#13296=CARTESIAN_POINT('Ctrl Pts',(14.8417087552824,15.5321104940175,-1.93510378473096));
#13297=CARTESIAN_POINT('Ctrl Pts',(15.3208543776412,16.0663892944466,-1.83475492870443));
#13298=CARTESIAN_POINT('Ctrl Pts',(15.594651876132,16.3717012113088,-1.77743586902584));
#13299=CARTESIAN_POINT('Ctrl Pts',(15.7315506253773,16.5243546442885,-1.7487703415134));
#13300=CARTESIAN_POINT('Ctrl Pts',(15.8,16.6006836129618,-1.7344429264487));
#13301=CARTESIAN_POINT('Ctrl Pts',(10.0502525316942,9.95881139224219,-3.05808383535426));
#13302=CARTESIAN_POINT('Ctrl Pts',(11.1454425256572,11.1626816238278,-2.85649631904975));
#13303=CARTESIAN_POINT('Ctrl Pts',(12.3775312688656,12.5171248305866,-2.62997738853438));
#13304=CARTESIAN_POINT('Ctrl Pts',(13.7465187613193,14.0219712727573,-2.37801889657081));
#13305=CARTESIAN_POINT('Ctrl Pts',(14.2941137583008,14.6239108703276,-2.27723855544496));
#13306=CARTESIAN_POINT('Ctrl Pts',(14.8417087552823,15.225860952321,-2.17648960137064));
#13307=CARTESIAN_POINT('Ctrl Pts',(15.3208543776412,15.7525640332375,-2.08832456454097));
#13308=CARTESIAN_POINT('Ctrl Pts',(15.5946518761319,16.0535332175881,-2.03793255455516));
#13309=CARTESIAN_POINT('Ctrl Pts',(15.7315506253773,16.2040188475872,-2.01273965647872));
#13310=CARTESIAN_POINT('Ctrl Pts',(15.8,16.2792607370613,-2.00014043670969));
#13311=CARTESIAN_POINT('Ctrl Pts',(10.0502525316942,9.78147886731912,-3.07559947603193));
#13312=CARTESIAN_POINT('Ctrl Pts',(11.1454425256572,10.9672359168267,-2.88676320881926));
#13313=CARTESIAN_POINT('Ctrl Pts',(12.3775312688656,12.3013551830101,-2.67450622091512));
#13314=CARTESIAN_POINT('Ctrl Pts',(13.7465187613193,13.7835653267336,-2.4384787180816));
#13315=CARTESIAN_POINT('Ctrl Pts',(14.2941137583008,14.3764510158762,-2.34406982037813));
#13316=CARTESIAN_POINT('Ctrl Pts',(14.8417087552824,14.9693534649946,-2.2496825286364));
#13317=CARTESIAN_POINT('Ctrl Pts',(15.3208543776412,15.4881379273167,-2.16708696976893));
#13318=CARTESIAN_POINT('Ctrl Pts',(15.5946518761319,15.7845797896778,-2.11988125471032));
#13319=CARTESIAN_POINT('Ctrl Pts',(15.7315506253773,15.9328023798814,-2.09628053589475));
#13320=CARTESIAN_POINT('Ctrl Pts',(15.8,16.0069121954757,-2.08447826919396));
#13321=CARTESIAN_POINT('Ctrl Pts',(10.0502525316942,9.60383008034201,-3.1022368453188));
#13322=CARTESIAN_POINT('Ctrl Pts',(11.1454425256572,10.7718807970721,-2.92542368552957));
#13323=CARTESIAN_POINT('Ctrl Pts',(12.3775312688656,12.0859609655105,-2.72674232124834));
#13324=CARTESIAN_POINT('Ctrl Pts',(13.7465187613193,13.5460266034681,-2.50574851695231));
#13325=CARTESIAN_POINT('Ctrl Pts',(14.2941137583008,14.1300531231308,-2.41735366657092));
#13326=CARTESIAN_POINT('Ctrl Pts',(14.8417087552823,14.7140823594691,-2.3289862555658));
#13327=CARTESIAN_POINT('Ctrl Pts',(15.3208543776412,15.2251071015168,-2.25165628918294));
#13328=CARTESIAN_POINT('Ctrl Pts',(15.5946518761319,15.5171202021386,-2.20745725592095));
#13329=CARTESIAN_POINT('Ctrl Pts',(15.7315506253773,15.6631270213657,-2.18536045543709));
#13330=CARTESIAN_POINT('Ctrl Pts',(15.8,15.7361301911613,-2.17430963295026));
#13331=CARTESIAN_POINT('Ctrl Pts',(10.0502525316942,9.33616641898042,-3.16416975479848));
#13332=CARTESIAN_POINT('Ctrl Pts',(11.1454425256572,10.4789053528453,-3.00789330574876));
#13333=CARTESIAN_POINT('Ctrl Pts',(12.3775312688656,11.7645911992084,-2.83212323706007));
#13334=CARTESIAN_POINT('Ctrl Pts',(13.7465187613193,13.1930250082462,-2.6367816468882));
#13335=CARTESIAN_POINT('Ctrl Pts',(14.2941137583008,13.7643997282132,-2.55864547926933));
#13336=CARTESIAN_POINT('Ctrl Pts',(14.8417087552823,14.3357867368398,-2.48051412346291));
#13337=CARTESIAN_POINT('Ctrl Pts',(15.3208543776412,14.8357465708549,-2.4121476997586));
#13338=CARTESIAN_POINT('Ctrl Pts',(15.5946518761319,15.1214332106675,-2.37307933395525));
#13339=CARTESIAN_POINT('Ctrl Pts',(15.7315506253773,15.2642777469938,-2.35354562736143));
#13340=CARTESIAN_POINT('Ctrl Pts',(15.8,15.3356989303604,-2.34377834929582));
#13341=CARTESIAN_POINT('Ctrl Pts',(10.0502525316942,9.08015411140624,-3.1498793996228));
#13342=CARTESIAN_POINT('Ctrl Pts',(11.1454425256572,10.19428901683,-3.0067293155267));
#13343=CARTESIAN_POINT('Ctrl Pts',(12.3775312688656,11.4477380681646,-2.84574388114627));
#13344=CARTESIAN_POINT('Ctrl Pts',(13.7465187613193,12.8404112867165,-2.66681194224705));
#13345=CARTESIAN_POINT('Ctrl Pts',(14.2941137583008,13.3974811152093,-2.59523983509502));
#13346=CARTESIAN_POINT('Ctrl Pts',(14.8417087552823,13.9545565014729,-2.52367459367682));
#13347=CARTESIAN_POINT('Ctrl Pts',(15.3208543776412,14.4419957464975,-2.46105288517697));
#13348=CARTESIAN_POINT('Ctrl Pts',(15.5946518761319,14.7205303350335,-2.42526642923796));
#13349=CARTESIAN_POINT('Ctrl Pts',(15.7315506253773,14.8597981794496,-2.40737388088826));
#13350=CARTESIAN_POINT('Ctrl Pts',(15.8,14.9294316110386,-2.39842700063225));
#13351=CARTESIAN_POINT('Ctrl Pts',(10.0502525316942,8.83780343943476,-3.10442465522081));
#13352=CARTESIAN_POINT('Ctrl Pts',(11.1454425256572,9.9230791616099,-2.96904269314958));
#13353=CARTESIAN_POINT('Ctrl Pts',(12.3775312688656,11.1440266947135,-2.81681208487056));
#13354=CARTESIAN_POINT('Ctrl Pts',(13.7465187613194,12.5006225450517,-2.64759182043347));
#13355=CARTESIAN_POINT('Ctrl Pts',(14.2941137583009,13.0432610264625,-2.57990456259871));
#13356=CARTESIAN_POINT('Ctrl Pts',(14.8417087552824,13.585900959023,-2.51222601461465));
#13357=CARTESIAN_POINT('Ctrl Pts',(15.3208543776412,14.0607104514503,-2.45300459283688));
#13358=CARTESIAN_POINT('Ctrl Pts',(15.594651876132,14.3320296071118,-2.41916045348294));
#13359=CARTESIAN_POINT('Ctrl Pts',(15.7315506253773,14.4676893285878,-2.40223924596973));
#13360=CARTESIAN_POINT('Ctrl Pts',(15.8,14.5355190612237,-2.39377787334028));
#13361=CARTESIAN_POINT('Ctrl Pts',(10.0502525316942,8.72224646189196,-3.06201554081689));
#13362=CARTESIAN_POINT('Ctrl Pts',(11.1454425256572,9.79262845293104,-2.92828468444751));
#13363=CARTESIAN_POINT('Ctrl Pts',(12.3775312688656,10.9969124481398,-2.77780914227504));
#13364=CARTESIAN_POINT('Ctrl Pts',(13.7465187613193,12.3349000504671,-2.61064282371592));
#13365=CARTESIAN_POINT('Ctrl Pts',(14.2941137583008,12.870096284426,-2.54377597211689));
#13366=CARTESIAN_POINT('Ctrl Pts',(14.8417087552824,13.4053047729009,-2.47690579066087));
#13367=CARTESIAN_POINT('Ctrl Pts',(15.3208543776412,13.8736084123374,-2.41839541117504));
#13368=CARTESIAN_POINT('Ctrl Pts',(15.5946518761319,14.1412058111469,-2.38496218052017));
#13369=CARTESIAN_POINT('Ctrl Pts',(15.7315506253773,14.2750057235919,-2.3682452355795));
#13370=CARTESIAN_POINT('Ctrl Pts',(15.8,14.3419045980318,-2.35988705705642));
#13371=CARTESIAN_POINT('Ctrl Pts',(10.0502525316942,8.64769560732005,-3.02626384252387));
#13372=CARTESIAN_POINT('Ctrl Pts',(11.1454425256572,9.70806748165927,-2.89260526381667));
#13373=CARTESIAN_POINT('Ctrl Pts',(12.3775312688656,10.9009858402909,-2.74223936277106));
#13374=CARTESIAN_POINT('Ctrl Pts',(13.7465187613193,12.2264506832149,-2.57516613938705));
#13375=CARTESIAN_POINT('Ctrl Pts',(14.2941137583008,12.7566366203845,-2.50833685003344));
#13376=CARTESIAN_POINT('Ctrl Pts',(14.8417087552824,13.2868225575541,-2.44150756067984));
#13377=CARTESIAN_POINT('Ctrl Pts',(15.3208543776412,13.7507352525775,-2.38303193249544));
#13378=CARTESIAN_POINT('Ctrl Pts',(15.5946518761319,14.0158282211623,-2.34961728781863));
#13379=CARTESIAN_POINT('Ctrl Pts',(15.7315506253773,14.1483747054547,-2.33290996548023));
#13380=CARTESIAN_POINT('Ctrl Pts',(15.8,14.2146479476009,-2.32455630431103));
#13381=CARTESIAN_POINT('',(15.8,14.2146479476009,-2.32455630431103));
#13382=CARTESIAN_POINT('Ctrl Pts',(15.8,14.2566004799664,-2.33570557485288));
#13383=CARTESIAN_POINT('Ctrl Pts',(15.8,14.2481979205348,-2.33357202566326));
#13384=CARTESIAN_POINT('Ctrl Pts',(15.8,14.2398013892846,-2.33139031275994));
#13385=CARTESIAN_POINT('Ctrl Pts',(15.8,14.2314108839843,-2.32916045010432));
#13386=CARTESIAN_POINT('Ctrl Pts',(15.8,14.2230264034132,-2.326882447186));
#13387=CARTESIAN_POINT('Ctrl Pts',(15.8,14.2146479476009,-2.32455630431103));
#13388=CARTESIAN_POINT('Ctrl Pts',(10.0502525316942,8.64769560732005,-3.02626384252387));
#13389=CARTESIAN_POINT('Ctrl Pts',(10.2399538592853,8.8379156589892,-3.00625338967613));
#13390=CARTESIAN_POINT('Ctrl Pts',(10.4321310528899,9.02976542249266,-2.98528677263247));
#13391=CARTESIAN_POINT('Ctrl Pts',(10.6260535771571,9.2224931401807,-2.96359080496244));
#13392=CARTESIAN_POINT('Ctrl Pts',(10.8154434277103,9.41071611112395,-2.9424019508561));
#13393=CARTESIAN_POINT('Ctrl Pts',(11.0064979730134,9.59977633037444,-2.92051732350852));
#13394=CARTESIAN_POINT('Ctrl Pts',(11.1985367155046,9.78902046263136,-2.89813133617984));
#13395=CARTESIAN_POINT('Ctrl Pts',(11.389602998892,9.97730628732557,-2.87585870856646));
#13396=CARTESIAN_POINT('Ctrl Pts',(11.581643537013,10.1657740234639,-2.85308955972937));
#13397=CARTESIAN_POINT('Ctrl Pts',(11.7739881178967,10.3538294697525,-2.83000106681659));
#13398=CARTESIAN_POINT('Ctrl Pts',(11.9659332365647,10.5414943615222,-2.80696052420475));
#13399=CARTESIAN_POINT('Ctrl Pts',(12.1581811364316,10.7287485903511,-2.78360167031422));
#13400=CARTESIAN_POINT('Ctrl Pts',(12.3500657725596,10.9150525380988,-2.76009024231676));
#13401=CARTESIAN_POINT('Ctrl Pts',(12.5349538836681,11.0945634446842,-2.73743609136633));
#13402=CARTESIAN_POINT('Ctrl Pts',(12.7195047388315,11.2731923646039,-2.7146399954872));
#13403=CARTESIAN_POINT('Ctrl Pts',(12.9031225251803,11.4505020946774,-2.69184501333336));
#13404=CARTESIAN_POINT('Ctrl Pts',(13.0466099992771,11.5890601603578,-2.67403195460754));
#13405=CARTESIAN_POINT('Ctrl Pts',(13.1909144693232,11.7281274609627,-2.65603885317597));
#13406=CARTESIAN_POINT('Ctrl Pts',(13.3358225135832,11.8675036836248,-2.63790201856914));
#13407=CARTESIAN_POINT('Ctrl Pts',(13.4722456635829,11.9987189203477,-2.6208271617472));
#13408=CARTESIAN_POINT('Ctrl Pts',(13.6092037742271,12.1302080042448,-2.60362489076148));
#13409=CARTESIAN_POINT('Ctrl Pts',(13.7465187613193,12.2618085151784,-2.58632488288814));
#13410=CARTESIAN_POINT('Ctrl Pts',(13.8831227642785,12.3927276301685,-2.56911445031434));
#13411=CARTESIAN_POINT('Ctrl Pts',(14.0200799576114,12.5237570157981,-2.55180727580019));
#13412=CARTESIAN_POINT('Ctrl Pts',(14.1572150090555,12.6547407331994,-2.53443232271127));
#13413=CARTESIAN_POINT('Ctrl Pts',(14.4088349682216,12.8950740198163,-2.50255218017504));
#13414=CARTESIAN_POINT('Ctrl Pts',(14.6610537068599,13.135250418528,-2.47044377568183));
#13415=CARTESIAN_POINT('Ctrl Pts',(14.912788167059,13.3743428798829,-2.43828616201197));
#13416=CARTESIAN_POINT('Ctrl Pts',(14.9347318651883,13.3951845747101,-2.43548298215979));
#13417=CARTESIAN_POINT('Ctrl Pts',(14.9566718834733,13.4160180659858,-2.43267942911461));
#13418=CARTESIAN_POINT('Ctrl Pts',(14.9786075045277,13.4368427586266,-2.42987562206087));
#13419=CARTESIAN_POINT('Ctrl Pts',(15.1157365203996,13.5670268824575,-2.4123478164419));
#13420=CARTESIAN_POINT('Ctrl Pts',(15.252693690801,13.6968667539964,-2.39481006097156));
#13421=CARTESIAN_POINT('Ctrl Pts',(15.3893037522639,13.8262197421006,-2.37729164508551));
#13422=CARTESIAN_POINT('Ctrl Pts',(15.4578478923357,13.8911226433977,-2.368501774563));
#13423=CARTESIAN_POINT('Ctrl Pts',(15.5263046465628,13.9559030572658,-2.35971677469616));
#13424=CARTESIAN_POINT('Ctrl Pts',(15.5946518761319,14.0205434363407,-2.35094037726561));
#13425=CARTESIAN_POINT('Ctrl Pts',(15.663218932117,14.085391719422,-2.34213575215115));
#13426=CARTESIAN_POINT('Ctrl Pts',(15.7316757577788,14.1500990399651,-2.33333979124571));
#13427=CARTESIAN_POINT('Ctrl Pts',(15.8,14.2146479476009,-2.32455630431103));
#13428=CARTESIAN_POINT('Origin',(15.8,15.0204902775358,-1.08357274193521));
#13429=CARTESIAN_POINT('Origin',(15.8,0.,0.));
#13430=CARTESIAN_POINT('Origin',(13.3251262658471,0.,0.));
#13431=CARTESIAN_POINT('',(15.8,-14.4034641071566,-1.76391562154631E-15));
#13432=CARTESIAN_POINT('',(13.3251262658471,-12.1473403730037,-1.48762015059523E-15));
#13433=CARTESIAN_POINT('Origin',(15.8,0.,0.));
#13434=CARTESIAN_POINT('',(15.8,-14.2372609598209,-2.18178336415567));
#13435=CARTESIAN_POINT('Ctrl Pts',(10.5501326772895,-9.61762388247333,-4.38386896228771E-10));
#13436=CARTESIAN_POINT('Ctrl Pts',(11.3205407897314,-10.3199368948271,-0.318347952011169));
#13437=CARTESIAN_POINT('Ctrl Pts',(12.1203771071554,-11.0330476815418,-0.652342287974112));
#13438=CARTESIAN_POINT('Ctrl Pts',(13.8535773385734,-12.5583034272282,-1.37415173034123));
#13439=CARTESIAN_POINT('Ctrl Pts',(14.8398793216181,-13.4127296512147,-1.78409574717497));
#13440=CARTESIAN_POINT('Ctrl Pts',(15.8,-14.2372609598209,-2.18178336415567));
#13441=CARTESIAN_POINT('Origin',(15.8,0.,0.));
#13442=CARTESIAN_POINT('',(15.8,-12.8662316724636,-6.47455487556025));
#13443=CARTESIAN_POINT('Ctrl Pts',(10.0502525316942,-8.77492596468499,-2.63468906623289));
#13444=CARTESIAN_POINT('Ctrl Pts',(10.2391461906127,-8.9164502426962,-2.76214144474561));
#13445=CARTESIAN_POINT('Ctrl Pts',(10.4304946780272,-9.05872439496926,-2.89131047500302));
#13446=CARTESIAN_POINT('Ctrl Pts',(10.6235767498548,-9.20127947078457,-3.02157840065359));
#13447=CARTESIAN_POINT('Ctrl Pts',(10.8128907594447,-9.34105253585759,-3.14930410347228));
#13448=CARTESIAN_POINT('Ctrl Pts',(11.003871350703,-9.48109547783796,-3.27808626456685));
#13449=CARTESIAN_POINT('Ctrl Pts',(11.1958386868234,-9.6209944304455,-3.40738413972936));
#13450=CARTESIAN_POINT('Ctrl Pts',(11.3869496174041,-9.76026926521909,-3.53610519063208));
#13451=CARTESIAN_POINT('Ctrl Pts',(11.5790385083443,-9.89940114828137,-3.66533747024572));
#13452=CARTESIAN_POINT('Ctrl Pts',(11.7714345809798,-10.0380132338096,-3.79458803732579));
#13453=CARTESIAN_POINT('Ctrl Pts',(11.963522415819,-10.1764032488808,-3.92363153203988));
#13454=CARTESIAN_POINT('Ctrl Pts',(12.1559164488704,-10.3142748929476,-4.05269344373601));
#13455=CARTESIAN_POINT('Ctrl Pts',(12.3479491202715,-10.4512882521924,-4.18132152636412));
#13456=CARTESIAN_POINT('Ctrl Pts',(12.5335453523396,-10.5837092773923,-4.30563832776951));
#13457=CARTESIAN_POINT('Ctrl Pts',(12.7188040406165,-10.7153286091805,-4.42955027592032));
#13458=CARTESIAN_POINT('Ctrl Pts',(12.9031225251803,-10.8458735001829,-4.55268038845334));
#13459=CARTESIAN_POINT('Ctrl Pts',(13.1554739610253,-11.0246032177402,-4.72125849263535));
#13460=CARTESIAN_POINT('Ctrl Pts',(13.4103523866339,-11.2042784469548,-4.89121179563063));
#13461=CARTESIAN_POINT('Ctrl Pts',(13.6665968506683,-11.3841414734476,-5.06174747048486));
#13462=CARTESIAN_POINT('Ctrl Pts',(13.9194672603243,-11.5616361848461,-5.2300376465239));
#13463=CARTESIAN_POINT('Ctrl Pts',(14.1736679711014,-11.7393134647369,-5.39889509460765));
#13464=CARTESIAN_POINT('Ctrl Pts',(14.428083290334,-11.9164831860886,-5.56759036901415));
#13465=CARTESIAN_POINT('Ctrl Pts',(14.6797373390534,-12.0917300140828,-5.73445472660187));
#13466=CARTESIAN_POINT('Ctrl Pts',(14.9316013630469,-12.2664800265877,-5.9011605955206));
#13467=CARTESIAN_POINT('Ctrl Pts',(15.1825956039693,-12.4401067548811,-6.06703163029926));
#13468=CARTESIAN_POINT('Ctrl Pts',(15.3891870324172,-12.5830175789824,-6.2035588027441));
#13469=CARTESIAN_POINT('Ctrl Pts',(15.5951891994095,-12.7251681216495,-6.3395209766308));
#13470=CARTESIAN_POINT('Ctrl Pts',(15.8,-12.8662316724636,-6.47455487556025));
#13471=CARTESIAN_POINT('Origin',(15.8,0.,0.));
#13472=CARTESIAN_POINT('',(15.8,-10.2357659846983,-10.1335518448686));
#13473=CARTESIAN_POINT('Ctrl Pts',(10.0502525316942,-7.53128682236137,-5.21733945232202));
#13474=CARTESIAN_POINT('Ctrl Pts',(10.2399700857352,-7.62691474601356,-5.38300672530998));
#13475=CARTESIAN_POINT('Ctrl Pts',(10.4321639293634,-7.72272706183512,-5.55055481152833));
#13476=CARTESIAN_POINT('Ctrl Pts',(10.6261033397486,-7.81846533797986,-5.71924202232276));
#13477=CARTESIAN_POINT('Ctrl Pts',(10.815494732925,-7.9119584834078,-5.88397339796183));
#13478=CARTESIAN_POINT('Ctrl Pts',(11.0065507832424,-8.00538083967114,-6.04979105175822));
#13479=CARTESIAN_POINT('Ctrl Pts',(11.1985909796536,-8.09850566734927,-6.21605213671099));
#13480=CARTESIAN_POINT('Ctrl Pts',(11.3896566244814,-8.19115791194337,-6.38146949203504));
#13481=CARTESIAN_POINT('Ctrl Pts',(11.5816964522019,-8.28351537255339,-6.54732580586895));
#13482=CARTESIAN_POINT('Ctrl Pts',(11.774040259505,-8.37537212829127,-6.71303622283048));
#13483=CARTESIAN_POINT('Ctrl Pts',(11.9659830376821,-8.46703736637656,-6.87840114021702));
#13484=CARTESIAN_POINT('Ctrl Pts',(12.1582285291929,-8.55820369955463,-7.04362087245224));
#13485=CARTESIAN_POINT('Ctrl Pts',(12.350110714034,-8.64868803888439,-7.20816146064353));
#13486=CARTESIAN_POINT('Ctrl Pts',(12.5349837899972,-8.73586714908811,-7.36669167899034));
#13487=CARTESIAN_POINT('Ctrl Pts',(12.7195196163976,-8.82241309395645,-7.52459184596087));
#13488=CARTESIAN_POINT('Ctrl Pts',(12.9031225251803,-8.90818466253794,-7.68142427504574));
#13489=CARTESIAN_POINT('Ctrl Pts',(13.0466099992771,-8.97521598468134,-7.80399035667839));
#13490=CARTESIAN_POINT('Ctrl Pts',(13.1909144693232,-9.04240096834747,-7.92707423833476));
#13491=CARTESIAN_POINT('Ctrl Pts',(13.3358225135832,-9.10965124727546,-8.05049252087456));
#13492=CARTESIAN_POINT('Ctrl Pts',(13.4722456635829,-9.17296377720826,-8.16668421304467));
#13493=CARTESIAN_POINT('Ctrl Pts',(13.6092037742271,-9.23633418862365,-8.28317233887351));
#13494=CARTESIAN_POINT('Ctrl Pts',(13.7465187613193,-9.29969102606761,-8.39980806233602));
#13495=CARTESIAN_POINT('Ctrl Pts',(13.8831227642785,-9.36271981697347,-8.51583987394238));
#13496=CARTESIAN_POINT('Ctrl Pts',(14.0200799576114,-9.42573515876482,-8.63201776215884));
#13497=CARTESIAN_POINT('Ctrl Pts',(14.1572150090555,-9.48866882093701,-8.74819853760654));
#13498=CARTESIAN_POINT('Ctrl Pts',(14.4088743845442,-9.60415968890035,-8.96140428686672));
#13499=CARTESIAN_POINT('Ctrl Pts',(14.6611327271176,-9.71937357878302,-9.17461726586999));
#13500=CARTESIAN_POINT('Ctrl Pts',(14.9129064698008,-9.83391026822831,-9.38698186590304));
#13501=CARTESIAN_POINT('Ctrl Pts',(14.9348107204665,-9.84387493066409,-9.40545753132419));
#13502=CARTESIAN_POINT('Ctrl Pts',(14.9567113032174,-9.85383448723409,-9.42392680146211));
#13503=CARTESIAN_POINT('Ctrl Pts',(14.9786075045277,-9.86378868594609,-9.44238912780876));
#13504=CARTESIAN_POINT('Ctrl Pts',(15.1157365203996,-9.92612869889287,-9.55801286576867));
#13505=CARTESIAN_POINT('Ctrl Pts',(15.252693690801,-9.98825831748494,-9.67336395156665));
#13506=CARTESIAN_POINT('Ctrl Pts',(15.3893037522639,-10.0501174002428,-9.78830977806043));
#13507=CARTESIAN_POINT('Ctrl Pts',(15.4578478923357,-10.0811552139138,-9.84598388161831));
#13508=CARTESIAN_POINT('Ctrl Pts',(15.5263046465628,-10.1121249718658,-9.90355602888934));
#13509=CARTESIAN_POINT('Ctrl Pts',(15.5946518761319,-10.1430193787867,-9.96100982960575));
#13510=CARTESIAN_POINT('Ctrl Pts',(15.663218932117,-10.1740131519407,-10.0186484200082));
#13511=CARTESIAN_POINT('Ctrl Pts',(15.7316757577788,-10.2049310789385,-10.076167877539));
#13512=CARTESIAN_POINT('Ctrl Pts',(15.8,-10.2357659846983,-10.1335518448686));
#13513=CARTESIAN_POINT('Origin',(15.8,0.,0.));
#13514=CARTESIAN_POINT('',(15.8,-6.60335220557564,-12.8006061549939));
#13515=CARTESIAN_POINT('Ctrl Pts',(10.0502525316942,-5.55043285230422,-7.28928030147641));
#13516=CARTESIAN_POINT('Ctrl Pts',(10.2399762236023,-5.5901876956016,-7.4763959480264));
#13517=CARTESIAN_POINT('Ctrl Pts',(10.4321763653293,-5.62953666502947,-7.66535745978647));
#13518=CARTESIAN_POINT('Ctrl Pts',(10.6261221631202,-5.66846318065116,-7.85537951329684));
#13519=CARTESIAN_POINT('Ctrl Pts',(10.8155134734716,-5.70647557321124,-8.04093922183353));
#13520=CARTESIAN_POINT('Ctrl Pts',(11.0065694150242,-5.74408496164277,-8.22751014665864));
#13521=CARTESIAN_POINT('Ctrl Pts',(11.1986094788125,-5.78127435838156,-8.41441083753434));
#13522=CARTESIAN_POINT('Ctrl Pts',(11.389674403306,-5.81827491513876,-8.60036248577636));
#13523=CARTESIAN_POINT('Ctrl Pts',(11.5817134810757,-5.85485947501131,-8.78664049259207));
#13524=CARTESIAN_POINT('Ctrl Pts',(11.7740565170535,-5.89101292727639,-8.97262500016449));
#13525=CARTESIAN_POINT('Ctrl Pts',(11.9659982062668,-5.92709094103641,-9.15822142880287));
#13526=CARTESIAN_POINT('Ctrl Pts',(12.1582425865211,-5.96273934048993,-9.34352559234182));
#13527=CARTESIAN_POINT('Ctrl Pts',(12.350123649327,-5.9979490001613,-9.5279730968269));
#13528=CARTESIAN_POINT('Ctrl Pts',(12.5349923977945,-6.03187191898524,-9.70567994717204));
#13529=CARTESIAN_POINT('Ctrl Pts',(12.7195238985382,-6.06538737998552,-9.88259194572981));
#13530=CARTESIAN_POINT('Ctrl Pts',(12.9031225251803,-6.0984963351851,-10.0582492231335));
#13531=CARTESIAN_POINT('Ctrl Pts',(13.0466099992771,-6.12437191191712,-10.1955303101566));
#13532=CARTESIAN_POINT('Ctrl Pts',(13.1909144693232,-6.15023362158894,-10.3333513349338));
#13533=CARTESIAN_POINT('Ctrl Pts',(13.3358225135832,-6.17605409599263,-10.4715105676525));
#13534=CARTESIAN_POINT('Ctrl Pts',(13.4722456635829,-6.20036268749026,-10.6015800736297));
#13535=CARTESIAN_POINT('Ctrl Pts',(13.6092037742271,-6.22463472522239,-10.7319493881454));
#13536=CARTESIAN_POINT('Ctrl Pts',(13.7465187613193,-6.24884824365307,-10.8624548834565));
#13537=CARTESIAN_POINT('Ctrl Pts',(13.8831227642785,-6.27293639028148,-10.9922846525529));
#13538=CARTESIAN_POINT('Ctrl Pts',(14.0200799576114,-6.29696660630782,-11.1222491940658));
#13539=CARTESIAN_POINT('Ctrl Pts',(14.1572150090555,-6.32091824773854,-11.2521912379382));
#13540=CARTESIAN_POINT('Ctrl Pts',(14.4088957070015,-6.36487612552952,-11.4906707801847));
#13541=CARTESIAN_POINT('Ctrl Pts',(14.6611754735345,-6.40856830116458,-11.7290715847991));
#13542=CARTESIAN_POINT('Ctrl Pts',(14.9129704662325,-6.45187850892463,-11.9664560266787));
#13543=CARTESIAN_POINT('Ctrl Pts',(14.9348533776129,-6.45564249735079,-11.987086550936));
#13544=CARTESIAN_POINT('Ctrl Pts',(14.9567326275257,-6.45940361158542,-12.0077094295138));
#13545=CARTESIAN_POINT('Ctrl Pts',(14.9786075045277,-6.46316178167156,-12.0283240646364));
#13546=CARTESIAN_POINT('Ctrl Pts',(15.1157365203996,-6.48672096169998,-12.1575528884896));
#13547=CARTESIAN_POINT('Ctrl Pts',(15.252693690801,-6.5101642983752,-12.2864573923713));
#13548=CARTESIAN_POINT('Ctrl Pts',(15.3893037522639,-6.53347557107031,-12.4148928744451));
#13549=CARTESIAN_POINT('Ctrl Pts',(15.4578478923357,-6.54517200926641,-12.4793354168112));
#13550=CARTESIAN_POINT('Ctrl Pts',(15.5263046465628,-6.5568352285584,-12.5436599631772));
#13551=CARTESIAN_POINT('Ctrl Pts',(15.5946518761319,-6.56846335549623,-12.6078486707221));
#13552=CARTESIAN_POINT('Ctrl Pts',(15.663218932117,-6.58012888218654,-12.6722438295541));
#13553=CARTESIAN_POINT('Ctrl Pts',(15.7316757577788,-6.59175908863286,-12.7365022490344));
#13554=CARTESIAN_POINT('Ctrl Pts',(15.8,-6.60335220557564,-12.8006061549939));
#13555=CARTESIAN_POINT('Origin',(15.8,0.,0.));
#13556=CARTESIAN_POINT('',(15.8,-2.32455630431103,-14.2146479476009));
#13557=CARTESIAN_POINT('Ctrl Pts',(10.0502525316942,-3.02626384252387,-8.64769560732005));
#13558=CARTESIAN_POINT('Ctrl Pts',(10.239953859285,-3.00625338967615,-8.83791565898895));
#13559=CARTESIAN_POINT('Ctrl Pts',(10.4321310528894,-2.98528677263252,-9.02976542249216));
#13560=CARTESIAN_POINT('Ctrl Pts',(10.6260535771564,-2.96359080496253,-9.22249314017995));
#13561=CARTESIAN_POINT('Ctrl Pts',(10.8154434277096,-2.94240195085618,-9.41071611112327));
#13562=CARTESIAN_POINT('Ctrl Pts',(11.0064979730128,-2.92051732350859,-9.59977633037382));
#13563=CARTESIAN_POINT('Ctrl Pts',(11.1985367155041,-2.8981313361799,-9.78902046263081));
#13564=CARTESIAN_POINT('Ctrl Pts',(11.3896029988914,-2.87585870856653,-9.97730628732503));
#13565=CARTESIAN_POINT('Ctrl Pts',(11.5816435370124,-2.85308955972943,-10.1657740234633));
#13566=CARTESIAN_POINT('Ctrl Pts',(11.7739881178962,-2.83000106681665,-10.353829469752));
#13567=CARTESIAN_POINT('Ctrl Pts',(11.9659332365641,-2.80696052420482,-10.5414943615216));
#13568=CARTESIAN_POINT('Ctrl Pts',(12.158181136431,-2.7836016703143,-10.7287485903505));
#13569=CARTESIAN_POINT('Ctrl Pts',(12.350065772559,-2.76009024231684,-10.9150525380982));
#13570=CARTESIAN_POINT('Ctrl Pts',(12.5349538836676,-2.73743609136638,-11.0945634446838));
#13571=CARTESIAN_POINT('Ctrl Pts',(12.7195047388313,-2.71463999548723,-11.2731923646037));
#13572=CARTESIAN_POINT('Ctrl Pts',(12.9031225251803,-2.69184501333336,-11.4505020946774));
#13573=CARTESIAN_POINT('Ctrl Pts',(13.0466099992771,-2.67403195460754,-11.5890601603578));
#13574=CARTESIAN_POINT('Ctrl Pts',(13.1909144693232,-2.65603885317597,-11.7281274609627));
#13575=CARTESIAN_POINT('Ctrl Pts',(13.3358225135832,-2.63790201856914,-11.8675036836248));
#13576=CARTESIAN_POINT('Ctrl Pts',(13.4722456635829,-2.6208271617472,-11.9987189203477));
#13577=CARTESIAN_POINT('Ctrl Pts',(13.6092037742271,-2.60362489076148,-12.1302080042448));
#13578=CARTESIAN_POINT('Ctrl Pts',(13.7465187613193,-2.58632488288814,-12.2618085151784));
#13579=CARTESIAN_POINT('Ctrl Pts',(13.8831227642785,-2.56911445031434,-12.3927276301685));
#13580=CARTESIAN_POINT('Ctrl Pts',(14.0200799576114,-2.55180727580019,-12.5237570157982));
#13581=CARTESIAN_POINT('Ctrl Pts',(14.1572150090555,-2.53443232271127,-12.6547407331994));
#13582=CARTESIAN_POINT('Ctrl Pts',(14.4088349682216,-2.50255218017505,-12.8950740198162));
#13583=CARTESIAN_POINT('Ctrl Pts',(14.6610537068598,-2.47044377568185,-13.1352504185278));
#13584=CARTESIAN_POINT('Ctrl Pts',(14.9127881670588,-2.438286162012,-13.3743428798827));
#13585=CARTESIAN_POINT('Ctrl Pts',(14.9347318651881,-2.43548298215981,-13.3951845747099));
#13586=CARTESIAN_POINT('Ctrl Pts',(14.9566718834732,-2.43267942911462,-13.4160180659858));
#13587=CARTESIAN_POINT('Ctrl Pts',(14.9786075045277,-2.42987562206087,-13.4368427586266));
#13588=CARTESIAN_POINT('Ctrl Pts',(15.1157365203996,-2.4123478164419,-13.5670268824575));
#13589=CARTESIAN_POINT('Ctrl Pts',(15.252693690801,-2.39481006097156,-13.6968667539964));
#13590=CARTESIAN_POINT('Ctrl Pts',(15.3893037522639,-2.3772916450855,-13.8262197421006));
#13591=CARTESIAN_POINT('Ctrl Pts',(15.4578478923357,-2.368501774563,-13.8911226433977));
#13592=CARTESIAN_POINT('Ctrl Pts',(15.5263046465628,-2.35971677469615,-13.9559030572658));
#13593=CARTESIAN_POINT('Ctrl Pts',(15.5946518761319,-2.3509403772656,-14.0205434363407));
#13594=CARTESIAN_POINT('Ctrl Pts',(15.663218932117,-2.34213575215115,-14.085391719422));
#13595=CARTESIAN_POINT('Ctrl Pts',(15.7316757577788,-2.33333979124571,-14.1500990399651));
#13596=CARTESIAN_POINT('Ctrl Pts',(15.8,-2.32455630431103,-14.2146479476009));
#13597=CARTESIAN_POINT('Origin',(15.8,0.,0.));
#13598=CARTESIAN_POINT('',(15.8,2.18178336415567,-14.2372609598209));
#13599=CARTESIAN_POINT('Ctrl Pts',(10.0502525316942,-0.205863042617262,
-9.15961421508102));
#13600=CARTESIAN_POINT('Ctrl Pts',(10.2391570234258,-0.128377591099423,
-9.33360673051062));
#13601=CARTESIAN_POINT('Ctrl Pts',(10.4305166252241,-0.0494911083977407,
-9.50884304477973));
#13602=CARTESIAN_POINT('Ctrl Pts',(10.6236099689118,0.0303537569978826,
-9.68468614630344));
#13603=CARTESIAN_POINT('Ctrl Pts',(10.8129280637648,0.108637541989126,-9.85709126570177));
#13604=CARTESIAN_POINT('Ctrl Pts',(11.0039127690162,0.187842691359046,-10.0300795089051));
#13605=CARTESIAN_POINT('Ctrl Pts',(11.195884205948,0.267582809353851,-10.2030901320277));
#13606=CARTESIAN_POINT('Ctrl Pts',(11.386997148711,0.346966330412115,-10.3753270535337));
#13607=CARTESIAN_POINT('Ctrl Pts',(11.5790880175811,0.426880221764407,-10.5475859558082));
#13608=CARTESIAN_POINT('Ctrl Pts',(11.7714860143417,0.506972115618924,-10.7193560970323));
#13609=CARTESIAN_POINT('Ctrl Pts',(11.9635738218519,0.586934883157499,-10.8908493057922));
#13610=CARTESIAN_POINT('Ctrl Pts',(12.1559677677311,0.667075331863647,-11.0618551603491));
#13611=CARTESIAN_POINT('Ctrl Pts',(12.3480002929715,0.747068390651276,-11.2319106356083));
#13612=CARTESIAN_POINT('Ctrl Pts',(12.5335794054255,0.824373216142153,-11.3962512551311));
#13613=CARTESIAN_POINT('Ctrl Pts',(12.7188209807522,0.901540748122806,-11.5597044367662));
#13614=CARTESIAN_POINT('Ctrl Pts',(12.9031225251803,0.978296811887799,-11.7218943942307));
#13615=CARTESIAN_POINT('Ctrl Pts',(13.1554719876675,1.08339279192334,-11.9439682173992));
#13616=CARTESIAN_POINT('Ctrl Pts',(13.410348400397,1.18950448019878,-12.1673662092161));
#13617=CARTESIAN_POINT('Ctrl Pts',(13.6665908392661,1.2961120061965,-12.3911227672762));
#13618=CARTESIAN_POINT('Ctrl Pts',(13.9194596713273,1.40131597126551,-12.6119334173481));
#13619=CARTESIAN_POINT('Ctrl Pts',(14.1736587969735,1.50700303047563,-12.8330929959809));
#13620=CARTESIAN_POINT('Ctrl Pts',(14.4280725441416,1.61269270111681,-13.0537197620231));
#13621=CARTESIAN_POINT('Ctrl Pts',(14.6797279548941,1.71723649159025,-13.2719545077841));
#13622=CARTESIAN_POINT('Ctrl Pts',(14.931593358573,1.82178307810192,-13.4896677845277));
#13623=CARTESIAN_POINT('Ctrl Pts',(15.1825889792242,1.92588279207063,-13.7060547738726));
#13624=CARTESIAN_POINT('Ctrl Pts',(15.3891826285177,2.01156691573547,-13.8841621753979));
#13625=CARTESIAN_POINT('Ctrl Pts',(15.5951870101943,2.09694862236073,-14.0613719009699));
#13626=CARTESIAN_POINT('Ctrl Pts',(15.8,2.18178336415567,-14.2372609598209));
#13627=CARTESIAN_POINT('Origin',(15.8,0.,0.));
#13628=CARTESIAN_POINT('',(15.8,6.47455487556025,-12.8662316724636));
#13629=CARTESIAN_POINT('Ctrl Pts',(10.0502525316942,2.63468906623289,-8.77492596468499));
#13630=CARTESIAN_POINT('Ctrl Pts',(10.2391461906127,2.76214144474559,-8.91645024269617));
#13631=CARTESIAN_POINT('Ctrl Pts',(10.4304946780271,2.89131047500297,-9.05872439496921));
#13632=CARTESIAN_POINT('Ctrl Pts',(10.6235767498547,3.02157840065351,-9.20127947078449));
#13633=CARTESIAN_POINT('Ctrl Pts',(10.8128907594447,3.1493041034723,-9.34105253585761));
#13634=CARTESIAN_POINT('Ctrl Pts',(11.0038713507032,3.27808626456696,-9.48109547783808));
#13635=CARTESIAN_POINT('Ctrl Pts',(11.1958386868237,3.40738413972955,-9.62099443044572));
#13636=CARTESIAN_POINT('Ctrl Pts',(11.3869496174045,3.53610519063233,-9.76026926521936));
#13637=CARTESIAN_POINT('Ctrl Pts',(11.5790385083447,3.665337470246,-9.89940114828168));
#13638=CARTESIAN_POINT('Ctrl Pts',(11.7714345809803,3.79458803732612,-10.0380132338099));
#13639=CARTESIAN_POINT('Ctrl Pts',(11.9635224158196,3.92363153204024,-10.1764032488812));
#13640=CARTESIAN_POINT('Ctrl Pts',(12.155916448871,4.05269344373641,-10.314274892948));
#13641=CARTESIAN_POINT('Ctrl Pts',(12.3479491202722,4.18132152636456,-10.4512882521928));
#13642=CARTESIAN_POINT('Ctrl Pts',(12.53354535234,4.30563832776981,-10.5837092773927));
#13643=CARTESIAN_POINT('Ctrl Pts',(12.7188040406167,4.42955027592047,-10.7153286091806));
#13644=CARTESIAN_POINT('Ctrl Pts',(12.9031225251803,4.55268038845334,-10.8458735001829));
#13645=CARTESIAN_POINT('Ctrl Pts',(13.1554739610256,4.72125849263551,-11.0246032177404));
#13646=CARTESIAN_POINT('Ctrl Pts',(13.4103523866344,4.89121179563095,-11.2042784469551));
#13647=CARTESIAN_POINT('Ctrl Pts',(13.666596850669,5.06174747048535,-11.3841414734481));
#13648=CARTESIAN_POINT('Ctrl Pts',(13.9194672603251,5.23003764652439,-11.5616361848466));
#13649=CARTESIAN_POINT('Ctrl Pts',(14.1736679711021,5.39889509460814,-11.7393134647374));
#13650=CARTESIAN_POINT('Ctrl Pts',(14.4280832903348,5.56759036901465,-11.9164831860891));
#13651=CARTESIAN_POINT('Ctrl Pts',(14.6797373390532,5.7344547266017,-12.0917300140826));
#13652=CARTESIAN_POINT('Ctrl Pts',(14.9316013630457,5.90116059551977,-12.2664800265868));
#13653=CARTESIAN_POINT('Ctrl Pts',(15.182595603967,6.06703163029777,-12.4401067548795));
#13654=CARTESIAN_POINT('Ctrl Pts',(15.3891870324157,6.20355880274311,-12.5830175789813));
#13655=CARTESIAN_POINT('Ctrl Pts',(15.5951891994088,6.3395209766303,-12.725168121649));
#13656=CARTESIAN_POINT('Ctrl Pts',(15.8,6.47455487556025,-12.8662316724636));
#13657=CARTESIAN_POINT('Origin',(15.8,0.,0.));
#13658=CARTESIAN_POINT('',(15.8,10.1335518448686,-10.2357659846983));
#13659=CARTESIAN_POINT('Ctrl Pts',(10.0502525316942,5.21733945232202,-7.53128682236137));
#13660=CARTESIAN_POINT('Ctrl Pts',(10.2399700857355,5.38300672531024,-7.62691474601371));
#13661=CARTESIAN_POINT('Ctrl Pts',(10.432163929364,5.55055481152886,-7.72272706183542));
#13662=CARTESIAN_POINT('Ctrl Pts',(10.6261033397496,5.71924202232356,-7.81846533798032));
#13663=CARTESIAN_POINT('Ctrl Pts',(10.815494732926,5.88397339796269,-7.91195848340829));
#13664=CARTESIAN_POINT('Ctrl Pts',(11.0065507832434,6.04979105175912,-8.00538083967165));
#13665=CARTESIAN_POINT('Ctrl Pts',(11.1985909796548,6.21605213671196,-8.09850566734981));
#13666=CARTESIAN_POINT('Ctrl Pts',(11.3896566244822,6.38146949203575,-8.19115791194377));
#13667=CARTESIAN_POINT('Ctrl Pts',(11.5816964522024,6.54732580586942,-8.28351537255365));
#13668=CARTESIAN_POINT('Ctrl Pts',(11.7740402595052,6.71303622283071,-8.3753721282914));
#13669=CARTESIAN_POINT('Ctrl Pts',(11.9659830376824,6.87840114021723,-8.46703736637668));
#13670=CARTESIAN_POINT('Ctrl Pts',(12.1582285291931,7.04362087245244,-8.55820369955474));
#13671=CARTESIAN_POINT('Ctrl Pts',(12.3501107140342,7.20816146064372,-8.64868803888449));
#13672=CARTESIAN_POINT('Ctrl Pts',(12.5349837899974,7.36669167899046,-8.73586714908818));
#13673=CARTESIAN_POINT('Ctrl Pts',(12.7195196163977,7.52459184596093,-8.82241309395648));
#13674=CARTESIAN_POINT('Ctrl Pts',(12.9031225251803,7.68142427504574,-8.90818466253794));
#13675=CARTESIAN_POINT('Ctrl Pts',(13.046609999277,7.80399035667838,-8.97521598468133));
#13676=CARTESIAN_POINT('Ctrl Pts',(13.1909144693232,7.92707423833475,-9.04240096834747));
#13677=CARTESIAN_POINT('Ctrl Pts',(13.3358225135832,8.05049252087456,-9.10965124727546));
#13678=CARTESIAN_POINT('Ctrl Pts',(13.4722456635829,8.16668421304466,-9.17296377720826));
#13679=CARTESIAN_POINT('Ctrl Pts',(13.6092037742271,8.2831723388735,-9.23633418862365));
#13680=CARTESIAN_POINT('Ctrl Pts',(13.7465187613193,8.39980806233602,-9.29969102606761));
#13681=CARTESIAN_POINT('Ctrl Pts',(13.8831227642785,8.51583987394238,-9.36271981697347));
#13682=CARTESIAN_POINT('Ctrl Pts',(14.0200799576114,8.63201776215884,-9.42573515876483));
#13683=CARTESIAN_POINT('Ctrl Pts',(14.1572150090555,8.74819853760654,-9.48866882093701));
#13684=CARTESIAN_POINT('Ctrl Pts',(14.4088743845434,8.96140428686608,-9.6041596889));
#13685=CARTESIAN_POINT('Ctrl Pts',(14.661132727116,9.1746172658687,-9.71937357878233));
#13686=CARTESIAN_POINT('Ctrl Pts',(14.9129064697985,9.38698186590108,-9.83391026822726));
#13687=CARTESIAN_POINT('Ctrl Pts',(14.934810720465,9.40545753132288,-9.84387493066339));
#13688=CARTESIAN_POINT('Ctrl Pts',(14.9567113032167,9.42392680146146,-9.85383448723374));
#13689=CARTESIAN_POINT('Ctrl Pts',(14.9786075045277,9.44238912780876,-9.86378868594609));
#13690=CARTESIAN_POINT('Ctrl Pts',(15.1157365203996,9.55801286576868,-9.92612869889287));
#13691=CARTESIAN_POINT('Ctrl Pts',(15.252693690801,9.67336395156666,-9.98825831748495));
#13692=CARTESIAN_POINT('Ctrl Pts',(15.3893037522639,9.78830977806043,-10.0501174002428));
#13693=CARTESIAN_POINT('Ctrl Pts',(15.4578478923357,9.84598388161831,-10.0811552139138));
#13694=CARTESIAN_POINT('Ctrl Pts',(15.5263046465628,9.90355602888933,-10.1121249718658));
#13695=CARTESIAN_POINT('Ctrl Pts',(15.5946518761319,9.96100982960574,-10.1430193787867));
#13696=CARTESIAN_POINT('Ctrl Pts',(15.663218932117,10.0186484200082,-10.1740131519407));
#13697=CARTESIAN_POINT('Ctrl Pts',(15.7316757577788,10.076167877539,-10.2049310789385));
#13698=CARTESIAN_POINT('Ctrl Pts',(15.8,10.1335518448686,-10.2357659846983));
#13699=CARTESIAN_POINT('Origin',(15.8,0.,0.));
#13700=CARTESIAN_POINT('',(15.8,12.8006061549939,-6.60335220557564));
#13701=CARTESIAN_POINT('Ctrl Pts',(10.0502525316942,7.28928030147641,-5.55043285230422));
#13702=CARTESIAN_POINT('Ctrl Pts',(10.2399762236016,7.47639594802568,-5.59018769560145));
#13703=CARTESIAN_POINT('Ctrl Pts',(10.4321763653278,7.66535745978503,-5.62953666502917));
#13704=CARTESIAN_POINT('Ctrl Pts',(10.626122163118,7.85537951329466,-5.66846318065072));
#13705=CARTESIAN_POINT('Ctrl Pts',(10.8155134734694,8.04093922183132,-5.7064755732108));
#13706=CARTESIAN_POINT('Ctrl Pts',(11.006569415022,8.2275101466564,-5.74408496164232));
#13707=CARTESIAN_POINT('Ctrl Pts',(11.1986094788102,8.41441083753208,-5.78127435838112));
#13708=CARTESIAN_POINT('Ctrl Pts',(11.3896744033038,8.60036248577428,-5.81827491513835));
#13709=CARTESIAN_POINT('Ctrl Pts',(11.5817134810738,8.78664049259016,-5.85485947501094));
#13710=CARTESIAN_POINT('Ctrl Pts',(11.7740565170517,8.97262500016277,-5.89101292727606));
#13711=CARTESIAN_POINT('Ctrl Pts',(11.9659982062651,9.15822142880125,-5.9270909410361));
#13712=CARTESIAN_POINT('Ctrl Pts',(12.1582425865195,9.34352559234031,-5.96273934048964));
#13713=CARTESIAN_POINT('Ctrl Pts',(12.3501236493255,9.52797309682549,-5.99794900016104));
#13714=CARTESIAN_POINT('Ctrl Pts',(12.5349923977935,9.70567994717111,-6.03187191898507));
#13715=CARTESIAN_POINT('Ctrl Pts',(12.7195238985377,9.88259194572934,-6.06538737998544));
#13716=CARTESIAN_POINT('Ctrl Pts',(12.9031225251803,10.0582492231335,-6.09849633518511));
#13717=CARTESIAN_POINT('Ctrl Pts',(13.0466099992771,10.1955303101566,-6.12437191191713));
#13718=CARTESIAN_POINT('Ctrl Pts',(13.1909144693232,10.3333513349338,-6.15023362158894));
#13719=CARTESIAN_POINT('Ctrl Pts',(13.3358225135832,10.4715105676525,-6.17605409599263));
#13720=CARTESIAN_POINT('Ctrl Pts',(13.4722456635829,10.6015800736297,-6.20036268749027));
#13721=CARTESIAN_POINT('Ctrl Pts',(13.6092037742271,10.7319493881454,-6.22463472522239));
#13722=CARTESIAN_POINT('Ctrl Pts',(13.7465187613193,10.8624548834565,-6.24884824365307));
#13723=CARTESIAN_POINT('Ctrl Pts',(13.8831227642785,10.9922846525529,-6.27293639028148));
#13724=CARTESIAN_POINT('Ctrl Pts',(14.0200799576114,11.1222491940658,-6.29696660630782));
#13725=CARTESIAN_POINT('Ctrl Pts',(14.1572150090555,11.2521912379382,-6.32091824773854));
#13726=CARTESIAN_POINT('Ctrl Pts',(14.408895707,11.4906707801833,-6.36487612552926));
#13727=CARTESIAN_POINT('Ctrl Pts',(14.6611754735313,11.7290715847961,-6.40856830116405));
#13728=CARTESIAN_POINT('Ctrl Pts',(14.9129704662278,11.9664560266743,-6.45187850892383));
#13729=CARTESIAN_POINT('Ctrl Pts',(14.9348533776098,11.9870865509331,-6.45564249735026));
#13730=CARTESIAN_POINT('Ctrl Pts',(14.9567326275241,12.0077094295123,-6.45940361158516));
#13731=CARTESIAN_POINT('Ctrl Pts',(14.9786075045277,12.0283240646364,-6.46316178167156));
#13732=CARTESIAN_POINT('Ctrl Pts',(15.1157365203996,12.1575528884896,-6.48672096169998));
#13733=CARTESIAN_POINT('Ctrl Pts',(15.252693690801,12.2864573923713,-6.5101642983752));
#13734=CARTESIAN_POINT('Ctrl Pts',(15.3893037522639,12.4148928744451,-6.53347557107031));
#13735=CARTESIAN_POINT('Ctrl Pts',(15.4578478923357,12.4793354168112,-6.54517200926641));
#13736=CARTESIAN_POINT('Ctrl Pts',(15.5263046465628,12.5436599631772,-6.5568352285584));
#13737=CARTESIAN_POINT('Ctrl Pts',(15.5946518761319,12.6078486707221,-6.56846335549623));
#13738=CARTESIAN_POINT('Ctrl Pts',(15.663218932117,12.6722438295541,-6.58012888218654));
#13739=CARTESIAN_POINT('Ctrl Pts',(15.7316757577788,12.7365022490344,-6.59175908863286));
#13740=CARTESIAN_POINT('Ctrl Pts',(15.8,12.8006061549939,-6.60335220557564));
#13741=CARTESIAN_POINT('Origin',(15.8,0.,0.));
#13742=CARTESIAN_POINT('',(15.8,14.2372609598209,2.18178336415567));
#13743=CARTESIAN_POINT('Ctrl Pts',(10.0502525316942,9.15961421508102,-0.20586304261726));
#13744=CARTESIAN_POINT('Ctrl Pts',(10.2391570234258,9.33360673051055,-0.128377591099454));
#13745=CARTESIAN_POINT('Ctrl Pts',(10.430516625224,9.50884304477959,-0.0494911083978059));
#13746=CARTESIAN_POINT('Ctrl Pts',(10.6236099689116,9.68468614630322,0.0303537569977821));
#13747=CARTESIAN_POINT('Ctrl Pts',(10.8129280637645,9.85709126570154,0.108637541989021));
#13748=CARTESIAN_POINT('Ctrl Pts',(11.0039127690159,10.0300795089048,0.187842691358935));
#13749=CARTESIAN_POINT('Ctrl Pts',(11.1958842059477,10.2030901320274,0.267582809353735));
#13750=CARTESIAN_POINT('Ctrl Pts',(11.3869971487108,10.3753270535335,0.346966330412031));
#13751=CARTESIAN_POINT('Ctrl Pts',(11.579088017581,10.5475859558081,0.426880221764355));
#13752=CARTESIAN_POINT('Ctrl Pts',(11.7714860143417,10.7193560970322,0.506972115618906));
#13753=CARTESIAN_POINT('Ctrl Pts',(11.9635738218519,10.8908493057922,0.586934883157515));
#13754=CARTESIAN_POINT('Ctrl Pts',(12.1559677677312,11.0618551603493,0.667075331863697));
#13755=CARTESIAN_POINT('Ctrl Pts',(12.3480002929717,11.2319106356085,0.747068390651361));
#13756=CARTESIAN_POINT('Ctrl Pts',(12.5335794054256,11.3962512551312,0.824373216142209));
#13757=CARTESIAN_POINT('Ctrl Pts',(12.7188209807523,11.5597044367662,0.901540748122834));
#13758=CARTESIAN_POINT('Ctrl Pts',(12.9031225251803,11.7218943942307,0.978296811887802));
#13759=CARTESIAN_POINT('Ctrl Pts',(13.1554719876668,11.9439682173986,1.08339279192306));
#13760=CARTESIAN_POINT('Ctrl Pts',(13.4103484003956,12.1673662092149,1.18950448019821));
#13761=CARTESIAN_POINT('Ctrl Pts',(13.666590839264,12.3911227672744,1.29611200619563));
#13762=CARTESIAN_POINT('Ctrl Pts',(13.9194596713251,12.6119334173462,1.40131597126461));
#13763=CARTESIAN_POINT('Ctrl Pts',(14.1736587969712,12.8330929959789,1.50700303047468));
#13764=CARTESIAN_POINT('Ctrl Pts',(14.4280725441392,13.053719762021,1.61269270111584));
#13765=CARTESIAN_POINT('Ctrl Pts',(14.6797279548917,13.271954507782,1.71723649158925));
#13766=CARTESIAN_POINT('Ctrl Pts',(14.9315933585706,13.4896677845255,1.82178307810091));
#13767=CARTESIAN_POINT('Ctrl Pts',(15.1825889792217,13.7060547738705,1.9258827920696));
#13768=CARTESIAN_POINT('Ctrl Pts',(15.3891826285161,13.8841621753965,2.01156691573479));
#13769=CARTESIAN_POINT('Ctrl Pts',(15.5951870101935,14.0613719009692,2.09694862236039));
#13770=CARTESIAN_POINT('Ctrl Pts',(15.8,14.2372609598209,2.18178336415567));
#13771=CARTESIAN_POINT('Origin',(15.8,0.,0.));
#13772=CARTESIAN_POINT('',(15.8,12.8662316724636,6.47455487556026));
#13773=CARTESIAN_POINT('Ctrl Pts',(10.0502525316942,8.77492596468499,2.63468906623289));
#13774=CARTESIAN_POINT('Ctrl Pts',(10.2391461906124,8.91645024269597,2.76214144474541));
#13775=CARTESIAN_POINT('Ctrl Pts',(10.4304946780266,9.05872439496881,2.89131047500261));
#13776=CARTESIAN_POINT('Ctrl Pts',(10.6235767498538,9.20127947078389,3.02157840065296));
#13777=CARTESIAN_POINT('Ctrl Pts',(10.8128907594439,9.34105253585702,3.14930410347176));
#13778=CARTESIAN_POINT('Ctrl Pts',(11.0038713507024,9.48109547783751,3.27808626456643));
#13779=CARTESIAN_POINT('Ctrl Pts',(11.195838686823,9.62099443044516,3.40738413972904));
#13780=CARTESIAN_POINT('Ctrl Pts',(11.3869496174036,9.76026926521869,3.53610519063172));
#13781=CARTESIAN_POINT('Ctrl Pts',(11.5790385083437,9.89940114828092,3.6653374702453));
#13782=CARTESIAN_POINT('Ctrl Pts',(11.7714345809791,10.0380132338091,3.79458803732532));
#13783=CARTESIAN_POINT('Ctrl Pts',(11.9635224158183,10.1764032488802,3.92363153203936));
#13784=CARTESIAN_POINT('Ctrl Pts',(12.1559164488696,10.314274892947,4.05269344373545));
#13785=CARTESIAN_POINT('Ctrl Pts',(12.3479491202706,10.4512882521917,4.18132152636351));
#13786=CARTESIAN_POINT('Ctrl Pts',(12.533545352339,10.5837092773919,4.30563832776911));
#13787=CARTESIAN_POINT('Ctrl Pts',(12.7188040406162,10.7153286091803,4.42955027592013));
#13788=CARTESIAN_POINT('Ctrl Pts',(12.9031225251803,10.8458735001829,4.55268038845334));
#13789=CARTESIAN_POINT('Ctrl Pts',(13.155473961026,11.0246032177407,4.72125849263582));
#13790=CARTESIAN_POINT('Ctrl Pts',(13.4103523866354,11.2042784469558,4.89121179563158));
#13791=CARTESIAN_POINT('Ctrl Pts',(13.6665968506704,11.3841414734491,5.0617474704863));
#13792=CARTESIAN_POINT('Ctrl Pts',(13.9194672603269,11.5616361848478,5.2300376465256));
#13793=CARTESIAN_POINT('Ctrl Pts',(14.1736679711043,11.7393134647389,5.3988950946096));
#13794=CARTESIAN_POINT('Ctrl Pts',(14.4280832903373,11.9164831860909,5.56759036901635));
#13795=CARTESIAN_POINT('Ctrl Pts',(14.6797373390571,12.0917300140853,5.73445472660428));
#13796=CARTESIAN_POINT('Ctrl Pts',(14.9316013630509,12.2664800265904,5.90116059552322));
#13797=CARTESIAN_POINT('Ctrl Pts',(15.1825956039735,12.440106754884,6.06703163030206));
#13798=CARTESIAN_POINT('Ctrl Pts',(15.3891870324201,12.5830175789843,6.20355880274597));
#13799=CARTESIAN_POINT('Ctrl Pts',(15.5951891994109,12.7251681216505,6.33952097663173));
#13800=CARTESIAN_POINT('Ctrl Pts',(15.8,12.8662316724636,6.47455487556026));
#13801=CARTESIAN_POINT('Origin',(15.8,0.,0.));
#13802=CARTESIAN_POINT('',(15.8,10.2357659846983,10.1335518448686));
#13803=CARTESIAN_POINT('Ctrl Pts',(10.0502525316942,7.53128682236137,5.21733945232202));
#13804=CARTESIAN_POINT('Ctrl Pts',(10.2399700857352,7.62691474601355,5.38300672530997));
#13805=CARTESIAN_POINT('Ctrl Pts',(10.4321639293634,7.72272706183511,5.55055481152831));
#13806=CARTESIAN_POINT('Ctrl Pts',(10.6261033397486,7.81846533797985,5.71924202232274));
#13807=CARTESIAN_POINT('Ctrl Pts',(10.8154947329249,7.91195848340778,5.8839733979618));
#13808=CARTESIAN_POINT('Ctrl Pts',(11.0065507832423,8.00538083967111,6.04979105175817));
#13809=CARTESIAN_POINT('Ctrl Pts',(11.1985909796536,8.09850566734924,6.21605213671094));
#13810=CARTESIAN_POINT('Ctrl Pts',(11.3896566244812,8.19115791194327,6.38146949203487));
#13811=CARTESIAN_POINT('Ctrl Pts',(11.5816964522015,8.28351537255324,6.54732580586867));
#13812=CARTESIAN_POINT('Ctrl Pts',(11.7740402595045,8.37537212829106,6.71303622283009));
#13813=CARTESIAN_POINT('Ctrl Pts',(11.9659830376819,8.46703736637644,6.87840114021681));
#13814=CARTESIAN_POINT('Ctrl Pts',(12.1582285291928,8.55820369955461,7.04362087245221));
#13815=CARTESIAN_POINT('Ctrl Pts',(12.3501107140342,8.64868803888447,7.20816146064368));
#13816=CARTESIAN_POINT('Ctrl Pts',(12.5349837899973,8.73586714908816,7.36669167899044));
#13817=CARTESIAN_POINT('Ctrl Pts',(12.7195196163976,8.82241309395647,7.52459184596092));
#13818=CARTESIAN_POINT('Ctrl Pts',(12.9031225251803,8.90818466253794,7.68142427504575));
#13819=CARTESIAN_POINT('Ctrl Pts',(13.0466099992771,8.97521598468133,7.80399035667839));
#13820=CARTESIAN_POINT('Ctrl Pts',(13.1909144693232,9.04240096834747,7.92707423833476));
#13821=CARTESIAN_POINT('Ctrl Pts',(13.3358225135832,9.10965124727546,8.05049252087456));
#13822=CARTESIAN_POINT('Ctrl Pts',(13.4722456635829,9.17296377720826,8.16668421304467));
#13823=CARTESIAN_POINT('Ctrl Pts',(13.6092037742271,9.23633418862365,8.2831723388735));
#13824=CARTESIAN_POINT('Ctrl Pts',(13.7465187613193,9.29969102606761,8.39980806233602));
#13825=CARTESIAN_POINT('Ctrl Pts',(13.8831227642785,9.36271981697347,8.51583987394238));
#13826=CARTESIAN_POINT('Ctrl Pts',(14.0200799576114,9.42573515876482,8.63201776215885));
#13827=CARTESIAN_POINT('Ctrl Pts',(14.1572150090555,9.48866882093701,8.74819853760654));
#13828=CARTESIAN_POINT('Ctrl Pts',(14.408874384546,9.6041596889012,8.9614042868683));
#13829=CARTESIAN_POINT('Ctrl Pts',(14.6611327271213,9.71937357878472,9.17461726587313));
#13830=CARTESIAN_POINT('Ctrl Pts',(14.9129064698064,9.83391026823084,9.38698186590772));
#13831=CARTESIAN_POINT('Ctrl Pts',(14.9348107204702,9.84387493066577,9.40545753132731));
#13832=CARTESIAN_POINT('Ctrl Pts',(14.9567113032193,9.85383448723492,9.42392680146367));
#13833=CARTESIAN_POINT('Ctrl Pts',(14.9786075045277,9.86378868594609,9.44238912780876));
#13834=CARTESIAN_POINT('Ctrl Pts',(15.1157365203996,9.92612869889287,9.55801286576868));
#13835=CARTESIAN_POINT('Ctrl Pts',(15.252693690801,9.98825831748494,9.67336395156666));
#13836=CARTESIAN_POINT('Ctrl Pts',(15.3893037522639,10.0501174002428,9.78830977806044));
#13837=CARTESIAN_POINT('Ctrl Pts',(15.4578478923357,10.0811552139138,9.84598388161831));
#13838=CARTESIAN_POINT('Ctrl Pts',(15.5263046465628,10.1121249718658,9.90355602888934));
#13839=CARTESIAN_POINT('Ctrl Pts',(15.5946518761319,10.1430193787867,9.96100982960575));
#13840=CARTESIAN_POINT('Ctrl Pts',(15.663218932117,10.1740131519407,10.0186484200082));
#13841=CARTESIAN_POINT('Ctrl Pts',(15.7316757577788,10.2049310789384,10.076167877539));
#13842=CARTESIAN_POINT('Ctrl Pts',(15.8,10.2357659846983,10.1335518448686));
#13843=CARTESIAN_POINT('Origin',(15.8,0.,0.));
#13844=CARTESIAN_POINT('',(15.8,6.60335220557564,12.8006061549939));
#13845=CARTESIAN_POINT('Ctrl Pts',(10.0502525316942,5.55043285230422,7.28928030147641));
#13846=CARTESIAN_POINT('Ctrl Pts',(10.2399762236018,5.59018769560149,7.47639594802589));
#13847=CARTESIAN_POINT('Ctrl Pts',(10.4321763653283,5.62953666502926,7.66535745978546));
#13848=CARTESIAN_POINT('Ctrl Pts',(10.6261221631187,5.66846318065085,7.85537951329531));
#13849=CARTESIAN_POINT('Ctrl Pts',(10.8155134734701,5.70647557321093,8.040939221832));
#13850=CARTESIAN_POINT('Ctrl Pts',(11.0065694150227,5.74408496164246,8.22751014665713));
#13851=CARTESIAN_POINT('Ctrl Pts',(11.198609478811,5.78127435838126,8.41441083753284));
#13852=CARTESIAN_POINT('Ctrl Pts',(11.3896744033045,5.81827491513847,8.60036248577492));
#13853=CARTESIAN_POINT('Ctrl Pts',(11.5817134810743,5.85485947501103,8.78664049259069));
#13854=CARTESIAN_POINT('Ctrl Pts',(11.7740565170522,5.89101292727613,8.97262500016317));
#13855=CARTESIAN_POINT('Ctrl Pts',(11.9659982062654,5.92709094103616,9.15822142880157));
#13856=CARTESIAN_POINT('Ctrl Pts',(12.1582425865198,5.96273934048968,9.34352559234053));
#13857=CARTESIAN_POINT('Ctrl Pts',(12.3501236493256,5.99794900016105,9.5279730968256));
#13858=CARTESIAN_POINT('Ctrl Pts',(12.5349923977936,6.03187191898508,9.7056799471712));
#13859=CARTESIAN_POINT('Ctrl Pts',(12.7195238985378,6.06538737998545,9.8825919457294));
#13860=CARTESIAN_POINT('Ctrl Pts',(12.9031225251803,6.0984963351851,10.0582492231335));
#13861=CARTESIAN_POINT('Ctrl Pts',(13.0466099992771,6.12437191191712,10.1955303101566));
#13862=CARTESIAN_POINT('Ctrl Pts',(13.1909144693232,6.15023362158894,10.3333513349338));
#13863=CARTESIAN_POINT('Ctrl Pts',(13.3358225135832,6.17605409599263,10.4715105676525));
#13864=CARTESIAN_POINT('Ctrl Pts',(13.4722456635829,6.20036268749026,10.6015800736297));
#13865=CARTESIAN_POINT('Ctrl Pts',(13.6092037742271,6.22463472522239,10.7319493881454));
#13866=CARTESIAN_POINT('Ctrl Pts',(13.7465187613193,6.24884824365306,10.8624548834565));
#13867=CARTESIAN_POINT('Ctrl Pts',(13.8831227642785,6.27293639028147,10.9922846525529));
#13868=CARTESIAN_POINT('Ctrl Pts',(14.0200799576114,6.29696660630781,11.1222491940658));
#13869=CARTESIAN_POINT('Ctrl Pts',(14.1572150090555,6.32091824773854,11.2521912379382));
#13870=CARTESIAN_POINT('Ctrl Pts',(14.4088957069953,6.36487612552845,11.4906707801789));
#13871=CARTESIAN_POINT('Ctrl Pts',(14.6611754735221,6.40856830116244,11.7290715847874));
#13872=CARTESIAN_POINT('Ctrl Pts',(14.912970466214,6.45187850892146,11.9664560266613));
#13873=CARTESIAN_POINT('Ctrl Pts',(14.9348533776006,6.45564249734868,11.9870865509245));
#13874=CARTESIAN_POINT('Ctrl Pts',(14.9567326275195,6.45940361158437,12.007709429508));
#13875=CARTESIAN_POINT('Ctrl Pts',(14.9786075045277,6.46316178167156,12.0283240646364));
#13876=CARTESIAN_POINT('Ctrl Pts',(15.1157365203996,6.48672096169998,12.1575528884896));
#13877=CARTESIAN_POINT('Ctrl Pts',(15.252693690801,6.5101642983752,12.2864573923713));
#13878=CARTESIAN_POINT('Ctrl Pts',(15.3893037522639,6.53347557107031,12.4148928744451));
#13879=CARTESIAN_POINT('Ctrl Pts',(15.4578478923357,6.54517200926641,12.4793354168112));
#13880=CARTESIAN_POINT('Ctrl Pts',(15.5263046465628,6.5568352285584,12.5436599631772));
#13881=CARTESIAN_POINT('Ctrl Pts',(15.5946518761319,6.56846335549623,12.6078486707221));
#13882=CARTESIAN_POINT('Ctrl Pts',(15.663218932117,6.58012888218654,12.6722438295541));
#13883=CARTESIAN_POINT('Ctrl Pts',(15.7316757577788,6.59175908863285,12.7365022490344));
#13884=CARTESIAN_POINT('Ctrl Pts',(15.8,6.60335220557564,12.8006061549939));
#13885=CARTESIAN_POINT('Origin',(15.8,0.,0.));
#13886=CARTESIAN_POINT('',(15.8,2.32455630431103,14.2146479476009));
#13887=CARTESIAN_POINT('Ctrl Pts',(10.0502525316942,3.02626384252387,8.64769560732005));
#13888=CARTESIAN_POINT('Ctrl Pts',(10.239953859285,3.00625338967616,8.83791565898891));
#13889=CARTESIAN_POINT('Ctrl Pts',(10.4321310528894,2.98528677263253,9.02976542249209));
#13890=CARTESIAN_POINT('Ctrl Pts',(10.6260535771563,2.96359080496254,9.22249314017983));
#13891=CARTESIAN_POINT('Ctrl Pts',(10.8154434277094,2.94240195085619,9.41071611112315));
#13892=CARTESIAN_POINT('Ctrl Pts',(11.0064979730127,2.9205173235086,9.5997763303737));
#13893=CARTESIAN_POINT('Ctrl Pts',(11.1985367155039,2.89813133617991,9.78902046263069));
#13894=CARTESIAN_POINT('Ctrl Pts',(11.3896029988914,2.87585870856653,9.97730628732497));
#13895=CARTESIAN_POINT('Ctrl Pts',(11.5816435370124,2.85308955972943,10.1657740234633));
#13896=CARTESIAN_POINT('Ctrl Pts',(11.7739881178962,2.83000106681665,10.353829469752));
#13897=CARTESIAN_POINT('Ctrl Pts',(11.9659332365641,2.80696052420482,10.5414943615216));
#13898=CARTESIAN_POINT('Ctrl Pts',(12.1581811364309,2.78360167031431,10.7287485903504));
#13899=CARTESIAN_POINT('Ctrl Pts',(12.3500657725588,2.76009024231686,10.9150525380981));
#13900=CARTESIAN_POINT('Ctrl Pts',(12.5349538836675,2.73743609136639,11.0945634446837));
#13901=CARTESIAN_POINT('Ctrl Pts',(12.7195047388313,2.71463999548723,11.2731923646037));
#13902=CARTESIAN_POINT('Ctrl Pts',(12.9031225251803,2.69184501333336,11.4505020946774));
#13903=CARTESIAN_POINT('Ctrl Pts',(13.0466099992771,2.67403195460754,11.5890601603578));
#13904=CARTESIAN_POINT('Ctrl Pts',(13.1909144693232,2.65603885317597,11.7281274609627));
#13905=CARTESIAN_POINT('Ctrl Pts',(13.3358225135832,2.63790201856914,11.8675036836248));
#13906=CARTESIAN_POINT('Ctrl Pts',(13.4722456635829,2.62082716174719,11.9987189203477));
#13907=CARTESIAN_POINT('Ctrl Pts',(13.6092037742272,2.60362489076148,12.1302080042448));
#13908=CARTESIAN_POINT('Ctrl Pts',(13.7465187613194,2.58632488288814,12.2618085151784));
#13909=CARTESIAN_POINT('Ctrl Pts',(13.8831227642785,2.56911445031434,12.3927276301685));
#13910=CARTESIAN_POINT('Ctrl Pts',(14.0200799576114,2.55180727580019,12.5237570157981));
#13911=CARTESIAN_POINT('Ctrl Pts',(14.1572150090555,2.53443232271127,12.6547407331994));
#13912=CARTESIAN_POINT('Ctrl Pts',(14.4088349682213,2.50255218017508,12.8950740198159));
#13913=CARTESIAN_POINT('Ctrl Pts',(14.6610537068593,2.47044377568191,13.1352504185273));
#13914=CARTESIAN_POINT('Ctrl Pts',(14.912788167058,2.4382861620121,13.374342879882));
#13915=CARTESIAN_POINT('Ctrl Pts',(14.9347318651876,2.43548298215988,13.3951845747094));
#13916=CARTESIAN_POINT('Ctrl Pts',(14.956671883473,2.43267942911465,13.4160180659855));
#13917=CARTESIAN_POINT('Ctrl Pts',(14.9786075045277,2.42987562206087,13.4368427586266));
#13918=CARTESIAN_POINT('Ctrl Pts',(15.1157365203996,2.4123478164419,13.5670268824575));
#13919=CARTESIAN_POINT('Ctrl Pts',(15.252693690801,2.39481006097156,13.6968667539964));
#13920=CARTESIAN_POINT('Ctrl Pts',(15.3893037522639,2.3772916450855,13.8262197421006));
#13921=CARTESIAN_POINT('Ctrl Pts',(15.4578478923357,2.368501774563,13.8911226433977));
#13922=CARTESIAN_POINT('Ctrl Pts',(15.5263046465628,2.35971677469615,13.9559030572658));
#13923=CARTESIAN_POINT('Ctrl Pts',(15.5946518761319,2.3509403772656,14.0205434363407));
#13924=CARTESIAN_POINT('Ctrl Pts',(15.663218932117,2.34213575215115,14.085391719422));
#13925=CARTESIAN_POINT('Ctrl Pts',(15.7316757577788,2.33333979124571,14.1500990399651));
#13926=CARTESIAN_POINT('Ctrl Pts',(15.8,2.32455630431103,14.2146479476009));
#13927=CARTESIAN_POINT('Origin',(15.8,0.,0.));
#13928=CARTESIAN_POINT('',(15.8,-2.18178336415567,14.2372609598209));
#13929=CARTESIAN_POINT('Ctrl Pts',(10.0502525316942,0.205863042617261,9.15961421508102));
#13930=CARTESIAN_POINT('Ctrl Pts',(10.2391570234259,0.128377591099419,9.33360673051063));
#13931=CARTESIAN_POINT('Ctrl Pts',(10.4305166252242,0.0494911083977331,
9.50884304477974));
#13932=CARTESIAN_POINT('Ctrl Pts',(10.6236099689119,-0.0303537569978928,
9.68468614630346));
#13933=CARTESIAN_POINT('Ctrl Pts',(10.8129280637648,-0.108637541989135,
9.85709126570178));
#13934=CARTESIAN_POINT('Ctrl Pts',(11.0039127690162,-0.187842691359053,
10.0300795089051));
#13935=CARTESIAN_POINT('Ctrl Pts',(11.195884205948,-0.267582809353856,10.2030901320277));
#13936=CARTESIAN_POINT('Ctrl Pts',(11.3869971487111,-0.34696633041216,10.3753270535338));
#13937=CARTESIAN_POINT('Ctrl Pts',(11.5790880175814,-0.426880221764492,
10.5475859558084));
#13938=CARTESIAN_POINT('Ctrl Pts',(11.771486014342,-0.50697211561905,10.7193560970325));
#13939=CARTESIAN_POINT('Ctrl Pts',(11.9635738218523,-0.586934883157645,
10.8908493057925));
#13940=CARTESIAN_POINT('Ctrl Pts',(12.1559677677314,-0.667075331863813,
11.0618551603495));
#13941=CARTESIAN_POINT('Ctrl Pts',(12.348000292972,-0.747068390651463,11.2319106356087));
#13942=CARTESIAN_POINT('Ctrl Pts',(12.5335794054258,-0.824373216142277,
11.3962512551313));
#13943=CARTESIAN_POINT('Ctrl Pts',(12.7188209807524,-0.901540748122868,
11.5597044367663));
#13944=CARTESIAN_POINT('Ctrl Pts',(12.9031225251803,-0.978296811887801,
11.7218943942307));
#13945=CARTESIAN_POINT('Ctrl Pts',(13.1554719876673,-1.08339279192325,11.943968217399));
#13946=CARTESIAN_POINT('Ctrl Pts',(13.4103484003965,-1.18950448019859,12.1673662092157));
#13947=CARTESIAN_POINT('Ctrl Pts',(13.6665908392654,-1.29611200619622,12.3911227672756));
#13948=CARTESIAN_POINT('Ctrl Pts',(13.9194596713268,-1.40131597126529,12.6119334173477));
#13949=CARTESIAN_POINT('Ctrl Pts',(14.1736587969731,-1.50700303047547,12.8330929959806));
#13950=CARTESIAN_POINT('Ctrl Pts',(14.4280725441414,-1.61269270111672,13.0537197620228));
#13951=CARTESIAN_POINT('Ctrl Pts',(14.6797279548927,-1.71723649158967,13.2719545077828));
#13952=CARTESIAN_POINT('Ctrl Pts',(14.9315933585705,-1.82178307810086,13.4896677845254));
#13953=CARTESIAN_POINT('Ctrl Pts',(15.1825889792205,-1.92588279206909,13.7060547738694));
#13954=CARTESIAN_POINT('Ctrl Pts',(15.3891826285153,-2.01156691573445,13.8841621753958));
#13955=CARTESIAN_POINT('Ctrl Pts',(15.5951870101931,-2.09694862236022,14.0613719009688));
#13956=CARTESIAN_POINT('Ctrl Pts',(15.8,-2.18178336415567,14.2372609598209));
#13957=CARTESIAN_POINT('Origin',(15.8,0.,0.));
#13958=CARTESIAN_POINT('',(15.8,-6.47455487556026,12.8662316724636));
#13959=CARTESIAN_POINT('Ctrl Pts',(10.0502525316942,-2.63468906623289,8.77492596468499));
#13960=CARTESIAN_POINT('Ctrl Pts',(10.2391461906128,-2.76214144474569,8.91645024269629));
#13961=CARTESIAN_POINT('Ctrl Pts',(10.4304946780274,-2.89131047500319,9.05872439496945));
#13962=CARTESIAN_POINT('Ctrl Pts',(10.6235767498551,-3.02157840065384,9.20127947078485));
#13963=CARTESIAN_POINT('Ctrl Pts',(10.8128907594452,-3.1493041034726,9.34105253585794));
#13964=CARTESIAN_POINT('Ctrl Pts',(11.0038713507036,-3.27808626456724,9.48109547783839));
#13965=CARTESIAN_POINT('Ctrl Pts',(11.1958386868241,-3.40738413972981,9.620994430446));
#13966=CARTESIAN_POINT('Ctrl Pts',(11.3869496174047,-3.53610519063243,9.76026926521946));
#13967=CARTESIAN_POINT('Ctrl Pts',(11.5790385083446,-3.66533747024595,9.89940114828162));
#13968=CARTESIAN_POINT('Ctrl Pts',(11.77143458098,-3.79458803732591,10.0380132338097));
#13969=CARTESIAN_POINT('Ctrl Pts',(11.9635224158189,-3.92363153203981,10.1764032488807));
#13970=CARTESIAN_POINT('Ctrl Pts',(12.15591644887,-4.05269344373575,10.3142748929473));
#13971=CARTESIAN_POINT('Ctrl Pts',(12.3479491202708,-4.18132152636367,10.4512882521919));
#13972=CARTESIAN_POINT('Ctrl Pts',(12.5335453523391,-4.30563832776922,10.583709277392));
#13973=CARTESIAN_POINT('Ctrl Pts',(12.7188040406163,-4.42955027592018,10.7153286091803));
#13974=CARTESIAN_POINT('Ctrl Pts',(12.9031225251803,-4.55268038845334,10.8458735001828));
#13975=CARTESIAN_POINT('Ctrl Pts',(13.1554739610255,-4.72125849263545,11.0246032177403));
#13976=CARTESIAN_POINT('Ctrl Pts',(13.4103523866342,-4.89121179563083,11.204278446955));
#13977=CARTESIAN_POINT('Ctrl Pts',(13.6665968506687,-5.06174747048518,11.3841414734479));
#13978=CARTESIAN_POINT('Ctrl Pts',(13.919467260325,-5.23003764652437,11.5616361848466));
#13979=CARTESIAN_POINT('Ctrl Pts',(14.1736679711023,-5.39889509460827,11.7393134647375));
#13980=CARTESIAN_POINT('Ctrl Pts',(14.4280832903352,-5.56759036901493,11.9164831860894));
#13981=CARTESIAN_POINT('Ctrl Pts',(14.6797373390547,-5.7344547266027,12.0917300140837));
#13982=CARTESIAN_POINT('Ctrl Pts',(14.9316013630483,-5.90116059552149,12.2664800265886));
#13983=CARTESIAN_POINT('Ctrl Pts',(15.1825956039707,-6.06703163030022,12.4401067548821));
#13984=CARTESIAN_POINT('Ctrl Pts',(15.3891870324182,-6.20355880274473,12.583017578983));
#13985=CARTESIAN_POINT('Ctrl Pts',(15.59518919941,-6.3395209766311,12.7251681216498));
#13986=CARTESIAN_POINT('Ctrl Pts',(15.8,-6.47455487556026,12.8662316724636));
#13987=CARTESIAN_POINT('Origin',(15.8,0.,0.));
#13988=CARTESIAN_POINT('',(15.8,-10.1335518448686,10.2357659846983));
#13989=CARTESIAN_POINT('Ctrl Pts',(10.0502525316942,-5.21733945232202,7.53128682236137));
#13990=CARTESIAN_POINT('Ctrl Pts',(10.2399700857352,-5.38300672530999,7.62691474601356));
#13991=CARTESIAN_POINT('Ctrl Pts',(10.4321639293634,-5.55055481152835,7.72272706183513));
#13992=CARTESIAN_POINT('Ctrl Pts',(10.6261033397487,-5.71924202232279,7.81846533797988));
#13993=CARTESIAN_POINT('Ctrl Pts',(10.815494732925,-5.88397339796186,7.91195848340782));
#13994=CARTESIAN_POINT('Ctrl Pts',(11.0065507832424,-6.04979105175824,8.00538083967115));
#13995=CARTESIAN_POINT('Ctrl Pts',(11.1985909796537,-6.21605213671102,8.09850566734929));
#13996=CARTESIAN_POINT('Ctrl Pts',(11.3896566244815,-6.38146949203515,8.19115791194343));
#13997=CARTESIAN_POINT('Ctrl Pts',(11.5816964522021,-6.54732580586915,8.2835153725535));
#13998=CARTESIAN_POINT('Ctrl Pts',(11.7740402595053,-6.71303622283077,8.37537212829144));
#13999=CARTESIAN_POINT('Ctrl Pts',(11.9659830376826,-6.87840114021745,8.4670373663768));
#14000=CARTESIAN_POINT('Ctrl Pts',(12.1582285291935,-7.0436208724528,8.55820369955494));
#14001=CARTESIAN_POINT('Ctrl Pts',(12.3501107140348,-7.20816146064422,8.64868803888477));
#14002=CARTESIAN_POINT('Ctrl Pts',(12.5349837899977,-7.3666916789908,8.73586714908836));
#14003=CARTESIAN_POINT('Ctrl Pts',(12.7195196163979,-7.5245918459611,8.82241309395657));
#14004=CARTESIAN_POINT('Ctrl Pts',(12.9031225251803,-7.68142427504574,8.90818466253794));
#14005=CARTESIAN_POINT('Ctrl Pts',(13.0466099992771,-7.80399035667839,8.97521598468134));
#14006=CARTESIAN_POINT('Ctrl Pts',(13.1909144693232,-7.92707423833475,9.04240096834747));
#14007=CARTESIAN_POINT('Ctrl Pts',(13.3358225135832,-8.05049252087456,9.10965124727546));
#14008=CARTESIAN_POINT('Ctrl Pts',(13.4722456635829,-8.16668421304467,9.17296377720826));
#14009=CARTESIAN_POINT('Ctrl Pts',(13.6092037742271,-8.2831723388735,9.23633418862365));
#14010=CARTESIAN_POINT('Ctrl Pts',(13.7465187613193,-8.39980806233602,9.29969102606761));
#14011=CARTESIAN_POINT('Ctrl Pts',(13.8831227642785,-8.51583987394238,9.36271981697347));
#14012=CARTESIAN_POINT('Ctrl Pts',(14.0200799576114,-8.63201776215885,9.42573515876482));
#14013=CARTESIAN_POINT('Ctrl Pts',(14.1572150090555,-8.74819853760654,9.48866882093701));
#14014=CARTESIAN_POINT('Ctrl Pts',(14.4088743845451,-8.96140428686748,9.60415968890076));
#14015=CARTESIAN_POINT('Ctrl Pts',(14.6611327271194,-9.17461726587151,9.71937357878384));
#14016=CARTESIAN_POINT('Ctrl Pts',(14.9129064698035,-9.38698186590529,9.83391026822953));
#14017=CARTESIAN_POINT('Ctrl Pts',(14.9348107204683,-9.40545753132569,9.8438749306649));
#14018=CARTESIAN_POINT('Ctrl Pts',(14.9567113032183,-9.42392680146286,9.85383448723449));
#14019=CARTESIAN_POINT('Ctrl Pts',(14.9786075045277,-9.44238912780876,9.86378868594609));
#14020=CARTESIAN_POINT('Ctrl Pts',(15.1157365203996,-9.55801286576868,9.92612869889287));
#14021=CARTESIAN_POINT('Ctrl Pts',(15.252693690801,-9.67336395156666,9.98825831748495));
#14022=CARTESIAN_POINT('Ctrl Pts',(15.3893037522639,-9.78830977806044,10.0501174002428));
#14023=CARTESIAN_POINT('Ctrl Pts',(15.4578478923357,-9.84598388161831,10.0811552139138));
#14024=CARTESIAN_POINT('Ctrl Pts',(15.5263046465628,-9.90355602888934,10.1121249718658));
#14025=CARTESIAN_POINT('Ctrl Pts',(15.5946518761319,-9.96100982960575,10.1430193787867));
#14026=CARTESIAN_POINT('Ctrl Pts',(15.663218932117,-10.0186484200082,10.1740131519407));
#14027=CARTESIAN_POINT('Ctrl Pts',(15.7316757577788,-10.076167877539,10.2049310789385));
#14028=CARTESIAN_POINT('Ctrl Pts',(15.8,-10.1335518448686,10.2357659846983));
#14029=CARTESIAN_POINT('Origin',(15.8,0.,0.));
#14030=CARTESIAN_POINT('',(15.8,-12.8006061549939,6.60335220557564));
#14031=CARTESIAN_POINT('Ctrl Pts',(10.0502525316942,-7.28928030147641,5.55043285230422));
#14032=CARTESIAN_POINT('Ctrl Pts',(10.2399762236017,-7.47639594802579,5.59018769560147));
#14033=CARTESIAN_POINT('Ctrl Pts',(10.4321763653281,-7.66535745978524,5.62953666502922));
#14034=CARTESIAN_POINT('Ctrl Pts',(10.6261221631183,-7.85537951329499,5.66846318065078));
#14035=CARTESIAN_POINT('Ctrl Pts',(10.8155134734698,-8.04093922183172,5.70647557321088));
#14036=CARTESIAN_POINT('Ctrl Pts',(11.0065694150225,-8.2275101466569,5.74408496164242));
#14037=CARTESIAN_POINT('Ctrl Pts',(11.1986094788108,-8.41441083753267,5.78127435838123));
#14038=CARTESIAN_POINT('Ctrl Pts',(11.3896744033043,-8.60036248577474,5.81827491513844));
#14039=CARTESIAN_POINT('Ctrl Pts',(11.5817134810741,-8.78664049259051,5.854859475011));
#14040=CARTESIAN_POINT('Ctrl Pts',(11.774056517052,-8.972625000163,5.89101292727611));
#14041=CARTESIAN_POINT('Ctrl Pts',(11.9659982062652,-9.15822142880141,5.92709094103613));
#14042=CARTESIAN_POINT('Ctrl Pts',(12.1582425865196,-9.3435255923404,5.96273934048966));
#14043=CARTESIAN_POINT('Ctrl Pts',(12.3501236493256,-9.52797309682552,5.99794900016104));
#14044=CARTESIAN_POINT('Ctrl Pts',(12.5349923977935,-9.70567994717112,6.03187191898507));
#14045=CARTESIAN_POINT('Ctrl Pts',(12.7195238985377,-9.88259194572935,6.06538737998544));
#14046=CARTESIAN_POINT('Ctrl Pts',(12.9031225251803,-10.0582492231335,6.0984963351851));
#14047=CARTESIAN_POINT('Ctrl Pts',(13.0466099992771,-10.1955303101566,6.12437191191712));
#14048=CARTESIAN_POINT('Ctrl Pts',(13.1909144693232,-10.3333513349338,6.15023362158894));
#14049=CARTESIAN_POINT('Ctrl Pts',(13.3358225135832,-10.4715105676525,6.17605409599263));
#14050=CARTESIAN_POINT('Ctrl Pts',(13.4722456635829,-10.6015800736297,6.20036268749026));
#14051=CARTESIAN_POINT('Ctrl Pts',(13.6092037742271,-10.7319493881454,6.22463472522239));
#14052=CARTESIAN_POINT('Ctrl Pts',(13.7465187613193,-10.8624548834565,6.24884824365307));
#14053=CARTESIAN_POINT('Ctrl Pts',(13.8831227642785,-10.9922846525529,6.27293639028148));
#14054=CARTESIAN_POINT('Ctrl Pts',(14.0200799576114,-11.1222491940658,6.29696660630782));
#14055=CARTESIAN_POINT('Ctrl Pts',(14.1572150090555,-11.2521912379382,6.32091824773854));
#14056=CARTESIAN_POINT('Ctrl Pts',(14.4088957069996,-11.4906707801829,6.36487612552919));
#14057=CARTESIAN_POINT('Ctrl Pts',(14.6611754735305,-11.7290715847954,6.40856830116391));
#14058=CARTESIAN_POINT('Ctrl Pts',(14.9129704662266,-11.9664560266731,6.45187850892362));
#14059=CARTESIAN_POINT('Ctrl Pts',(14.9348533776089,-11.9870865509323,6.45564249735012));
#14060=CARTESIAN_POINT('Ctrl Pts',(14.9567326275237,-12.007709429512,6.45940361158509));
#14061=CARTESIAN_POINT('Ctrl Pts',(14.9786075045277,-12.0283240646364,6.46316178167156));
#14062=CARTESIAN_POINT('Ctrl Pts',(15.1157365203997,-12.1575528884896,6.48672096169998));
#14063=CARTESIAN_POINT('Ctrl Pts',(15.252693690801,-12.2864573923713,6.5101642983752));
#14064=CARTESIAN_POINT('Ctrl Pts',(15.3893037522639,-12.4148928744451,6.53347557107031));
#14065=CARTESIAN_POINT('Ctrl Pts',(15.4578478923357,-12.4793354168112,6.54517200926641));
#14066=CARTESIAN_POINT('Ctrl Pts',(15.5263046465628,-12.5436599631772,6.5568352285584));
#14067=CARTESIAN_POINT('Ctrl Pts',(15.5946518761319,-12.6078486707221,6.56846335549623));
#14068=CARTESIAN_POINT('Ctrl Pts',(15.663218932117,-12.6722438295541,6.58012888218654));
#14069=CARTESIAN_POINT('Ctrl Pts',(15.7316757577788,-12.7365022490344,6.59175908863286));
#14070=CARTESIAN_POINT('Ctrl Pts',(15.8,-12.8006061549939,6.60335220557564));
#14071=CARTESIAN_POINT('Origin',(15.8,0.,0.));
#14072=CARTESIAN_POINT('',(15.8,-14.2146479476009,2.32455630431103));
#14073=CARTESIAN_POINT('Ctrl Pts',(10.0502525316942,-8.64769560732005,3.02626384252387));
#14074=CARTESIAN_POINT('Ctrl Pts',(10.2399538592853,-8.83791565898925,3.00625338967612));
#14075=CARTESIAN_POINT('Ctrl Pts',(10.43213105289,-9.02976542249276,2.98528677263246));
#14076=CARTESIAN_POINT('Ctrl Pts',(10.6260535771573,-9.22249314018085,2.96359080496243));
#14077=CARTESIAN_POINT('Ctrl Pts',(10.8154434277105,-9.41071611112417,2.94240195085607));
#14078=CARTESIAN_POINT('Ctrl Pts',(11.0064979730137,-9.59977633037473,2.92051732350848));
#14079=CARTESIAN_POINT('Ctrl Pts',(11.198536715505,-9.78902046263172,2.89813133617979));
#14080=CARTESIAN_POINT('Ctrl Pts',(11.3896029988924,-9.97730628732604,2.8758587085664));
#14081=CARTESIAN_POINT('Ctrl Pts',(11.5816435370135,-10.1657740234644,2.85308955972929));
#14082=CARTESIAN_POINT('Ctrl Pts',(11.7739881178974,-10.3538294697532,2.8300010668165));
#14083=CARTESIAN_POINT('Ctrl Pts',(11.9659332365655,-10.5414943615229,2.80696052420466));
#14084=CARTESIAN_POINT('Ctrl Pts',(12.1581811364325,-10.7287485903519,2.78360167031412));
#14085=CARTESIAN_POINT('Ctrl Pts',(12.3500657725605,-10.9150525380997,2.76009024231665));
#14086=CARTESIAN_POINT('Ctrl Pts',(12.5349538836687,-11.0945634446848,2.73743609136625));
#14087=CARTESIAN_POINT('Ctrl Pts',(12.7195047388318,-11.2731923646042,2.71463999548716));
#14088=CARTESIAN_POINT('Ctrl Pts',(12.9031225251803,-11.4505020946774,2.69184501333336));
#14089=CARTESIAN_POINT('Ctrl Pts',(13.0466099992771,-11.5890601603578,2.67403195460754));
#14090=CARTESIAN_POINT('Ctrl Pts',(13.1909144693232,-11.7281274609627,2.65603885317597));
#14091=CARTESIAN_POINT('Ctrl Pts',(13.3358225135832,-11.8675036836248,2.63790201856914));
#14092=CARTESIAN_POINT('Ctrl Pts',(13.4722456635829,-11.9987189203477,2.62082716174719));
#14093=CARTESIAN_POINT('Ctrl Pts',(13.6092037742271,-12.1302080042448,2.60362489076148));
#14094=CARTESIAN_POINT('Ctrl Pts',(13.7465187613193,-12.2618085151784,2.58632488288814));
#14095=CARTESIAN_POINT('Ctrl Pts',(13.8831227642785,-12.3927276301685,2.56911445031434));
#14096=CARTESIAN_POINT('Ctrl Pts',(14.0200799576114,-12.5237570157981,2.55180727580019));
#14097=CARTESIAN_POINT('Ctrl Pts',(14.1572150090555,-12.6547407331994,2.53443232271127));
#14098=CARTESIAN_POINT('Ctrl Pts',(14.4088349682203,-12.895074019815,2.5025521801752));
#14099=CARTESIAN_POINT('Ctrl Pts',(14.6610537068573,-13.1352504185255,2.47044377568216));
#14100=CARTESIAN_POINT('Ctrl Pts',(14.912788167055,-13.3743428798791,2.43828616201247));
#14101=CARTESIAN_POINT('Ctrl Pts',(14.9347318651856,-13.3951845747076,2.43548298216013));
#14102=CARTESIAN_POINT('Ctrl Pts',(14.956671883472,-13.4160180659846,2.43267942911478));
#14103=CARTESIAN_POINT('Ctrl Pts',(14.9786075045277,-13.4368427586266,2.42987562206087));
#14104=CARTESIAN_POINT('Ctrl Pts',(15.1157365203996,-13.5670268824575,2.4123478164419));
#14105=CARTESIAN_POINT('Ctrl Pts',(15.252693690801,-13.6968667539964,2.39481006097156));
#14106=CARTESIAN_POINT('Ctrl Pts',(15.3893037522639,-13.8262197421006,2.3772916450855));
#14107=CARTESIAN_POINT('Ctrl Pts',(15.4578478923357,-13.8911226433977,2.368501774563));
#14108=CARTESIAN_POINT('Ctrl Pts',(15.5263046465628,-13.9559030572657,2.35971677469615));
#14109=CARTESIAN_POINT('Ctrl Pts',(15.5946518761319,-14.0205434363407,2.3509403772656));
#14110=CARTESIAN_POINT('Ctrl Pts',(15.663218932117,-14.085391719422,2.34213575215115));
#14111=CARTESIAN_POINT('Ctrl Pts',(15.7316757577788,-14.1500990399651,2.33333979124571));
#14112=CARTESIAN_POINT('Ctrl Pts',(15.8,-14.2146479476009,2.32455630431103));
#14113=CARTESIAN_POINT('Origin',(15.8,0.,0.));
#14114=CARTESIAN_POINT('Ctrl Pts',(10.0502525316942,9.2755658561365,-5.45537535466284));
#14115=CARTESIAN_POINT('Ctrl Pts',(11.1454425256572,10.527811485966,-5.54272139501844));
#14116=CARTESIAN_POINT('Ctrl Pts',(12.3775312688656,11.9365878195243,-5.64098569041847));
#14117=CARTESIAN_POINT('Ctrl Pts',(13.7465187613193,13.5018948568112,-5.75016824086296));
#14118=CARTESIAN_POINT('Ctrl Pts',(14.2941137583009,14.1280176717259,-5.79384126104075));
#14119=CARTESIAN_POINT('Ctrl Pts',(14.8417087552824,14.7541404866407,-5.83751428121855));
#14120=CARTESIAN_POINT('Ctrl Pts',(15.3208543776412,15.3019979496911,-5.87572817387412));
#14121=CARTESIAN_POINT('Ctrl Pts',(15.5946518761319,15.6150593571485,-5.89756468396302));
#14122=CARTESIAN_POINT('Ctrl Pts',(15.7315506253773,15.7715900608772,-5.90848293900747));
#14123=CARTESIAN_POINT('Ctrl Pts',(15.8,15.8498554127416,-5.91394206652969));
#14124=CARTESIAN_POINT('Ctrl Pts',(10.0502525316942,9.09326359699885,-5.66046875858054));
#14125=CARTESIAN_POINT('Ctrl Pts',(11.1454425256572,10.3398594101876,-5.77604676609018));
#14126=CARTESIAN_POINT('Ctrl Pts',(12.3775312688656,11.7423187718539,-5.90654052031257));
#14127=CARTESIAN_POINT('Ctrl Pts',(13.7465187613193,13.3005670731329,-6.05105541408884));
#14128=CARTESIAN_POINT('Ctrl Pts',(14.2941137583009,13.9238668895967,-6.10886731837785));
#14129=CARTESIAN_POINT('Ctrl Pts',(14.8417087552824,14.5471710567224,-6.16673138983645));
#14130=CARTESIAN_POINT('Ctrl Pts',(15.3208543776412,15.0925608480023,-6.21734620559882));
#14131=CARTESIAN_POINT('Ctrl Pts',(15.5946518761319,15.4042104768461,-6.24624880770452));
#14132=CARTESIAN_POINT('Ctrl Pts',(15.7315506253773,15.5600357233504,-6.26070528969669));
#14133=CARTESIAN_POINT('Ctrl Pts',(15.8,15.6379479616747,-6.26792891516604));
#14134=CARTESIAN_POINT('Ctrl Pts',(10.0502525316942,8.78255765938311,-5.94355560685308));
#14135=CARTESIAN_POINT('Ctrl Pts',(11.1454425256572,10.0148869038525,-6.10292787924083));
#14136=CARTESIAN_POINT('Ctrl Pts',(12.3775312688656,11.4012092316412,-6.28165449494742));
#14137=CARTESIAN_POINT('Ctrl Pts',(13.7465187613194,12.9416164381759,-6.48081852219946));
#14138=CARTESIAN_POINT('Ctrl Pts',(14.2941137583009,13.5577787105922,-6.56047693355266));
#14139=CARTESIAN_POINT('Ctrl Pts',(14.8417087552824,14.1739356301478,-6.64007218801817));
#14140=CARTESIAN_POINT('Ctrl Pts',(15.3208543776412,14.7130746018355,-6.70973770503941));
#14141=CARTESIAN_POINT('Ctrl Pts',(15.594651876132,15.0211560817903,-6.74957096648569));
#14142=CARTESIAN_POINT('Ctrl Pts',(15.7315506253773,15.1751962901528,-6.76948132483474));
#14143=CARTESIAN_POINT('Ctrl Pts',(15.8,15.2522168679322,-6.77944209185897));
#14144=CARTESIAN_POINT('Ctrl Pts',(10.0502525316942,8.52639512605652,-5.98584659003549));
#14145=CARTESIAN_POINT('Ctrl Pts',(11.1454425256572,9.73363772297167,-6.16614182963237));
#14146=CARTESIAN_POINT('Ctrl Pts',(12.3775312688656,11.0917875706281,-6.36925721416675));
#14147=CARTESIAN_POINT('Ctrl Pts',(13.7465187613193,12.6008409910269,-6.59465188812855));
#14148=CARTESIAN_POINT('Ctrl Pts',(14.2941137583008,13.2044623836355,-6.68481335297615));
#14149=CARTESIAN_POINT('Ctrl Pts',(14.8417087552823,13.8080839907189,-6.77500635669625));
#14150=CARTESIAN_POINT('Ctrl Pts',(15.3208543776412,14.3362528301216,-6.85391541259335));
#14151=CARTESIAN_POINT('Ctrl Pts',(15.5946518761319,14.6380635126529,-6.89899411967348));
#14152=CARTESIAN_POINT('Ctrl Pts',(15.7315506253773,14.7889688752189,-6.9215366054706));
#14153=CARTESIAN_POINT('Ctrl Pts',(15.8,14.8644215375261,-6.9328050579454));
#14154=CARTESIAN_POINT('Ctrl Pts',(10.0502525316942,8.35233000922534,-5.94770436886829));
#14155=CARTESIAN_POINT('Ctrl Pts',(11.1454425256572,9.5384055936255,-6.13452948592057));
#14156=CARTESIAN_POINT('Ctrl Pts',(12.3775312688656,10.8728200811769,-6.34492663085593));
#14157=CARTESIAN_POINT('Ctrl Pts',(13.7465187613193,12.3554217499083,-6.57847782979355));
#14158=CARTESIAN_POINT('Ctrl Pts',(14.2941137583008,12.9484634259519,-6.67190108779269));
#14159=CARTESIAN_POINT('Ctrl Pts',(14.8417087552824,13.541513949349,-6.7653487190758));
#14160=CARTESIAN_POINT('Ctrl Pts',(15.3208543776412,14.0604304019321,-6.84710780571678));
#14161=CARTESIAN_POINT('Ctrl Pts',(15.5946518761319,14.3569506718,-6.89381786952799));
#14162=CARTESIAN_POINT('Ctrl Pts',(15.7315506253773,14.5052116854016,-6.91717532204614));
#14163=CARTESIAN_POINT('Ctrl Pts',(15.8,14.5793414094266,-6.92885189186191));
#14164=CARTESIAN_POINT('Ctrl Pts',(10.0502525316942,8.1751443698686,-5.91814205125966));
#14165=CARTESIAN_POINT('Ctrl Pts',(11.1454425256572,9.34066488658195,-6.11093026523681));
#14166=CARTESIAN_POINT('Ctrl Pts',(12.3775312688656,10.6518240329443,-6.32804641946555));
#14167=CARTESIAN_POINT('Ctrl Pts',(13.7465187613193,12.1087200255634,-6.56905244176937));
#14168=CARTESIAN_POINT('Ctrl Pts',(14.2941137583008,12.6914777697296,-6.66545776271566));
#14169=CARTESIAN_POINT('Ctrl Pts',(14.8417087552823,13.2742297865971,-6.76188862893654));
#14170=CARTESIAN_POINT('Ctrl Pts',(15.3208543776412,13.7841395850464,-6.84625768114734));
#14171=CARTESIAN_POINT('Ctrl Pts',(15.5946518761319,14.0755188249216,-6.89445870116996));
#14172=CARTESIAN_POINT('Ctrl Pts',(15.7315506253773,14.2212078760573,-6.91856174818909));
#14173=CARTESIAN_POINT('Ctrl Pts',(15.8,14.2940529083518,-6.93061101156266));
#14174=CARTESIAN_POINT('Ctrl Pts',(10.0502525316942,7.90144264462466,-5.89433124999989));
#14175=CARTESIAN_POINT('Ctrl Pts',(11.1454425256572,9.03654403267794,-6.09882926548583));
#14176=CARTESIAN_POINT('Ctrl Pts',(12.3775312688656,10.3136205759385,-6.32895925304844));
#14177=CARTESIAN_POINT('Ctrl Pts',(13.7465187613193,11.7325052253954,-6.58458807992399));
#14178=CARTESIAN_POINT('Ctrl Pts',(14.2941137583008,12.3000601956136,-6.68684049565602));
#14179=CARTESIAN_POINT('Ctrl Pts',(14.8417087552823,12.86762490695,-6.78910067475031));
#14180=CARTESIAN_POINT('Ctrl Pts',(15.3208543776411,13.364240995629,-6.87857591366297));
#14181=CARTESIAN_POINT('Ctrl Pts',(15.5946518761319,13.6480178551891,-6.92970162298622));
#14182=CARTESIAN_POINT('Ctrl Pts',(15.7315506253773,13.7899072524002,-6.95526524865976));
#14183=CARTESIAN_POINT('Ctrl Pts',(15.8,13.8608510891535,-6.96804637462763));
#14184=CARTESIAN_POINT('Ctrl Pts',(10.0502525316942,7.66237562613099,-5.80163007173557));
#14185=CARTESIAN_POINT('Ctrl Pts',(11.1454425256572,8.76621669669801,-6.00977287125004));
#14186=CARTESIAN_POINT('Ctrl Pts',(12.3775312688656,10.008064757174,-6.24400287259235));
#14187=CARTESIAN_POINT('Ctrl Pts',(13.7465187613193,11.3878685250288,-6.50418764618811));
#14188=CARTESIAN_POINT('Ctrl Pts',(14.2941137583008,11.9397903730643,-6.60826243593386));
#14189=CARTESIAN_POINT('Ctrl Pts',(14.8417087552823,12.4917152115347,-6.71234494803684));
#14190=CARTESIAN_POINT('Ctrl Pts',(15.3208543776411,12.9746485138656,-6.80341474110257));
#14191=CARTESIAN_POINT('Ctrl Pts',(15.5946518761319,13.2506092458454,-6.85545164006593));
#14192=CARTESIAN_POINT('Ctrl Pts',(15.7315506253773,13.388589908828,-6.88147085648712));
#14193=CARTESIAN_POINT('Ctrl Pts',(15.8,13.4575799757384,-6.89447978145678));
#14194=CARTESIAN_POINT('Ctrl Pts',(10.0502525316942,7.44593237535689,-5.68351040711503));
#14195=CARTESIAN_POINT('Ctrl Pts',(11.1454425256572,8.51992624992032,-5.89012315163303));
#14196=CARTESIAN_POINT('Ctrl Pts',(12.3775312688656,9.72815762348205,-6.12263633930509));
#14197=CARTESIAN_POINT('Ctrl Pts',(13.7465187613194,11.0706489050023,-6.38090895110342));
#14198=CARTESIAN_POINT('Ctrl Pts',(14.2941137583009,11.60764526865,-6.48421893322741));
#14199=CARTESIAN_POINT('Ctrl Pts',(14.8417087552824,12.1446403255654,-6.58753713858488));
#14200=CARTESIAN_POINT('Ctrl Pts',(15.3208543776412,12.6145114073305,-6.67793800725711));
#14201=CARTESIAN_POINT('Ctrl Pts',(15.594651876132,12.8830096730692,-6.72959247024462));
#14202=CARTESIAN_POINT('Ctrl Pts',(15.7315506253773,13.0172586761616,-6.75542051842202));
#14203=CARTESIAN_POINT('Ctrl Pts',(15.8,13.0843832933218,-6.76833381495439));
#14204=CARTESIAN_POINT('Ctrl Pts',(10.0502525316942,7.34913449516209,-5.60747221894231));
#14205=CARTESIAN_POINT('Ctrl Pts',(11.1454425256572,8.40845336995523,-5.81105284226644));
#14206=CARTESIAN_POINT('Ctrl Pts',(12.3775312688656,9.60029668798142,-6.04008639989119));
#14207=CARTESIAN_POINT('Ctrl Pts',(13.7465187613193,10.9244551954278,-6.29456266363367));
#14208=CARTESIAN_POINT('Ctrl Pts',(14.2941137583009,11.4541199893924,-6.39635323712111));
#14209=CARTESIAN_POINT('Ctrl Pts',(14.8417087552824,11.9837969855611,-6.49814440704392));
#14210=CARTESIAN_POINT('Ctrl Pts',(15.3208543776412,12.4472605569962,-6.58721149497459));
#14211=CARTESIAN_POINT('Ctrl Pts',(15.5946518761319,12.7120921703849,-6.6381067434168));
#14212=CARTESIAN_POINT('Ctrl Pts',(15.7315506253773,12.8445091889311,-6.66355442687239));
#14213=CARTESIAN_POINT('Ctrl Pts',(15.8,12.9107166186057,-6.67627821583014));
#14214=CARTESIAN_POINT('Ctrl Pts',(10.0502525316942,7.28928030147641,-5.55043285230422));
#14215=CARTESIAN_POINT('Ctrl Pts',(11.1454425256572,8.33905665452735,-5.75098891959401));
#14216=CARTESIAN_POINT('Ctrl Pts',(12.3775312688656,9.52005505170966,-5.97661449529503));
#14217=CARTESIAN_POINT('Ctrl Pts',(13.7465187613193,10.8322754930233,-6.22730957940728));
#14218=CARTESIAN_POINT('Ctrl Pts',(14.2941137583009,11.3571636695488,-6.32758761305217));
#14219=CARTESIAN_POINT('Ctrl Pts',(14.8417087552824,11.8820518460743,-6.42786564669707));
#14220=CARTESIAN_POINT('Ctrl Pts',(15.3208543776412,12.3413290005341,-6.51560892613635));
#14221=CARTESIAN_POINT('Ctrl Pts',(15.5946518761319,12.6037730887968,-6.56574794295881));
#14222=CARTESIAN_POINT('Ctrl Pts',(15.7315506253773,12.7349951329282,-6.59081745137003));
#14223=CARTESIAN_POINT('Ctrl Pts',(15.8,12.8006061549939,-6.60335220557564));
#14224=CARTESIAN_POINT('Ctrl Pts',(15.8,12.8370600702028,-6.62691983743441));
#14225=CARTESIAN_POINT('Ctrl Pts',(15.8,12.8297280642598,-6.62229417791417));
#14226=CARTESIAN_POINT('Ctrl Pts',(15.8,12.8224166748639,-6.61762457479065));
#14227=CARTESIAN_POINT('Ctrl Pts',(15.8,12.8151258955788,-6.6129110406524));
#14228=CARTESIAN_POINT('Ctrl Pts',(15.8,12.8078557223109,-6.60815358414732));
#14229=CARTESIAN_POINT('Ctrl Pts',(15.8,12.8006061549939,-6.60335220557564));
#14230=CARTESIAN_POINT('Origin',(15.8,13.950492764499,-5.67212567669951));
#14231=CARTESIAN_POINT('Ctrl Pts',(10.0502525316942,7.13578365451837,-8.05467776187827));
#14232=CARTESIAN_POINT('Ctrl Pts',(11.1454425256572,8.29974860990864,-8.52471396348012));
#14233=CARTESIAN_POINT('Ctrl Pts',(12.3775312688656,9.6092091847227,-9.05350469028219));
#14234=CARTESIAN_POINT('Ctrl Pts',(13.7465187613193,11.0641653789605,-9.6410499422845));
#14235=CARTESIAN_POINT('Ctrl Pts',(14.2941137583009,11.6461478566557,-9.87606804308543));
#14236=CARTESIAN_POINT('Ctrl Pts',(14.8417087552824,12.2281303343508,-10.1110861438864));
#14237=CARTESIAN_POINT('Ctrl Pts',(15.3208543776412,12.737365002334,-10.3167269820872));
#14238=CARTESIAN_POINT('Ctrl Pts',(15.5946518761319,13.0283562411816,-10.4342360324876));
#14239=CARTESIAN_POINT('Ctrl Pts',(15.7315506253773,13.1738518606054,-10.4929905576879));
#14240=CARTESIAN_POINT('Ctrl Pts',(15.8,13.2465996703173,-10.522367820288));
#14241=CARTESIAN_POINT('Ctrl Pts',(10.0502525316942,6.89902655578542,-8.19339868393687));
#14242=CARTESIAN_POINT('Ctrl Pts',(11.1454425256572,8.04889405860838,-8.68853919251131));
#14243=CARTESIAN_POINT('Ctrl Pts',(12.3775312688656,9.34238794408146,-9.24602752966092));
#14244=CARTESIAN_POINT('Ctrl Pts',(13.7465187613193,10.779712402918,-9.86499535005157));
#14245=CARTESIAN_POINT('Ctrl Pts',(14.2941137583009,11.354640872798,-10.1125880646808));
#14246=CARTESIAN_POINT('Ctrl Pts',(14.8417087552824,11.9295571981554,-10.3602324253388));
#14247=CARTESIAN_POINT('Ctrl Pts',(15.3208543776412,12.4326127553978,-10.5769051976768));
#14248=CARTESIAN_POINT('Ctrl Pts',(15.5946518761319,12.7200777462785,-10.7006983402633));
#14249=CARTESIAN_POINT('Ctrl Pts',(15.7315506253773,12.8638090371883,-10.7626000339661));
#14250=CARTESIAN_POINT('Ctrl Pts',(15.8,12.9356757561148,-10.793546315752));
#14251=CARTESIAN_POINT('Ctrl Pts',(10.0502525316942,6.51604789180995,-8.36661813687799));
#14252=CARTESIAN_POINT('Ctrl Pts',(11.1454425256572,7.63881390938369,-8.89900085425541));
#14253=CARTESIAN_POINT('Ctrl Pts',(12.3775312688656,8.90205445633837,-9.49738068383037));
#14254=CARTESIAN_POINT('Ctrl Pts',(13.7465187613194,10.3055239107478,-10.1628080503653));
#14255=CARTESIAN_POINT('Ctrl Pts',(14.2941137583009,10.8669132727126,-10.4289722391039));
#14256=CARTESIAN_POINT('Ctrl Pts',(14.8417087552824,11.4283172433782,-10.6950739523901));
#14257=CARTESIAN_POINT('Ctrl Pts',(15.3208543776412,11.9195411796877,-10.9279323587878));
#14258=CARTESIAN_POINT('Ctrl Pts',(15.5946518761319,12.2002349513456,-11.061018341967));
#14259=CARTESIAN_POINT('Ctrl Pts',(15.7315506253773,12.3405832861097,-11.1275551370521));
#14260=CARTESIAN_POINT('Ctrl Pts',(15.8,12.4107561622081,-11.1608290568882));
#14261=CARTESIAN_POINT('Ctrl Pts',(10.0502525316942,6.25935291859363,-8.32768215464935));
#14262=CARTESIAN_POINT('Ctrl Pts',(11.1454425256572,7.35179456409853,-8.87221159590509));
#14263=CARTESIAN_POINT('Ctrl Pts',(12.3775312688656,8.5807059309797,-9.48507728715609));
#14264=CARTESIAN_POINT('Ctrl Pts',(13.7465187613193,9.94625006691878,-10.1657641132886));
#14265=CARTESIAN_POINT('Ctrl Pts',(14.2941137583008,10.4924666723322,-10.4380421577189));
#14266=CARTESIAN_POINT('Ctrl Pts',(14.8417087552823,11.0386735802612,-10.7103508393265));
#14267=CARTESIAN_POINT('Ctrl Pts',(15.3208543776411,11.5166076371098,-10.9486114186505));
#14268=CARTESIAN_POINT('Ctrl Pts',(15.5946518761319,11.7897165434404,-11.0847485338421));
#14269=CARTESIAN_POINT('Ctrl Pts',(15.7315506253773,11.9262700347798,-11.1528201301259));
#14270=CARTESIAN_POINT('Ctrl Pts',(15.8,11.9945476376239,-11.1868532202044));
#14271=CARTESIAN_POINT('Ctrl Pts',(10.0502525316942,6.10559301495173,-8.23761851725688));
#14272=CARTESIAN_POINT('Ctrl Pts',(11.1454425256572,7.17588579216884,-8.7818172744299));
#14273=CARTESIAN_POINT('Ctrl Pts',(12.3775312688656,8.37997276877533,-9.39427431712614));
#14274=CARTESIAN_POINT('Ctrl Pts',(13.7465187613193,9.71783944471698,-10.0745443941304));
#14275=CARTESIAN_POINT('Ctrl Pts',(14.2941137583008,10.2529862083793,-10.3466552894421));
#14276=CARTESIAN_POINT('Ctrl Pts',(14.8417087552823,10.7881338344522,-10.61879266668));
#14277=CARTESIAN_POINT('Ctrl Pts',(15.3208543776412,11.2563877393682,-10.856904645461));
#14278=CARTESIAN_POINT('Ctrl Pts',(15.5946518761319,11.5239610675182,-10.9929584447386));
#14279=CARTESIAN_POINT('Ctrl Pts',(15.7315506253773,11.6577478171298,-11.060987970935));
#14280=CARTESIAN_POINT('Ctrl Pts',(15.8,11.7246411157058,-11.0950003932583));
#14281=CARTESIAN_POINT('Ctrl Pts',(10.0502525316941,5.94621492062452,-8.15474945546092));
#14282=CARTESIAN_POINT('Ctrl Pts',(11.1454425256572,6.99511596848632,-8.69826758958589));
#14283=CARTESIAN_POINT('Ctrl Pts',(12.3775312688656,8.17501015002258,-9.30992859260386));
#14284=CARTESIAN_POINT('Ctrl Pts',(13.7465187613193,9.48612538727717,-9.98934507962172));
#14285=CARTESIAN_POINT('Ctrl Pts',(14.2941137583008,10.0105700158496,-10.2611141666576));
#14286=CARTESIAN_POINT('Ctrl Pts',(14.8417087552823,10.535001088446,-10.532906293941));
#14287=CARTESIAN_POINT('Ctrl Pts',(15.3208543776412,10.9938824879741,-10.7707172481292));
#14288=CARTESIAN_POINT('Ctrl Pts',(15.5946518761319,11.2561056460575,-10.9066003574976));
#14289=CARTESIAN_POINT('Ctrl Pts',(15.7315506253773,11.3872158805765,-10.9745441973833));
#14290=CARTESIAN_POINT('Ctrl Pts',(15.8,11.4527721960679,-11.0085140807661));
#14291=CARTESIAN_POINT('Ctrl Pts',(10.0502525316942,5.69326714724857,-8.04752551167496));
#14292=CARTESIAN_POINT('Ctrl Pts',(11.1454425256572,6.70961935691121,-8.59278030111934));
#14293=CARTESIAN_POINT('Ctrl Pts',(12.3775312688656,7.85307681747464,-9.20628631668584));
#14294=CARTESIAN_POINT('Ctrl Pts',(13.7465187613193,9.12352275260843,-9.8878635484672));
#14295=CARTESIAN_POINT('Ctrl Pts',(14.2941137583008,9.63170187793886,-10.1604955992679));
#14296=CARTESIAN_POINT('Ctrl Pts',(14.8417087552823,10.1398879487016,-10.4331383564046));
#14297=CARTESIAN_POINT('Ctrl Pts',(15.3208543776412,10.5845486031013,-10.6716974431005));
#14298=CARTESIAN_POINT('Ctrl Pts',(15.5946518761319,10.8386377334452,-10.8080128020807));
#14299=CARTESIAN_POINT('Ctrl Pts',(15.7315506253773,10.9656829874862,-10.8761715434576));
#14300=CARTESIAN_POINT('Ctrl Pts',(15.8,11.0292050005901,-10.9102499677978));
#14301=CARTESIAN_POINT('Ctrl Pts',(10.0502525316942,5.49454791241252,-7.88548479029561));
#14302=CARTESIAN_POINT('Ctrl Pts',(11.1454425256572,6.48004349322276,-8.42454600598801));
#14303=CARTESIAN_POINT('Ctrl Pts',(12.3775312688655,7.5887300381936,-9.03106484753221));
#14304=CARTESIAN_POINT('Ctrl Pts',(13.7465187613193,8.82059988637917,-9.70489831419831));
#14305=CARTESIAN_POINT('Ctrl Pts',(14.2941137583008,9.31334787493986,-9.97443262085553));
#14306=CARTESIAN_POINT('Ctrl Pts',(14.8417087552823,9.8060963191458,-10.2439754326772));
#14307=CARTESIAN_POINT('Ctrl Pts',(15.3208543776411,10.2372510662851,-10.4798227509907));
#14308=CARTESIAN_POINT('Ctrl Pts',(15.5946518761319,10.4836250322036,-10.6145893749119));
#14309=CARTESIAN_POINT('Ctrl Pts',(15.7315506253773,10.6068120603552,-10.6819735304405));
#14310=CARTESIAN_POINT('Ctrl Pts',(15.8,10.6684055341558,-10.7156648564213));
#14311=CARTESIAN_POINT('Ctrl Pts',(10.0502525316942,5.32519947010607,-7.70626127860212));
#14312=CARTESIAN_POINT('Ctrl Pts',(11.1454425256572,6.28278149366019,-8.23464403472028));
#14313=CARTESIAN_POINT('Ctrl Pts',(12.3775312688656,7.3600274050152,-8.82914182271549));
#14314=CARTESIAN_POINT('Ctrl Pts',(13.7465187613194,8.55700179652725,-9.48962649341722));
#14315=CARTESIAN_POINT('Ctrl Pts',(14.2941137583009,9.03579113757914,-9.75382118614166));
#14316=CARTESIAN_POINT('Ctrl Pts',(14.8417087552824,9.51457663691211,-10.0180235007136));
#14317=CARTESIAN_POINT('Ctrl Pts',(15.3208543776412,9.93351514221374,-10.2491981583259));
#14318=CARTESIAN_POINT('Ctrl Pts',(15.594651876132,10.172910051869,-10.3812950302631));
#14319=CARTESIAN_POINT('Ctrl Pts',(15.7315506253773,10.2926071256634,-10.4473442221896));
#14320=CARTESIAN_POINT('Ctrl Pts',(15.8,10.3524560021355,-10.480368144447));
#14321=CARTESIAN_POINT('Ctrl Pts',(10.0502525316942,5.25663803961482,-7.60403044672135));
#14322=CARTESIAN_POINT('Ctrl Pts',(11.1454425256572,6.20120028598869,-8.12499465989843));
#14323=CARTESIAN_POINT('Ctrl Pts',(12.3775312688656,7.2639348461738,-8.71111815506916));
#14324=CARTESIAN_POINT('Ctrl Pts',(13.7465187613193,8.44464710847933,-9.36232701259537));
#14325=CARTESIAN_POINT('Ctrl Pts',(14.2941137583009,8.91693326542986,-9.62281103116557));
#14326=CARTESIAN_POINT('Ctrl Pts',(14.8417087552824,9.38923099717743,-9.88329944620756));
#14327=CARTESIAN_POINT('Ctrl Pts',(15.3208543776412,9.80248791688054,-10.1112254436565));
#14328=CARTESIAN_POINT('Ctrl Pts',(15.5946518761319,10.0386302748779,-10.2414671792814));
#14329=CARTESIAN_POINT('Ctrl Pts',(15.7315506253773,10.1567026018999,-10.3065884831493));
#14330=CARTESIAN_POINT('Ctrl Pts',(15.8,10.2157377422983,-10.3391487464728));
#14331=CARTESIAN_POINT('Ctrl Pts',(10.0502525316942,5.21733945232202,-7.53128682236137));
#14332=CARTESIAN_POINT('Ctrl Pts',(11.1454425256572,6.15376086042613,-8.04642571042556));
#14333=CARTESIAN_POINT('Ctrl Pts',(12.3775312688656,7.20723494454326,-8.62595695949777));
#14334=CARTESIAN_POINT('Ctrl Pts',(13.7465187613193,8.37776170467339,-9.269880569578));
#14335=CARTESIAN_POINT('Ctrl Pts',(14.2941137583009,8.84597240872545,-9.52745001361009));
#14336=CARTESIAN_POINT('Ctrl Pts',(14.8417087552824,9.31418311277751,-9.78501945764219));
#14337=CARTESIAN_POINT('Ctrl Pts',(15.3208543776412,9.72386747882305,-10.0103927211703));
#14338=CARTESIAN_POINT('Ctrl Pts',(15.5946518761319,9.95797283084908,-10.1391774431863));
#14339=CARTESIAN_POINT('Ctrl Pts',(15.7315506253773,10.0750255068621,-10.2035698041943));
#14340=CARTESIAN_POINT('Ctrl Pts',(15.8,10.1335518448686,-10.2357659846983));
#14341=CARTESIAN_POINT('Ctrl Pts',(15.8,10.160938779711,-10.2694450138623));
#14342=CARTESIAN_POINT('Ctrl Pts',(15.8,10.1553950350833,-10.2627800357942));
#14343=CARTESIAN_POINT('Ctrl Pts',(15.8,10.1498844772774,-10.2560796357392));
#14344=CARTESIAN_POINT('Ctrl Pts',(15.8,10.1444070962816,-10.2493438236809));
#14345=CARTESIAN_POINT('Ctrl Pts',(15.8,10.1389628855307,-10.242572606579));
#14346=CARTESIAN_POINT('Ctrl Pts',(15.8,10.1335518448686,-10.2357659846983));
#14347=CARTESIAN_POINT('Origin',(15.8,11.5149238208745,-9.70545143020505));
#14348=CARTESIAN_POINT('Ctrl Pts',(10.0502525316942,4.29750123086779,-9.86553218952114));
#14349=CARTESIAN_POINT('Ctrl Pts',(11.9668350211294,5.98055897313701,-11.2772850923971));
#14350=CARTESIAN_POINT('Ctrl Pts',(13.8834175105647,7.66361671540623,-12.689037995273));
#14351=CARTESIAN_POINT('Ctrl Pts',(15.8,9.34667445767544,-14.1007908981489));
#14352=CARTESIAN_POINT('Ctrl Pts',(10.0502525316942,4.02946472694721,-9.92430165934404));
#14353=CARTESIAN_POINT('Ctrl Pts',(11.9668350211294,5.67542688932036,-11.3702854403574));
#14354=CARTESIAN_POINT('Ctrl Pts',(13.8834175105647,7.32120731702057,-12.8166324188796));
#14355=CARTESIAN_POINT('Ctrl Pts',(15.8,8.96716947939372,-14.262616199893));
#14356=CARTESIAN_POINT('Ctrl Pts',(10.0502525316942,3.61211062987325,-9.97045860619056));
#14357=CARTESIAN_POINT('Ctrl Pts',(11.9668350211294,5.19299729643613,-11.4635526451079));
#14358=CARTESIAN_POINT('Ctrl Pts',(13.8834175105647,6.77411605990066,-12.956112555571));
#14359=CARTESIAN_POINT('Ctrl Pts',(15.8,8.35500272646353,-14.4492065944883));
#14360=CARTESIAN_POINT('Ctrl Pts',(10.0502525316942,3.40259706500423,-9.86609404202409));
#14361=CARTESIAN_POINT('Ctrl Pts',(11.9668350211294,4.93192196434906,-11.3629139742223));
#14362=CARTESIAN_POINT('Ctrl Pts',(13.8834175105647,6.4612970474202,-12.8596985741914));
#14363=CARTESIAN_POINT('Ctrl Pts',(15.8,7.99062194676503,-14.3565185063896));
#14364=CARTESIAN_POINT('Ctrl Pts',(10.0502525316942,3.30601090928165,-9.77087387154055));
#14365=CARTESIAN_POINT('Ctrl Pts',(11.9668350211295,4.80688444200921,-11.2600017151873));
#14366=CARTESIAN_POINT('Ctrl Pts',(13.8834175105647,6.30755492143113,-12.7494883087275));
#14367=CARTESIAN_POINT('Ctrl Pts',(15.8,7.8084284541587,-14.2386161523742));
#14368=CARTESIAN_POINT('Ctrl Pts',(10.0502525316942,3.24522078037662,-9.7053049496755));
#14369=CARTESIAN_POINT('Ctrl Pts',(11.9668350211294,4.72781700580773,-11.1883166806211));
#14370=CARTESIAN_POINT('Ctrl Pts',(13.8834175105647,6.21037804061049,-12.6715703878316));
#14371=CARTESIAN_POINT('Ctrl Pts',(15.8,7.69297426604161,-14.1545821187772));
#14372=CARTESIAN_POINT('Ctrl Pts',(10.0502525316942,3.13558852137588,-9.59290229251195));
#14373=CARTESIAN_POINT('Ctrl Pts',(11.9668350211294,4.58744122478927,-11.0646742694967));
#14374=CARTESIAN_POINT('Ctrl Pts',(13.8834175105647,6.03905717649217,-12.5366026187688));
#14375=CARTESIAN_POINT('Ctrl Pts',(15.8,7.49090987990556,-14.0083745957535));
#14376=CARTESIAN_POINT('Ctrl Pts',(10.0502525316942,2.92757116168118,-9.41310152025599));
#14377=CARTESIAN_POINT('Ctrl Pts',(11.9668350211294,4.32424671627921,-10.8702564567215));
#14378=CARTESIAN_POINT('Ctrl Pts',(13.8834175105647,5.72097159497831,-12.3275956094625));
#14379=CARTESIAN_POINT('Ctrl Pts',(15.8,7.11764714957634,-13.784750545928));
#14380=CARTESIAN_POINT('Ctrl Pts',(10.0502525316942,2.78894862571458,-9.19740926566327));
#14381=CARTESIAN_POINT('Ctrl Pts',(11.9668350211294,4.13765656795513,-10.6275127538178));
#14382=CARTESIAN_POINT('Ctrl Pts',(13.8834175105647,5.48632659127461,-12.0577280234799));
#14383=CARTESIAN_POINT('Ctrl Pts',(15.8,6.83503453351516,-13.4878315116344));
#14384=CARTESIAN_POINT('Ctrl Pts',(10.0502525316942,2.68315129602989,-8.97469639188219));
#14385=CARTESIAN_POINT('Ctrl Pts',(11.9668350211294,3.99115284441713,-10.3719655284903));
#14386=CARTESIAN_POINT('Ctrl Pts',(13.8834175105647,5.29909475352164,-11.7692966119437));
#14387=CARTESIAN_POINT('Ctrl Pts',(15.8,6.60709630190888,-13.1665657485518));
#14388=CARTESIAN_POINT('Ctrl Pts',(10.0502525316942,2.64958522759923,-8.85625319397989));
#14389=CARTESIAN_POINT('Ctrl Pts',(11.9668350211294,3.93994688562079,-10.2341088589535));
#14390=CARTESIAN_POINT('Ctrl Pts',(13.8834175105647,5.23040962052304,-11.612095695752));
#14391=CARTESIAN_POINT('Ctrl Pts',(15.8,6.5207712785446,-12.9899513607256));
#14392=CARTESIAN_POINT('Ctrl Pts',(10.0502525316942,2.63468906623289,-8.77492596468499));
#14393=CARTESIAN_POINT('Ctrl Pts',(11.9668350211294,3.91464433600868,-10.1386945339445));
#14394=CARTESIAN_POINT('Ctrl Pts',(13.8834175105647,5.19459960578446,-11.5024631032041));
#14395=CARTESIAN_POINT('Ctrl Pts',(15.8,6.47455487556025,-12.8662316724636));
#14396=CARTESIAN_POINT('Ctrl Pts',(15.8,6.49019400603777,-12.9067253609027));
#14397=CARTESIAN_POINT('Ctrl Pts',(15.8,6.48698118307512,-12.8986734787776));
#14398=CARTESIAN_POINT('Ctrl Pts',(15.8,6.48381086865141,-12.890598163633));
#14399=CARTESIAN_POINT('Ctrl Pts',(15.8,6.48068305016014,-12.8824994218701));
#14400=CARTESIAN_POINT('Ctrl Pts',(15.8,6.47759771920651,-12.874377258079));
#14401=CARTESIAN_POINT('Ctrl Pts',(15.8,6.47455487556025,-12.8662316724636));
#14402=CARTESIAN_POINT('Origin',(15.8,7.95219390447097,-12.7887399758658));
#14403=CARTESIAN_POINT('Ctrl Pts',(10.0502525316942,1.03854944428814,-10.7106795892491));
#14404=CARTESIAN_POINT('Ctrl Pts',(11.9668350211294,2.20297683852746,-12.5734298318033));
#14405=CARTESIAN_POINT('Ctrl Pts',(13.8834175105647,3.36740423276678,-14.4361800743576));
#14406=CARTESIAN_POINT('Ctrl Pts',(15.8,4.5318316270061,-16.2989303169119));
#14407=CARTESIAN_POINT('Ctrl Pts',(10.0502525316942,0.765470815703813,-10.6837448416591));
#14408=CARTESIAN_POINT('Ctrl Pts',(11.9668350211294,1.88404029388038,-12.5675874193204));
#14409=CARTESIAN_POINT('Ctrl Pts',(13.8834175105647,3.00232469790949,-14.4517192592367));
#14410=CARTESIAN_POINT('Ctrl Pts',(15.8,4.12089417608606,-16.335561836898));
#14411=CARTESIAN_POINT('Ctrl Pts',(10.0502525316942,0.354275884655604,-10.5986742216641));
#14412=CARTESIAN_POINT('Ctrl Pts',(11.9668350211294,1.39639701818897,-12.5072118829665));
#14413=CARTESIAN_POINT('Ctrl Pts',(13.8834175105647,2.43890221878171,-14.4153151096236));
#14414=CARTESIAN_POINT('Ctrl Pts',(15.8,3.48102335231507,-16.3238527709261));
#14415=CARTESIAN_POINT('Ctrl Pts',(10.0502525316942,0.187261072828497,-10.4346757823309));
#14416=CARTESIAN_POINT('Ctrl Pts',(11.9668350211294,1.17919268731442,-12.3308235163868));
#14417=CARTESIAN_POINT('Ctrl Pts',(13.8834175105647,2.17117887432506,-14.2269575174279));
#14418=CARTESIAN_POINT('Ctrl Pts',(15.8,3.16311048881099,-16.1231052514838));
#14419=CARTESIAN_POINT('Ctrl Pts',(10.0502525316942,0.124824203483031,-10.3142698682631));
#14420=CARTESIAN_POINT('Ctrl Pts',(11.9668350211295,1.09207394643473,-12.1943100355803));
#14421=CARTESIAN_POINT('Ctrl Pts',(13.8834175105647,2.05901454824881,-14.0746341437949));
#14422=CARTESIAN_POINT('Ctrl Pts',(15.8,3.02626429120051,-15.9546743111121));
#14423=CARTESIAN_POINT('Ctrl Pts',(10.0502525316942,0.0872711810328548,
-10.2331249635989));
#14424=CARTESIAN_POINT('Ctrl Pts',(11.9668350211294,1.03902815454411,-12.1017003635113));
#14425=CARTESIAN_POINT('Ctrl Pts',(13.8834175105647,1.99067177195527,-13.9705005205662));
#14426=CARTESIAN_POINT('Ctrl Pts',(15.8,2.94242874546653,-15.8390759204785));
#14427=CARTESIAN_POINT('Ctrl Pts',(10.0502525316942,0.0177390798696538,
-10.09234540735));
#14428=CARTESIAN_POINT('Ctrl Pts',(11.9668350211294,0.943730501418605,-11.9407308952458));
#14429=CARTESIAN_POINT('Ctrl Pts',(13.8834175105647,1.86944300220408,-13.789197555515));
#14430=CARTESIAN_POINT('Ctrl Pts',(15.8,2.79543442375303,-15.6375830434108));
#14431=CARTESIAN_POINT('Ctrl Pts',(10.0502525316942,-0.124535428292434,
-9.85706386916291));
#14432=CARTESIAN_POINT('Ctrl Pts',(11.9668350211294,0.753496320252983,-11.6744970487389));
#14433=CARTESIAN_POINT('Ctrl Pts',(13.8834175105647,1.63151416409049,-13.4921256030567));
#14434=CARTESIAN_POINT('Ctrl Pts',(15.8,2.50954591263591,-15.3095587826327));
#14435=CARTESIAN_POINT('Ctrl Pts',(10.0502525316942,-0.189717758784556,
-9.60909091476054));
#14436=CARTESIAN_POINT('Ctrl Pts',(11.9668350211294,0.651053436707715,-11.3859738307471));
#14437=CARTESIAN_POINT('Ctrl Pts',(13.8834175105647,1.49175101418763,-13.1629551482145));
#14438=CARTESIAN_POINT('Ctrl Pts',(15.8,2.3325222096799,-14.9398380642011));
#14439=CARTESIAN_POINT('Ctrl Pts',(10.0502525316942,-0.221513186022214,
-9.36458479377687));
#14440=CARTESIAN_POINT('Ctrl Pts',(11.9668350211294,0.590690300968106,-11.0976614182865));
#14441=CARTESIAN_POINT('Ctrl Pts',(13.8834175105648,1.40281548080797,-12.8307816497324));
#14442=CARTESIAN_POINT('Ctrl Pts',(15.8,2.21501896779829,-14.563858274242));
#14443=CARTESIAN_POINT('Ctrl Pts',(10.0502525316942,-0.216827447239561,
-9.24156417346731));
#14444=CARTESIAN_POINT('Ctrl Pts',(11.9668350211294,0.58459859972662,-10.9507264633732));
#14445=CARTESIAN_POINT('Ctrl Pts',(13.8834175105647,1.38608024219576,-12.6600447395717));
#14446=CARTESIAN_POINT('Ctrl Pts',(15.8,2.18750628916194,-14.3692070294775));
#14447=CARTESIAN_POINT('Ctrl Pts',(10.0502525316942,-0.205863042617262,
-9.15961421508102));
#14448=CARTESIAN_POINT('Ctrl Pts',(11.9668350211294,0.590019092973715,-10.8521631299943));
#14449=CARTESIAN_POINT('Ctrl Pts',(13.8834175105647,1.38590122856469,-12.5447120449076));
#14450=CARTESIAN_POINT('Ctrl Pts',(15.8,2.18178336415567,-14.2372609598209));
#14451=CARTESIAN_POINT('Ctrl Pts',(15.8,2.18414382321291,-14.2806055031745));
#14452=CARTESIAN_POINT('Ctrl Pts',(15.8,2.18357641541193,-14.2719548913156));
#14453=CARTESIAN_POINT('Ctrl Pts',(15.8,2.18305667683517,-14.2632951291918));
#14454=CARTESIAN_POINT('Ctrl Pts',(15.8,2.18258459351507,-14.2546262189952));
#14455=CARTESIAN_POINT('Ctrl Pts',(15.8,2.18216015604921,-14.2459481624974));
#14456=CARTESIAN_POINT('Ctrl Pts',(15.8,2.18178336415567,-14.2372609598209));
#14457=CARTESIAN_POINT('Origin',(15.8,3.61104784250494,-14.6201775482978));
#14458=CARTESIAN_POINT('Ctrl Pts',(10.0502525316942,-2.32206279789789,-10.5073910450885));
#14459=CARTESIAN_POINT('Ctrl Pts',(11.1454425256572,-2.01816863800157,-11.7253388222013));
#14460=CARTESIAN_POINT('Ctrl Pts',(12.3775312688656,-1.67628770811821,-13.0955300714531));
#14461=CARTESIAN_POINT('Ctrl Pts',(13.7465187613193,-1.29642000824781,-14.617964792844));
#14462=CARTESIAN_POINT('Ctrl Pts',(14.2941137583009,-1.14447292829965,-15.2269386814004));
#14463=CARTESIAN_POINT('Ctrl Pts',(14.8417087552824,-0.992525848351484,
-15.8359125699568));
#14464=CARTESIAN_POINT('Ctrl Pts',(15.3208543776412,-0.859572153396842,
-16.3687647224436));
#14465=CARTESIAN_POINT('Ctrl Pts',(15.5946518761319,-0.783598613422762,
-16.6732516667218));
#14466=CARTESIAN_POINT('Ctrl Pts',(15.7315506253773,-0.745611843435722,
-16.8254951388609));
#14467=CARTESIAN_POINT('Ctrl Pts',(15.8,-0.726618458442201,-16.9016168749304));
#14468=CARTESIAN_POINT('Ctrl Pts',(10.0502525316942,-2.57345271232946,-10.3973886408451));
#14469=CARTESIAN_POINT('Ctrl Pts',(11.1454425256572,-2.29815463811993,-11.618687280661));
#14470=CARTESIAN_POINT('Ctrl Pts',(12.3775312688656,-1.98887116228557,-12.9928273987101));
#14471=CARTESIAN_POINT('Ctrl Pts',(13.7465187613193,-1.64478997784958,-14.519468077176));
#14472=CARTESIAN_POINT('Ctrl Pts',(14.2941137583009,-1.50716238874916,-15.1301263986154));
#14473=CARTESIAN_POINT('Ctrl Pts',(14.8417087552824,-1.36958497392712,-15.740805777741));
#14474=CARTESIAN_POINT('Ctrl Pts',(15.3208543776412,-1.24918922664557,-16.2751437253593));
#14475=CARTESIAN_POINT('Ctrl Pts',(15.5946518761319,-1.18037249165619,-16.5804716520035));
#14476=CARTESIAN_POINT('Ctrl Pts',(15.7315506253773,-1.14596909077302,-16.7331376997671));
#14477=CARTESIAN_POINT('Ctrl Pts',(15.8,-1.12876296113493,-16.8094688647556));
#14478=CARTESIAN_POINT('Ctrl Pts',(10.0502525316942,-2.93870070814822,-10.189368118401));
#14479=CARTESIAN_POINT('Ctrl Pts',(11.1454425256572,-2.70946206711307,-11.4106316171747));
#14480=CARTESIAN_POINT('Ctrl Pts',(12.3775312688656,-2.45105312324518,-12.7843360022416));
#14481=CARTESIAN_POINT('Ctrl Pts',(13.7465187613194,-2.16445481731473,-14.310894320163));
#14482=CARTESIAN_POINT('Ctrl Pts',(14.2941137583009,-2.04980959621707,-14.9215151635443));
#14483=CARTESIAN_POINT('Ctrl Pts',(14.8417087552824,-1.93510378473095,-15.5321104940175));
#14484=CARTESIAN_POINT('Ctrl Pts',(15.3208543776412,-1.83475492870442,-16.0663892944466));
#14485=CARTESIAN_POINT('Ctrl Pts',(15.5946518761319,-1.77743586902583,-16.3717012113088));
#14486=CARTESIAN_POINT('Ctrl Pts',(15.7315506253773,-1.7487703415134,-16.5243546442885));
#14487=CARTESIAN_POINT('Ctrl Pts',(15.8,-1.7344429264487,-16.6006836129618));
#14488=CARTESIAN_POINT('Ctrl Pts',(10.0502525316942,-3.05808383535427,-9.95881139224219));
#14489=CARTESIAN_POINT('Ctrl Pts',(11.1454425256572,-2.85649631904975,-11.1626816238278));
#14490=CARTESIAN_POINT('Ctrl Pts',(12.3775312688656,-2.62997738853438,-12.5171248305866));
#14491=CARTESIAN_POINT('Ctrl Pts',(13.7465187613193,-2.37801889657081,-14.0219712727573));
#14492=CARTESIAN_POINT('Ctrl Pts',(14.2941137583008,-2.27723855544496,-14.6239108703276));
#14493=CARTESIAN_POINT('Ctrl Pts',(14.8417087552823,-2.17648960137064,-15.225860952321));
#14494=CARTESIAN_POINT('Ctrl Pts',(15.3208543776412,-2.08832456454097,-15.7525640332375));
#14495=CARTESIAN_POINT('Ctrl Pts',(15.5946518761319,-2.03793255455516,-16.0535332175881));
#14496=CARTESIAN_POINT('Ctrl Pts',(15.7315506253773,-2.01273965647872,-16.2040188475872));
#14497=CARTESIAN_POINT('Ctrl Pts',(15.8,-2.00014043670969,-16.2792607370613));
#14498=CARTESIAN_POINT('Ctrl Pts',(10.0502525316942,-3.07559947603194,-9.78147886731912));
#14499=CARTESIAN_POINT('Ctrl Pts',(11.1454425256572,-2.88676320881927,-10.9672359168267));
#14500=CARTESIAN_POINT('Ctrl Pts',(12.3775312688656,-2.67450622091512,-12.3013551830101));
#14501=CARTESIAN_POINT('Ctrl Pts',(13.7465187613194,-2.4384787180816,-13.7835653267336));
#14502=CARTESIAN_POINT('Ctrl Pts',(14.2941137583009,-2.34406982037813,-14.3764510158762));
#14503=CARTESIAN_POINT('Ctrl Pts',(14.8417087552824,-2.2496825286364,-14.9693534649946));
#14504=CARTESIAN_POINT('Ctrl Pts',(15.3208543776412,-2.16708696976893,-15.4881379273167));
#14505=CARTESIAN_POINT('Ctrl Pts',(15.5946518761319,-2.11988125471031,-15.7845797896778));
#14506=CARTESIAN_POINT('Ctrl Pts',(15.7315506253773,-2.09628053589475,-15.9328023798814));
#14507=CARTESIAN_POINT('Ctrl Pts',(15.8,-2.08447826919396,-16.0069121954757));
#14508=CARTESIAN_POINT('Ctrl Pts',(10.0502525316942,-3.10223684531881,-9.60383008034201));
#14509=CARTESIAN_POINT('Ctrl Pts',(11.1454425256572,-2.92542368552958,-10.7718807970721));
#14510=CARTESIAN_POINT('Ctrl Pts',(12.3775312688656,-2.72674232124834,-12.0859609655105));
#14511=CARTESIAN_POINT('Ctrl Pts',(13.7465187613193,-2.50574851695231,-13.5460266034681));
#14512=CARTESIAN_POINT('Ctrl Pts',(14.2941137583008,-2.41735366657092,-14.1300531231308));
#14513=CARTESIAN_POINT('Ctrl Pts',(14.8417087552824,-2.32898625556579,-14.7140823594691));
#14514=CARTESIAN_POINT('Ctrl Pts',(15.3208543776412,-2.25165628918294,-15.2251071015168));
#14515=CARTESIAN_POINT('Ctrl Pts',(15.5946518761319,-2.20745725592095,-15.5171202021386));
#14516=CARTESIAN_POINT('Ctrl Pts',(15.7315506253773,-2.18536045543708,-15.6631270213657));
#14517=CARTESIAN_POINT('Ctrl Pts',(15.8,-2.17430963295026,-15.7361301911613));
#14518=CARTESIAN_POINT('Ctrl Pts',(10.0502525316942,-3.16416975479849,-9.33616641898042));
#14519=CARTESIAN_POINT('Ctrl Pts',(11.1454425256572,-3.00789330574877,-10.4789053528453));
#14520=CARTESIAN_POINT('Ctrl Pts',(12.3775312688656,-2.83212323706007,-11.7645911992084));
#14521=CARTESIAN_POINT('Ctrl Pts',(13.7465187613193,-2.6367816468882,-13.1930250082462));
#14522=CARTESIAN_POINT('Ctrl Pts',(14.2941137583008,-2.55864547926934,-13.7643997282132));
#14523=CARTESIAN_POINT('Ctrl Pts',(14.8417087552823,-2.48051412346291,-14.3357867368398));
#14524=CARTESIAN_POINT('Ctrl Pts',(15.3208543776412,-2.4121476997586,-14.8357465708549));
#14525=CARTESIAN_POINT('Ctrl Pts',(15.5946518761319,-2.37307933395524,-15.1214332106675));
#14526=CARTESIAN_POINT('Ctrl Pts',(15.7315506253773,-2.35354562736142,-15.2642777469938));
#14527=CARTESIAN_POINT('Ctrl Pts',(15.8,-2.34377834929582,-15.3356989303604));
#14528=CARTESIAN_POINT('Ctrl Pts',(10.0502525316942,-3.14987939962279,-9.08015411140624));
#14529=CARTESIAN_POINT('Ctrl Pts',(11.1454425256572,-3.0067293155267,-10.19428901683));
#14530=CARTESIAN_POINT('Ctrl Pts',(12.3775312688656,-2.84574388114627,-11.4477380681646));
#14531=CARTESIAN_POINT('Ctrl Pts',(13.7465187613193,-2.66681194224705,-12.8404112867165));
#14532=CARTESIAN_POINT('Ctrl Pts',(14.2941137583008,-2.59523983509501,-13.3974811152093));
#14533=CARTESIAN_POINT('Ctrl Pts',(14.8417087552823,-2.52367459367681,-13.9545565014729));
#14534=CARTESIAN_POINT('Ctrl Pts',(15.3208543776412,-2.46105288517697,-14.4419957464975));
#14535=CARTESIAN_POINT('Ctrl Pts',(15.5946518761319,-2.42526642923796,-14.7205303350335));
#14536=CARTESIAN_POINT('Ctrl Pts',(15.7315506253773,-2.40737388088825,-14.8597981794497));
#14537=CARTESIAN_POINT('Ctrl Pts',(15.8,-2.39842700063224,-14.9294316110386));
#14538=CARTESIAN_POINT('Ctrl Pts',(10.0502525316942,-3.10442465522081,-8.83780343943476));
#14539=CARTESIAN_POINT('Ctrl Pts',(11.1454425256572,-2.96904269314958,-9.92307916160989));
#14540=CARTESIAN_POINT('Ctrl Pts',(12.3775312688656,-2.81681208487056,-11.1440266947135));
#14541=CARTESIAN_POINT('Ctrl Pts',(13.7465187613194,-2.64759182043347,-12.5006225450517));
#14542=CARTESIAN_POINT('Ctrl Pts',(14.2941137583009,-2.5799045625987,-13.0432610264625));
#14543=CARTESIAN_POINT('Ctrl Pts',(14.8417087552824,-2.51222601461465,-13.585900959023));
#14544=CARTESIAN_POINT('Ctrl Pts',(15.3208543776412,-2.45300459283688,-14.0607104514503));
#14545=CARTESIAN_POINT('Ctrl Pts',(15.594651876132,-2.41916045348293,-14.3320296071118));
#14546=CARTESIAN_POINT('Ctrl Pts',(15.7315506253773,-2.40223924596973,-14.4676893285877));
#14547=CARTESIAN_POINT('Ctrl Pts',(15.8,-2.39377787334028,-14.5355190612237));
#14548=CARTESIAN_POINT('Ctrl Pts',(10.0502525316942,-3.06201554081689,-8.72224646189196));
#14549=CARTESIAN_POINT('Ctrl Pts',(11.1454425256572,-2.92828468444751,-9.79262845293104));
#14550=CARTESIAN_POINT('Ctrl Pts',(12.3775312688656,-2.77780914227504,-10.9969124481398));
#14551=CARTESIAN_POINT('Ctrl Pts',(13.7465187613193,-2.61064282371592,-12.3349000504671));
#14552=CARTESIAN_POINT('Ctrl Pts',(14.2941137583009,-2.54377597211689,-12.870096284426));
#14553=CARTESIAN_POINT('Ctrl Pts',(14.8417087552824,-2.47690579066087,-13.4053047729009));
#14554=CARTESIAN_POINT('Ctrl Pts',(15.3208543776412,-2.41839541117503,-13.8736084123374));
#14555=CARTESIAN_POINT('Ctrl Pts',(15.5946518761319,-2.38496218052017,-14.1412058111469));
#14556=CARTESIAN_POINT('Ctrl Pts',(15.7315506253773,-2.3682452355795,-14.2750057235919));
#14557=CARTESIAN_POINT('Ctrl Pts',(15.8,-2.35988705705642,-14.3419045980318));
#14558=CARTESIAN_POINT('Ctrl Pts',(10.0502525316942,-3.02626384252387,-8.64769560732005));
#14559=CARTESIAN_POINT('Ctrl Pts',(11.1454425256572,-2.89260526381667,-9.70806748165927));
#14560=CARTESIAN_POINT('Ctrl Pts',(12.3775312688656,-2.74223936277106,-10.9009858402909));
#14561=CARTESIAN_POINT('Ctrl Pts',(13.7465187613193,-2.57516613938705,-12.2264506832149));
#14562=CARTESIAN_POINT('Ctrl Pts',(14.2941137583009,-2.50833685003344,-12.7566366203845));
#14563=CARTESIAN_POINT('Ctrl Pts',(14.8417087552824,-2.44150756067984,-13.2868225575541));
#14564=CARTESIAN_POINT('Ctrl Pts',(15.3208543776412,-2.38303193249543,-13.7507352525775));
#14565=CARTESIAN_POINT('Ctrl Pts',(15.5946518761319,-2.34961728781863,-14.0158282211623));
#14566=CARTESIAN_POINT('Ctrl Pts',(15.7315506253773,-2.33290996548023,-14.1483747054547));
#14567=CARTESIAN_POINT('Ctrl Pts',(15.8,-2.32455630431103,-14.2146479476009));
#14568=CARTESIAN_POINT('Ctrl Pts',(15.8,-2.33570557485288,-14.2566004799664));
#14569=CARTESIAN_POINT('Ctrl Pts',(15.8,-2.33357202566325,-14.2481979205348));
#14570=CARTESIAN_POINT('Ctrl Pts',(15.8,-2.33139031275994,-14.2398013892846));
#14571=CARTESIAN_POINT('Ctrl Pts',(15.8,-2.32916045010432,-14.2314108839843));
#14572=CARTESIAN_POINT('Ctrl Pts',(15.8,-2.326882447186,-14.2230264034132));
#14573=CARTESIAN_POINT('Ctrl Pts',(15.8,-2.32455630431103,-14.2146479476009));
#14574=CARTESIAN_POINT('Origin',(15.8,-1.08357274193521,-15.0204902775358));
#14575=CARTESIAN_POINT('Ctrl Pts',(10.0502525316942,-5.45537535466284,-9.2755658561365));
#14576=CARTESIAN_POINT('Ctrl Pts',(11.1454425256572,-5.54272139501843,-10.527811485966));
#14577=CARTESIAN_POINT('Ctrl Pts',(12.3775312688656,-5.64098569041847,-11.9365878195243));
#14578=CARTESIAN_POINT('Ctrl Pts',(13.7465187613193,-5.75016824086296,-13.5018948568112));
#14579=CARTESIAN_POINT('Ctrl Pts',(14.2941137583009,-5.79384126104075,-14.1280176717259));
#14580=CARTESIAN_POINT('Ctrl Pts',(14.8417087552824,-5.83751428121855,-14.7541404866407));
#14581=CARTESIAN_POINT('Ctrl Pts',(15.3208543776412,-5.87572817387412,-15.3019979496911));
#14582=CARTESIAN_POINT('Ctrl Pts',(15.5946518761319,-5.89756468396302,-15.6150593571485));
#14583=CARTESIAN_POINT('Ctrl Pts',(15.7315506253773,-5.90848293900746,-15.7715900608772));
#14584=CARTESIAN_POINT('Ctrl Pts',(15.8,-5.91394206652969,-15.8498554127416));
#14585=CARTESIAN_POINT('Ctrl Pts',(10.0502525316942,-5.66046875858054,-9.09326359699885));
#14586=CARTESIAN_POINT('Ctrl Pts',(11.1454425256572,-5.77604676609019,-10.3398594101876));
#14587=CARTESIAN_POINT('Ctrl Pts',(12.3775312688656,-5.90654052031257,-11.7423187718539));
#14588=CARTESIAN_POINT('Ctrl Pts',(13.7465187613193,-6.05105541408884,-13.3005670731329));
#14589=CARTESIAN_POINT('Ctrl Pts',(14.2941137583009,-6.10886731837785,-13.9238668895967));
#14590=CARTESIAN_POINT('Ctrl Pts',(14.8417087552824,-6.16673138983645,-14.5471710567224));
#14591=CARTESIAN_POINT('Ctrl Pts',(15.3208543776412,-6.21734620559881,-15.0925608480023));
#14592=CARTESIAN_POINT('Ctrl Pts',(15.5946518761319,-6.24624880770452,-15.4042104768461));
#14593=CARTESIAN_POINT('Ctrl Pts',(15.7315506253773,-6.26070528969669,-15.5600357233504));
#14594=CARTESIAN_POINT('Ctrl Pts',(15.8,-6.26792891516604,-15.6379479616747));
#14595=CARTESIAN_POINT('Ctrl Pts',(10.0502525316942,-5.94355560685309,-8.78255765938311));
#14596=CARTESIAN_POINT('Ctrl Pts',(11.1454425256572,-6.10292787924083,-10.0148869038525));
#14597=CARTESIAN_POINT('Ctrl Pts',(12.3775312688656,-6.2816544949474,-11.4012092316412));
#14598=CARTESIAN_POINT('Ctrl Pts',(13.7465187613194,-6.48081852219944,-12.9416164381759));
#14599=CARTESIAN_POINT('Ctrl Pts',(14.2941137583009,-6.56047693355264,-13.5577787105922));
#14600=CARTESIAN_POINT('Ctrl Pts',(14.8417087552824,-6.64007218801815,-14.1739356301478));
#14601=CARTESIAN_POINT('Ctrl Pts',(15.3208543776412,-6.70973770503938,-14.7130746018355));
#14602=CARTESIAN_POINT('Ctrl Pts',(15.594651876132,-6.74957096648566,-15.0211560817903));
#14603=CARTESIAN_POINT('Ctrl Pts',(15.7315506253773,-6.76948132483471,-15.1751962901528));
#14604=CARTESIAN_POINT('Ctrl Pts',(15.8,-6.77944209185894,-15.2522168679322));
#14605=CARTESIAN_POINT('Ctrl Pts',(10.0502525316942,-5.98584659003549,-8.52639512605652));
#14606=CARTESIAN_POINT('Ctrl Pts',(11.1454425256572,-6.16614182963237,-9.73363772297167));
#14607=CARTESIAN_POINT('Ctrl Pts',(12.3775312688656,-6.36925721416675,-11.0917875706281));
#14608=CARTESIAN_POINT('Ctrl Pts',(13.7465187613193,-6.59465188812854,-12.6008409910269));
#14609=CARTESIAN_POINT('Ctrl Pts',(14.2941137583008,-6.68481335297615,-13.2044623836355));
#14610=CARTESIAN_POINT('Ctrl Pts',(14.8417087552823,-6.77500635669625,-13.8080839907189));
#14611=CARTESIAN_POINT('Ctrl Pts',(15.3208543776412,-6.85391541259334,-14.3362528301216));
#14612=CARTESIAN_POINT('Ctrl Pts',(15.5946518761319,-6.89899411967348,-14.6380635126529));
#14613=CARTESIAN_POINT('Ctrl Pts',(15.7315506253773,-6.92153660547059,-14.7889688752189));
#14614=CARTESIAN_POINT('Ctrl Pts',(15.8,-6.9328050579454,-14.8644215375261));
#14615=CARTESIAN_POINT('Ctrl Pts',(10.0502525316942,-5.94770436886828,-8.35233000922534));
#14616=CARTESIAN_POINT('Ctrl Pts',(11.1454425256572,-6.13452948592056,-9.5384055936255));
#14617=CARTESIAN_POINT('Ctrl Pts',(12.3775312688656,-6.34492663085593,-10.8728200811769));
#14618=CARTESIAN_POINT('Ctrl Pts',(13.7465187613193,-6.57847782979355,-12.3554217499083));
#14619=CARTESIAN_POINT('Ctrl Pts',(14.2941137583008,-6.67190108779269,-12.9484634259519));
#14620=CARTESIAN_POINT('Ctrl Pts',(14.8417087552824,-6.76534871907581,-13.541513949349));
#14621=CARTESIAN_POINT('Ctrl Pts',(15.3208543776412,-6.84710780571679,-14.0604304019321));
#14622=CARTESIAN_POINT('Ctrl Pts',(15.5946518761319,-6.89381786952799,-14.3569506718));
#14623=CARTESIAN_POINT('Ctrl Pts',(15.7315506253773,-6.91717532204614,-14.5052116854016));
#14624=CARTESIAN_POINT('Ctrl Pts',(15.8,-6.92885189186191,-14.5793414094266));
#14625=CARTESIAN_POINT('Ctrl Pts',(10.0502525316942,-5.91814205125966,-8.1751443698686));
#14626=CARTESIAN_POINT('Ctrl Pts',(11.1454425256572,-6.11093026523681,-9.34066488658195));
#14627=CARTESIAN_POINT('Ctrl Pts',(12.3775312688656,-6.32804641946555,-10.6518240329443));
#14628=CARTESIAN_POINT('Ctrl Pts',(13.7465187613193,-6.56905244176938,-12.1087200255634));
#14629=CARTESIAN_POINT('Ctrl Pts',(14.2941137583008,-6.66545776271567,-12.6914777697296));
#14630=CARTESIAN_POINT('Ctrl Pts',(14.8417087552823,-6.76188862893655,-13.2742297865971));
#14631=CARTESIAN_POINT('Ctrl Pts',(15.3208543776412,-6.84625768114735,-13.7841395850464));
#14632=CARTESIAN_POINT('Ctrl Pts',(15.5946518761319,-6.89445870116997,-14.0755188249216));
#14633=CARTESIAN_POINT('Ctrl Pts',(15.7315506253773,-6.9185617481891,-14.2212078760573));
#14634=CARTESIAN_POINT('Ctrl Pts',(15.8,-6.93061101156267,-14.2940529083518));
#14635=CARTESIAN_POINT('Ctrl Pts',(10.0502525316942,-5.8943312499999,-7.90144264462466));
#14636=CARTESIAN_POINT('Ctrl Pts',(11.1454425256572,-6.09882926548584,-9.03654403267794));
#14637=CARTESIAN_POINT('Ctrl Pts',(12.3775312688656,-6.32895925304843,-10.3136205759385));
#14638=CARTESIAN_POINT('Ctrl Pts',(13.7465187613193,-6.58458807992399,-11.7325052253954));
#14639=CARTESIAN_POINT('Ctrl Pts',(14.2941137583008,-6.68684049565601,-12.3000601956136));
#14640=CARTESIAN_POINT('Ctrl Pts',(14.8417087552823,-6.7891006747503,-12.86762490695));
#14641=CARTESIAN_POINT('Ctrl Pts',(15.3208543776411,-6.87857591366296,-13.364240995629));
#14642=CARTESIAN_POINT('Ctrl Pts',(15.5946518761319,-6.92970162298621,-13.6480178551891));
#14643=CARTESIAN_POINT('Ctrl Pts',(15.7315506253773,-6.95526524865974,-13.7899072524002));
#14644=CARTESIAN_POINT('Ctrl Pts',(15.8,-6.96804637462761,-13.8608510891535));
#14645=CARTESIAN_POINT('Ctrl Pts',(10.0502525316942,-5.80163007173558,-7.66237562613099));
#14646=CARTESIAN_POINT('Ctrl Pts',(11.1454425256572,-6.00977287125004,-8.76621669669801));
#14647=CARTESIAN_POINT('Ctrl Pts',(12.3775312688656,-6.24400287259235,-10.008064757174));
#14648=CARTESIAN_POINT('Ctrl Pts',(13.7465187613193,-6.50418764618811,-11.3878685250288));
#14649=CARTESIAN_POINT('Ctrl Pts',(14.2941137583008,-6.60826243593386,-11.9397903730643));
#14650=CARTESIAN_POINT('Ctrl Pts',(14.8417087552823,-6.71234494803684,-12.4917152115347));
#14651=CARTESIAN_POINT('Ctrl Pts',(15.3208543776411,-6.80341474110257,-12.9746485138656));
#14652=CARTESIAN_POINT('Ctrl Pts',(15.5946518761319,-6.85545164006593,-13.2506092458454));
#14653=CARTESIAN_POINT('Ctrl Pts',(15.7315506253773,-6.88147085648712,-13.388589908828));
#14654=CARTESIAN_POINT('Ctrl Pts',(15.8,-6.89447978145678,-13.4575799757384));
#14655=CARTESIAN_POINT('Ctrl Pts',(10.0502525316942,-5.68351040711504,-7.44593237535689));
#14656=CARTESIAN_POINT('Ctrl Pts',(11.1454425256572,-5.89012315163304,-8.51992624992032));
#14657=CARTESIAN_POINT('Ctrl Pts',(12.3775312688656,-6.12263633930509,-9.72815762348205));
#14658=CARTESIAN_POINT('Ctrl Pts',(13.7465187613194,-6.38090895110341,-11.0706489050023));
#14659=CARTESIAN_POINT('Ctrl Pts',(14.2941137583009,-6.4842189332274,-11.60764526865));
#14660=CARTESIAN_POINT('Ctrl Pts',(14.8417087552824,-6.58753713858487,-12.1446403255654));
#14661=CARTESIAN_POINT('Ctrl Pts',(15.3208543776412,-6.6779380072571,-12.6145114073305));
#14662=CARTESIAN_POINT('Ctrl Pts',(15.594651876132,-6.72959247024461,-12.8830096730692));
#14663=CARTESIAN_POINT('Ctrl Pts',(15.7315506253773,-6.755420518422,-13.0172586761616));
#14664=CARTESIAN_POINT('Ctrl Pts',(15.8,-6.76833381495438,-13.0843832933218));
#14665=CARTESIAN_POINT('Ctrl Pts',(10.0502525316942,-5.60747221894231,-7.34913449516209));
#14666=CARTESIAN_POINT('Ctrl Pts',(11.1454425256572,-5.81105284226644,-8.40845336995523));
#14667=CARTESIAN_POINT('Ctrl Pts',(12.3775312688656,-6.04008639989118,-9.60029668798142));
#14668=CARTESIAN_POINT('Ctrl Pts',(13.7465187613193,-6.29456266363366,-10.9244551954278));
#14669=CARTESIAN_POINT('Ctrl Pts',(14.2941137583009,-6.3963532371211,-11.4541199893924));
#14670=CARTESIAN_POINT('Ctrl Pts',(14.8417087552824,-6.49814440704391,-11.9837969855611));
#14671=CARTESIAN_POINT('Ctrl Pts',(15.3208543776412,-6.58721149497458,-12.4472605569962));
#14672=CARTESIAN_POINT('Ctrl Pts',(15.5946518761319,-6.63810674341679,-12.7120921703849));
#14673=CARTESIAN_POINT('Ctrl Pts',(15.7315506253773,-6.66355442687238,-12.8445091889311));
#14674=CARTESIAN_POINT('Ctrl Pts',(15.8,-6.67627821583014,-12.9107166186057));
#14675=CARTESIAN_POINT('Ctrl Pts',(10.0502525316942,-5.55043285230422,-7.28928030147641));
#14676=CARTESIAN_POINT('Ctrl Pts',(11.1454425256572,-5.75098891959401,-8.33905665452735));
#14677=CARTESIAN_POINT('Ctrl Pts',(12.3775312688656,-5.97661449529503,-9.52005505170966));
#14678=CARTESIAN_POINT('Ctrl Pts',(13.7465187613193,-6.22730957940728,-10.8322754930233));
#14679=CARTESIAN_POINT('Ctrl Pts',(14.2941137583009,-6.32758761305217,-11.3571636695488));
#14680=CARTESIAN_POINT('Ctrl Pts',(14.8417087552824,-6.42786564669707,-11.8820518460743));
#14681=CARTESIAN_POINT('Ctrl Pts',(15.3208543776412,-6.51560892613635,-12.3413290005341));
#14682=CARTESIAN_POINT('Ctrl Pts',(15.5946518761319,-6.56574794295881,-12.6037730887968));
#14683=CARTESIAN_POINT('Ctrl Pts',(15.7315506253773,-6.59081745137003,-12.7349951329282));
#14684=CARTESIAN_POINT('Ctrl Pts',(15.8,-6.60335220557564,-12.8006061549939));
#14685=CARTESIAN_POINT('Ctrl Pts',(15.8,-6.62691983743441,-12.8370600702028));
#14686=CARTESIAN_POINT('Ctrl Pts',(15.8,-6.62229417791417,-12.8297280642598));
#14687=CARTESIAN_POINT('Ctrl Pts',(15.8,-6.61762457479065,-12.8224166748639));
#14688=CARTESIAN_POINT('Ctrl Pts',(15.8,-6.61291104065239,-12.8151258955788));
#14689=CARTESIAN_POINT('Ctrl Pts',(15.8,-6.60815358414732,-12.8078557223109));
#14690=CARTESIAN_POINT('Ctrl Pts',(15.8,-6.60335220557564,-12.8006061549939));
#14691=CARTESIAN_POINT('Origin',(15.8,-5.67212567669951,-13.950492764499));
#14692=CARTESIAN_POINT('Ctrl Pts',(10.0502525316942,-8.05467776187827,-7.13578365451838));
#14693=CARTESIAN_POINT('Ctrl Pts',(11.1454425256572,-8.52471396348012,-8.29974860990865));
#14694=CARTESIAN_POINT('Ctrl Pts',(12.3775312688656,-9.05350469028219,-9.6092091847227));
#14695=CARTESIAN_POINT('Ctrl Pts',(13.7465187613193,-9.6410499422845,-11.0641653789605));
#14696=CARTESIAN_POINT('Ctrl Pts',(14.2941137583009,-9.87606804308543,-11.6461478566557));
#14697=CARTESIAN_POINT('Ctrl Pts',(14.8417087552824,-10.1110861438864,-12.2281303343508));
#14698=CARTESIAN_POINT('Ctrl Pts',(15.3208543776412,-10.3167269820872,-12.737365002334));
#14699=CARTESIAN_POINT('Ctrl Pts',(15.5946518761319,-10.4342360324876,-13.0283562411816));
#14700=CARTESIAN_POINT('Ctrl Pts',(15.7315506253773,-10.4929905576879,-13.1738518606054));
#14701=CARTESIAN_POINT('Ctrl Pts',(15.8,-10.522367820288,-13.2465996703173));
#14702=CARTESIAN_POINT('Ctrl Pts',(10.0502525316942,-8.19339868393687,-6.89902655578542));
#14703=CARTESIAN_POINT('Ctrl Pts',(11.1454425256572,-8.68853919251131,-8.04889405860839));
#14704=CARTESIAN_POINT('Ctrl Pts',(12.3775312688656,-9.24602752966092,-9.34238794408146));
#14705=CARTESIAN_POINT('Ctrl Pts',(13.7465187613193,-9.86499535005157,-10.779712402918));
#14706=CARTESIAN_POINT('Ctrl Pts',(14.2941137583009,-10.1125880646808,-11.354640872798));
#14707=CARTESIAN_POINT('Ctrl Pts',(14.8417087552824,-10.3602324253388,-11.9295571981554));
#14708=CARTESIAN_POINT('Ctrl Pts',(15.3208543776412,-10.5769051976768,-12.4326127553978));
#14709=CARTESIAN_POINT('Ctrl Pts',(15.5946518761319,-10.7006983402633,-12.7200777462785));
#14710=CARTESIAN_POINT('Ctrl Pts',(15.7315506253773,-10.7626000339661,-12.8638090371883));
#14711=CARTESIAN_POINT('Ctrl Pts',(15.8,-10.793546315752,-12.9356757561148));
#14712=CARTESIAN_POINT('Ctrl Pts',(10.0502525316942,-8.36661813687798,-6.51604789180993));
#14713=CARTESIAN_POINT('Ctrl Pts',(11.1454425256572,-8.8990008542554,-7.63881390938367));
#14714=CARTESIAN_POINT('Ctrl Pts',(12.3775312688656,-9.49738068383039,-8.90205445633838));
#14715=CARTESIAN_POINT('Ctrl Pts',(13.7465187613194,-10.1628080503653,-10.3055239107478));
#14716=CARTESIAN_POINT('Ctrl Pts',(14.2941137583009,-10.4289722391039,-10.8669132727127));
#14717=CARTESIAN_POINT('Ctrl Pts',(14.8417087552824,-10.6950739523901,-11.4283172433782));
#14718=CARTESIAN_POINT('Ctrl Pts',(15.3208543776412,-10.9279323587878,-11.9195411796877));
#14719=CARTESIAN_POINT('Ctrl Pts',(15.594651876132,-11.0610183419671,-12.2002349513456));
#14720=CARTESIAN_POINT('Ctrl Pts',(15.7315506253773,-11.1275551370522,-12.3405832861097));
#14721=CARTESIAN_POINT('Ctrl Pts',(15.8,-11.1608290568883,-12.4107561622081));
#14722=CARTESIAN_POINT('Ctrl Pts',(10.0502525316942,-8.32768215464935,-6.25935291859366));
#14723=CARTESIAN_POINT('Ctrl Pts',(11.1454425256572,-8.87221159590509,-7.35179456409856));
#14724=CARTESIAN_POINT('Ctrl Pts',(12.3775312688656,-9.48507728715609,-8.58070593097969));
#14725=CARTESIAN_POINT('Ctrl Pts',(13.7465187613193,-10.1657641132886,-9.94625006691877));
#14726=CARTESIAN_POINT('Ctrl Pts',(14.2941137583008,-10.4380421577189,-10.4924666723322));
#14727=CARTESIAN_POINT('Ctrl Pts',(14.8417087552823,-10.7103508393265,-11.0386735802612));
#14728=CARTESIAN_POINT('Ctrl Pts',(15.3208543776412,-10.9486114186505,-11.5166076371098));
#14729=CARTESIAN_POINT('Ctrl Pts',(15.5946518761319,-11.0847485338421,-11.7897165434404));
#14730=CARTESIAN_POINT('Ctrl Pts',(15.7315506253773,-11.1528201301259,-11.9262700347798));
#14731=CARTESIAN_POINT('Ctrl Pts',(15.8,-11.1868532202043,-11.9945476376238));
#14732=CARTESIAN_POINT('Ctrl Pts',(10.0502525316942,-8.23761851725689,-6.10559301495173));
#14733=CARTESIAN_POINT('Ctrl Pts',(11.1454425256572,-8.78181727442991,-7.17588579216885));
#14734=CARTESIAN_POINT('Ctrl Pts',(12.3775312688656,-9.39427431712614,-8.37997276877534));
#14735=CARTESIAN_POINT('Ctrl Pts',(13.7465187613193,-10.0745443941304,-9.71783944471699));
#14736=CARTESIAN_POINT('Ctrl Pts',(14.2941137583009,-10.3466552894421,-10.2529862083793));
#14737=CARTESIAN_POINT('Ctrl Pts',(14.8417087552824,-10.61879266668,-10.7881338344522));
#14738=CARTESIAN_POINT('Ctrl Pts',(15.3208543776412,-10.856904645461,-11.2563877393682));
#14739=CARTESIAN_POINT('Ctrl Pts',(15.5946518761319,-10.9929584447386,-11.5239610675182));
#14740=CARTESIAN_POINT('Ctrl Pts',(15.7315506253773,-11.060987970935,-11.6577478171298));
#14741=CARTESIAN_POINT('Ctrl Pts',(15.8,-11.0950003932583,-11.7246411157058));
#14742=CARTESIAN_POINT('Ctrl Pts',(10.0502525316942,-8.15474945546092,-5.94621492062453));
#14743=CARTESIAN_POINT('Ctrl Pts',(11.1454425256572,-8.69826758958589,-6.99511596848632));
#14744=CARTESIAN_POINT('Ctrl Pts',(12.3775312688656,-9.30992859260386,-8.17501015002259));
#14745=CARTESIAN_POINT('Ctrl Pts',(13.7465187613193,-9.98934507962172,-9.48612538727718));
#14746=CARTESIAN_POINT('Ctrl Pts',(14.2941137583008,-10.2611141666576,-10.0105700158496));
#14747=CARTESIAN_POINT('Ctrl Pts',(14.8417087552823,-10.532906293941,-10.535001088446));
#14748=CARTESIAN_POINT('Ctrl Pts',(15.3208543776412,-10.7707172481292,-10.9938824879741));
#14749=CARTESIAN_POINT('Ctrl Pts',(15.5946518761319,-10.9066003574976,-11.2561056460575));
#14750=CARTESIAN_POINT('Ctrl Pts',(15.7315506253773,-10.9745441973833,-11.3872158805765));
#14751=CARTESIAN_POINT('Ctrl Pts',(15.8,-11.0085140807661,-11.4527721960679));
#14752=CARTESIAN_POINT('Ctrl Pts',(10.0502525316942,-8.04752551167497,-5.69326714724858));
#14753=CARTESIAN_POINT('Ctrl Pts',(11.1454425256572,-8.59278030111935,-6.70961935691122));
#14754=CARTESIAN_POINT('Ctrl Pts',(12.3775312688656,-9.20628631668585,-7.85307681747465));
#14755=CARTESIAN_POINT('Ctrl Pts',(13.7465187613193,-9.8878635484672,-9.12352275260843));
#14756=CARTESIAN_POINT('Ctrl Pts',(14.2941137583008,-10.1604955992679,-9.63170187793887));
#14757=CARTESIAN_POINT('Ctrl Pts',(14.8417087552824,-10.4331383564046,-10.1398879487016));
#14758=CARTESIAN_POINT('Ctrl Pts',(15.3208543776412,-10.6716974431005,-10.5845486031013));
#14759=CARTESIAN_POINT('Ctrl Pts',(15.5946518761319,-10.8080128020807,-10.8386377334453));
#14760=CARTESIAN_POINT('Ctrl Pts',(15.7315506253773,-10.8761715434576,-10.9656829874862));
#14761=CARTESIAN_POINT('Ctrl Pts',(15.8,-10.9102499677978,-11.0292050005901));
#14762=CARTESIAN_POINT('Ctrl Pts',(10.0502525316942,-7.88548479029562,-5.49454791241254));
#14763=CARTESIAN_POINT('Ctrl Pts',(11.1454425256572,-8.42454600598801,-6.48004349322278));
#14764=CARTESIAN_POINT('Ctrl Pts',(12.3775312688656,-9.03106484753224,-7.58873003819356));
#14765=CARTESIAN_POINT('Ctrl Pts',(13.7465187613193,-9.70489831419834,-8.82059988637913));
#14766=CARTESIAN_POINT('Ctrl Pts',(14.2941137583008,-9.97443262085556,-9.31334787493982));
#14767=CARTESIAN_POINT('Ctrl Pts',(14.8417087552823,-10.2439754326772,-9.80609631914575));
#14768=CARTESIAN_POINT('Ctrl Pts',(15.3208543776411,-10.4798227509908,-10.237251066285));
#14769=CARTESIAN_POINT('Ctrl Pts',(15.5946518761319,-10.614589374912,-10.4836250322036));
#14770=CARTESIAN_POINT('Ctrl Pts',(15.7315506253773,-10.6819735304405,-10.6068120603551));
#14771=CARTESIAN_POINT('Ctrl Pts',(15.8,-10.7156648564213,-10.6684055341557));
#14772=CARTESIAN_POINT('Ctrl Pts',(10.0502525316942,-7.70626127860213,-5.32519947010611));
#14773=CARTESIAN_POINT('Ctrl Pts',(11.1454425256572,-8.23464403472029,-6.28278149366022));
#14774=CARTESIAN_POINT('Ctrl Pts',(12.3775312688656,-8.82914182271552,-7.36002740501521));
#14775=CARTESIAN_POINT('Ctrl Pts',(13.7465187613194,-9.48962649341726,-8.55700179652725));
#14776=CARTESIAN_POINT('Ctrl Pts',(14.2941137583009,-9.7538211861417,-9.03579113757913));
#14777=CARTESIAN_POINT('Ctrl Pts',(14.8417087552824,-10.0180235007137,-9.5145766369121));
#14778=CARTESIAN_POINT('Ctrl Pts',(15.3208543776412,-10.2491981583259,-9.93351514221373));
#14779=CARTESIAN_POINT('Ctrl Pts',(15.594651876132,-10.3812950302632,-10.172910051869));
#14780=CARTESIAN_POINT('Ctrl Pts',(15.7315506253773,-10.4473442221897,-10.2926071256634));
#14781=CARTESIAN_POINT('Ctrl Pts',(15.8,-10.4803681444471,-10.3524560021355));
#14782=CARTESIAN_POINT('Ctrl Pts',(10.0502525316942,-7.60403044672135,-5.25663803961482));
#14783=CARTESIAN_POINT('Ctrl Pts',(11.1454425256572,-8.12499465989843,-6.20120028598869));
#14784=CARTESIAN_POINT('Ctrl Pts',(12.3775312688656,-8.71111815506916,-7.26393484617381));
#14785=CARTESIAN_POINT('Ctrl Pts',(13.7465187613193,-9.36232701259537,-8.44464710847935));
#14786=CARTESIAN_POINT('Ctrl Pts',(14.2941137583009,-9.62281103116557,-8.91693326542987));
#14787=CARTESIAN_POINT('Ctrl Pts',(14.8417087552824,-9.88329944620756,-9.38923099717744));
#14788=CARTESIAN_POINT('Ctrl Pts',(15.3208543776412,-10.1112254436565,-9.80248791688055));
#14789=CARTESIAN_POINT('Ctrl Pts',(15.5946518761319,-10.2414671792814,-10.0386302748779));
#14790=CARTESIAN_POINT('Ctrl Pts',(15.7315506253773,-10.3065884831493,-10.1567026019));
#14791=CARTESIAN_POINT('Ctrl Pts',(15.8,-10.3391487464728,-10.2157377422983));
#14792=CARTESIAN_POINT('Ctrl Pts',(10.0502525316942,-7.53128682236137,-5.21733945232202));
#14793=CARTESIAN_POINT('Ctrl Pts',(11.1454425256572,-8.04642571042556,-6.15376086042613));
#14794=CARTESIAN_POINT('Ctrl Pts',(12.3775312688656,-8.62595695949777,-7.20723494454326));
#14795=CARTESIAN_POINT('Ctrl Pts',(13.7465187613193,-9.269880569578,-8.3777617046734));
#14796=CARTESIAN_POINT('Ctrl Pts',(14.2941137583009,-9.52745001361009,-8.84597240872545));
#14797=CARTESIAN_POINT('Ctrl Pts',(14.8417087552824,-9.78501945764219,-9.31418311277751));
#14798=CARTESIAN_POINT('Ctrl Pts',(15.3208543776412,-10.0103927211703,-9.72386747882306));
#14799=CARTESIAN_POINT('Ctrl Pts',(15.5946518761319,-10.1391774431863,-9.95797283084909));
#14800=CARTESIAN_POINT('Ctrl Pts',(15.7315506253773,-10.2035698041943,-10.0750255068621));
#14801=CARTESIAN_POINT('Ctrl Pts',(15.8,-10.2357659846983,-10.1335518448686));
#14802=CARTESIAN_POINT('Ctrl Pts',(15.8,-10.2694450138623,-10.160938779711));
#14803=CARTESIAN_POINT('Ctrl Pts',(15.8,-10.2627800357942,-10.1553950350833));
#14804=CARTESIAN_POINT('Ctrl Pts',(15.8,-10.2560796357392,-10.1498844772774));
#14805=CARTESIAN_POINT('Ctrl Pts',(15.8,-10.2493438236809,-10.1444070962816));
#14806=CARTESIAN_POINT('Ctrl Pts',(15.8,-10.242572606579,-10.1389628855307));
#14807=CARTESIAN_POINT('Ctrl Pts',(15.8,-10.2357659846983,-10.1335518448686));
#14808=CARTESIAN_POINT('Origin',(15.8,-9.70545143020505,-11.5149238208745));
#14809=CARTESIAN_POINT('Ctrl Pts',(10.0502525316942,-9.86553218952113,-4.29750123086779));
#14810=CARTESIAN_POINT('Ctrl Pts',(11.9668350211294,-11.2772850923971,-5.98055897313701));
#14811=CARTESIAN_POINT('Ctrl Pts',(13.8834175105647,-12.689037995273,-7.66361671540623));
#14812=CARTESIAN_POINT('Ctrl Pts',(15.8,-14.1007908981489,-9.34667445767544));
#14813=CARTESIAN_POINT('Ctrl Pts',(10.0502525316942,-9.92430165934405,-4.02946472694721));
#14814=CARTESIAN_POINT('Ctrl Pts',(11.9668350211294,-11.3702854403574,-5.67542688932036));
#14815=CARTESIAN_POINT('Ctrl Pts',(13.8834175105647,-12.8166324188796,-7.32120731702056));
#14816=CARTESIAN_POINT('Ctrl Pts',(15.8,-14.262616199893,-8.96716947939371));
#14817=CARTESIAN_POINT('Ctrl Pts',(10.0502525316942,-9.97045860619055,-3.61211062987325));
#14818=CARTESIAN_POINT('Ctrl Pts',(11.9668350211295,-11.4635526451079,-5.19299729643612));
#14819=CARTESIAN_POINT('Ctrl Pts',(13.8834175105647,-12.956112555571,-6.77411605990067));
#14820=CARTESIAN_POINT('Ctrl Pts',(15.8,-14.4492065944883,-8.35500272646354));
#14821=CARTESIAN_POINT('Ctrl Pts',(10.0502525316942,-9.86609404202411,-3.40259706500424));
#14822=CARTESIAN_POINT('Ctrl Pts',(11.9668350211295,-11.3629139742223,-4.93192196434907));
#14823=CARTESIAN_POINT('Ctrl Pts',(13.8834175105647,-12.8596985741914,-6.46129704742022));
#14824=CARTESIAN_POINT('Ctrl Pts',(15.8,-14.3565185063897,-7.99062194676505));
#14825=CARTESIAN_POINT('Ctrl Pts',(10.0502525316942,-9.77087387154056,-3.30601090928165));
#14826=CARTESIAN_POINT('Ctrl Pts',(11.9668350211295,-11.2600017151874,-4.80688444200922));
#14827=CARTESIAN_POINT('Ctrl Pts',(13.8834175105647,-12.7494883087275,-6.30755492143114));
#14828=CARTESIAN_POINT('Ctrl Pts',(15.8,-14.2386161523743,-7.80842845415871));
#14829=CARTESIAN_POINT('Ctrl Pts',(10.0502525316942,-9.70530494967552,-3.24522078037662));
#14830=CARTESIAN_POINT('Ctrl Pts',(11.9668350211295,-11.1883166806212,-4.72781700580775));
#14831=CARTESIAN_POINT('Ctrl Pts',(13.8834175105647,-12.6715703878316,-6.2103780406105));
#14832=CARTESIAN_POINT('Ctrl Pts',(15.8,-14.1545821187772,-7.69297426604162));
#14833=CARTESIAN_POINT('Ctrl Pts',(10.0502525316942,-9.59290229251197,-3.13558852137589));
#14834=CARTESIAN_POINT('Ctrl Pts',(11.9668350211294,-11.0646742694967,-4.58744122478928));
#14835=CARTESIAN_POINT('Ctrl Pts',(13.8834175105647,-12.5366026187688,-6.03905717649217));
#14836=CARTESIAN_POINT('Ctrl Pts',(15.8,-14.0083745957535,-7.49090987990556));
#14837=CARTESIAN_POINT('Ctrl Pts',(10.0502525316942,-9.413101520256,-2.92757116168118));
#14838=CARTESIAN_POINT('Ctrl Pts',(11.9668350211295,-10.8702564567215,-4.32424671627921));
#14839=CARTESIAN_POINT('Ctrl Pts',(13.8834175105647,-12.3275956094625,-5.72097159497833));
#14840=CARTESIAN_POINT('Ctrl Pts',(15.8,-13.784750545928,-7.11764714957635));
#14841=CARTESIAN_POINT('Ctrl Pts',(10.0502525316942,-9.19740926566326,-2.7889486257146));
#14842=CARTESIAN_POINT('Ctrl Pts',(11.9668350211294,-10.6275127538178,-4.13765656795515));
#14843=CARTESIAN_POINT('Ctrl Pts',(13.8834175105647,-12.0577280234798,-5.48632659127459));
#14844=CARTESIAN_POINT('Ctrl Pts',(15.8,-13.4878315116343,-6.83503453351514));
#14845=CARTESIAN_POINT('Ctrl Pts',(10.0502525316942,-8.97469639188219,-2.6831512960299));
#14846=CARTESIAN_POINT('Ctrl Pts',(11.9668350211294,-10.3719655284903,-3.99115284441713));
#14847=CARTESIAN_POINT('Ctrl Pts',(13.8834175105648,-11.7692966119438,-5.29909475352163));
#14848=CARTESIAN_POINT('Ctrl Pts',(15.8,-13.1665657485518,-6.60709630190887));
#14849=CARTESIAN_POINT('Ctrl Pts',(10.0502525316942,-8.85625319397989,-2.64958522759923));
#14850=CARTESIAN_POINT('Ctrl Pts',(11.9668350211294,-10.2341088589535,-3.93994688562079));
#14851=CARTESIAN_POINT('Ctrl Pts',(13.8834175105647,-11.612095695752,-5.23040962052305));
#14852=CARTESIAN_POINT('Ctrl Pts',(15.8,-12.9899513607256,-6.52077127854461));
#14853=CARTESIAN_POINT('Ctrl Pts',(10.0502525316942,-8.77492596468499,-2.63468906623289));
#14854=CARTESIAN_POINT('Ctrl Pts',(11.9668350211294,-10.1386945339445,-3.91464433600868));
#14855=CARTESIAN_POINT('Ctrl Pts',(13.8834175105647,-11.5024631032041,-5.19459960578446));
#14856=CARTESIAN_POINT('Ctrl Pts',(15.8,-12.8662316724636,-6.47455487556025));
#14857=CARTESIAN_POINT('Ctrl Pts',(15.8,-12.9067253609027,-6.49019400603777));
#14858=CARTESIAN_POINT('Ctrl Pts',(15.8,-12.8986734787776,-6.48698118307512));
#14859=CARTESIAN_POINT('Ctrl Pts',(15.8,-12.890598163633,-6.48381086865141));
#14860=CARTESIAN_POINT('Ctrl Pts',(15.8,-12.8824994218701,-6.48068305016014));
#14861=CARTESIAN_POINT('Ctrl Pts',(15.8,-12.874377258079,-6.47759771920651));
#14862=CARTESIAN_POINT('Ctrl Pts',(15.8,-12.8662316724636,-6.47455487556025));
#14863=CARTESIAN_POINT('Origin',(15.8,-12.7887399758658,-7.95219390447097));
#14864=CARTESIAN_POINT('Ctrl Pts',(10.0502525316942,-10.7106795892491,-1.03854944428814));
#14865=CARTESIAN_POINT('Ctrl Pts',(11.9668350211294,-12.5734298318033,-2.20297683852746));
#14866=CARTESIAN_POINT('Ctrl Pts',(13.8834175105647,-14.4361800743576,-3.36740423276678));
#14867=CARTESIAN_POINT('Ctrl Pts',(15.8,-16.2989303169119,-4.5318316270061));
#14868=CARTESIAN_POINT('Ctrl Pts',(10.0502525316942,-10.6837448416591,-0.765470815703814));
#14869=CARTESIAN_POINT('Ctrl Pts',(11.9668350211294,-12.5675874193204,-1.88404029388038));
#14870=CARTESIAN_POINT('Ctrl Pts',(13.8834175105647,-14.4517192592367,-3.00232469790949));
#14871=CARTESIAN_POINT('Ctrl Pts',(15.8,-16.335561836898,-4.12089417608606));
#14872=CARTESIAN_POINT('Ctrl Pts',(10.0502525316942,-10.5986742216641,-0.354275884655604));
#14873=CARTESIAN_POINT('Ctrl Pts',(11.9668350211294,-12.5072118829665,-1.39639701818897));
#14874=CARTESIAN_POINT('Ctrl Pts',(13.8834175105647,-14.4153151096236,-2.43890221878171));
#14875=CARTESIAN_POINT('Ctrl Pts',(15.8,-16.3238527709261,-3.48102335231507));
#14876=CARTESIAN_POINT('Ctrl Pts',(10.0502525316942,-10.4346757823309,-0.187261072828499));
#14877=CARTESIAN_POINT('Ctrl Pts',(11.9668350211294,-12.3308235163868,-1.17919268731443));
#14878=CARTESIAN_POINT('Ctrl Pts',(13.8834175105647,-14.2269575174279,-2.17117887432506));
#14879=CARTESIAN_POINT('Ctrl Pts',(15.8,-16.1231052514838,-3.16311048881098));
#14880=CARTESIAN_POINT('Ctrl Pts',(10.0502525316942,-10.3142698682631,-0.124824203483033));
#14881=CARTESIAN_POINT('Ctrl Pts',(11.9668350211295,-12.1943100355803,-1.09207394643473));
#14882=CARTESIAN_POINT('Ctrl Pts',(13.8834175105647,-14.0746341437949,-2.05901454824881));
#14883=CARTESIAN_POINT('Ctrl Pts',(15.8,-15.9546743111121,-3.02626429120051));
#14884=CARTESIAN_POINT('Ctrl Pts',(10.0502525316942,-10.2331249635989,-0.0872711810328558));
#14885=CARTESIAN_POINT('Ctrl Pts',(11.9668350211294,-12.1017003635113,-1.03902815454411));
#14886=CARTESIAN_POINT('Ctrl Pts',(13.8834175105647,-13.9705005205662,-1.99067177195527));
#14887=CARTESIAN_POINT('Ctrl Pts',(15.8,-15.8390759204785,-2.94242874546653));
#14888=CARTESIAN_POINT('Ctrl Pts',(10.0502525316942,-10.09234540735,-0.0177390798696546));
#14889=CARTESIAN_POINT('Ctrl Pts',(11.9668350211294,-11.9407308952458,-0.943730501418607));
#14890=CARTESIAN_POINT('Ctrl Pts',(13.8834175105647,-13.789197555515,-1.86944300220407));
#14891=CARTESIAN_POINT('Ctrl Pts',(15.8,-15.6375830434108,-2.79543442375303));
#14892=CARTESIAN_POINT('Ctrl Pts',(10.0502525316942,-9.85706386916291,0.124535428292433));
#14893=CARTESIAN_POINT('Ctrl Pts',(11.9668350211294,-11.6744970487389,-0.753496320252986));
#14894=CARTESIAN_POINT('Ctrl Pts',(13.8834175105647,-13.4921256030567,-1.63151416409049));
#14895=CARTESIAN_POINT('Ctrl Pts',(15.8,-15.3095587826327,-2.50954591263591));
#14896=CARTESIAN_POINT('Ctrl Pts',(10.0502525316942,-9.60909091476054,0.189717758784556));
#14897=CARTESIAN_POINT('Ctrl Pts',(11.9668350211294,-11.3859738307471,-0.651053436707714));
#14898=CARTESIAN_POINT('Ctrl Pts',(13.8834175105647,-13.1629551482145,-1.49175101418762));
#14899=CARTESIAN_POINT('Ctrl Pts',(15.8,-14.9398380642011,-2.33252220967989));
#14900=CARTESIAN_POINT('Ctrl Pts',(10.0502525316942,-9.36458479377687,0.221513186022213));
#14901=CARTESIAN_POINT('Ctrl Pts',(11.9668350211294,-11.0976614182865,-0.590690300968109));
#14902=CARTESIAN_POINT('Ctrl Pts',(13.8834175105648,-12.8307816497324,-1.40281548080796));
#14903=CARTESIAN_POINT('Ctrl Pts',(15.8,-14.563858274242,-2.21501896779828));
#14904=CARTESIAN_POINT('Ctrl Pts',(10.0502525316942,-9.24156417346731,0.21682744723956));
#14905=CARTESIAN_POINT('Ctrl Pts',(11.9668350211294,-10.9507264633732,-0.584598599726619));
#14906=CARTESIAN_POINT('Ctrl Pts',(13.8834175105647,-12.6600447395717,-1.38608024219576));
#14907=CARTESIAN_POINT('Ctrl Pts',(15.8,-14.3692070294775,-2.18750628916194));
#14908=CARTESIAN_POINT('Ctrl Pts',(10.0502525316942,-9.15961421508102,0.205863042617261));
#14909=CARTESIAN_POINT('Ctrl Pts',(11.9668350211294,-10.8521631299943,-0.590019092973716));
#14910=CARTESIAN_POINT('Ctrl Pts',(13.8834175105647,-12.5447120449076,-1.38590122856469));
#14911=CARTESIAN_POINT('Ctrl Pts',(15.8,-14.2372609598209,-2.18178336415567));
#14912=CARTESIAN_POINT('Ctrl Pts',(15.8,-14.2806055031745,-2.18414382321291));
#14913=CARTESIAN_POINT('Ctrl Pts',(15.8,-14.2719548913156,-2.18357641541193));
#14914=CARTESIAN_POINT('Ctrl Pts',(15.8,-14.2632951291918,-2.18305667683517));
#14915=CARTESIAN_POINT('Ctrl Pts',(15.8,-14.2546262189952,-2.18258459351507));
#14916=CARTESIAN_POINT('Ctrl Pts',(15.8,-14.2459481624974,-2.18216015604921));
#14917=CARTESIAN_POINT('Ctrl Pts',(15.8,-14.2372609598209,-2.18178336415567));
#14918=CARTESIAN_POINT('Origin',(15.8,-14.6201775482978,-3.61104784250494));
#14919=CARTESIAN_POINT('Ctrl Pts',(10.0502525316942,-10.5073910450885,2.32206279789789));
#14920=CARTESIAN_POINT('Ctrl Pts',(11.1454425256572,-11.7253388222013,2.01816863800157));
#14921=CARTESIAN_POINT('Ctrl Pts',(12.3775312688656,-13.0955300714531,1.67628770811821));
#14922=CARTESIAN_POINT('Ctrl Pts',(13.7465187613193,-14.617964792844,1.29642000824781));
#14923=CARTESIAN_POINT('Ctrl Pts',(14.2941137583009,-15.2269386814004,1.14447292829964));
#14924=CARTESIAN_POINT('Ctrl Pts',(14.8417087552824,-15.8359125699568,0.992525848351483));
#14925=CARTESIAN_POINT('Ctrl Pts',(15.3208543776412,-16.3687647224436,0.859572153396841));
#14926=CARTESIAN_POINT('Ctrl Pts',(15.5946518761319,-16.6732516667218,0.783598613422761));
#14927=CARTESIAN_POINT('Ctrl Pts',(15.7315506253773,-16.8254951388609,0.745611843435721));
#14928=CARTESIAN_POINT('Ctrl Pts',(15.8,-16.9016168749304,0.7266184584422));
#14929=CARTESIAN_POINT('Ctrl Pts',(10.0502525316942,-10.3973886408451,2.57345271232945));
#14930=CARTESIAN_POINT('Ctrl Pts',(11.1454425256572,-11.618687280661,2.29815463811993));
#14931=CARTESIAN_POINT('Ctrl Pts',(12.3775312688656,-12.9928273987101,1.98887116228557));
#14932=CARTESIAN_POINT('Ctrl Pts',(13.7465187613193,-14.519468077176,1.64478997784958));
#14933=CARTESIAN_POINT('Ctrl Pts',(14.2941137583009,-15.1301263986154,1.50716238874916));
#14934=CARTESIAN_POINT('Ctrl Pts',(14.8417087552824,-15.740805777741,1.36958497392712));
#14935=CARTESIAN_POINT('Ctrl Pts',(15.3208543776412,-16.2751437253593,1.24918922664557));
#14936=CARTESIAN_POINT('Ctrl Pts',(15.5946518761319,-16.5804716520035,1.18037249165619));
#14937=CARTESIAN_POINT('Ctrl Pts',(15.7315506253773,-16.7331376997671,1.14596909077302));
#14938=CARTESIAN_POINT('Ctrl Pts',(15.8,-16.8094688647556,1.12876296113493));
#14939=CARTESIAN_POINT('Ctrl Pts',(10.0502525316942,-10.189368118401,2.93870070814822));
#14940=CARTESIAN_POINT('Ctrl Pts',(11.1454425256572,-11.4106316171747,2.70946206711307));
#14941=CARTESIAN_POINT('Ctrl Pts',(12.3775312688656,-12.7843360022416,2.45105312324518));
#14942=CARTESIAN_POINT('Ctrl Pts',(13.7465187613194,-14.310894320163,2.16445481731473));
#14943=CARTESIAN_POINT('Ctrl Pts',(14.2941137583009,-14.9215151635443,2.04980959621707));
#14944=CARTESIAN_POINT('Ctrl Pts',(14.8417087552824,-15.5321104940175,1.93510378473096));
#14945=CARTESIAN_POINT('Ctrl Pts',(15.3208543776412,-16.0663892944466,1.83475492870443));
#14946=CARTESIAN_POINT('Ctrl Pts',(15.5946518761319,-16.3717012113088,1.77743586902584));
#14947=CARTESIAN_POINT('Ctrl Pts',(15.7315506253773,-16.5243546442885,1.7487703415134));
#14948=CARTESIAN_POINT('Ctrl Pts',(15.8,-16.6006836129618,1.7344429264487));
#14949=CARTESIAN_POINT('Ctrl Pts',(10.0502525316942,-9.95881139224219,3.05808383535426));
#14950=CARTESIAN_POINT('Ctrl Pts',(11.1454425256572,-11.1626816238278,2.85649631904974));
#14951=CARTESIAN_POINT('Ctrl Pts',(12.3775312688656,-12.5171248305866,2.62997738853437));
#14952=CARTESIAN_POINT('Ctrl Pts',(13.7465187613193,-14.0219712727573,2.37801889657081));
#14953=CARTESIAN_POINT('Ctrl Pts',(14.2941137583008,-14.6239108703276,2.27723855544496));
#14954=CARTESIAN_POINT('Ctrl Pts',(14.8417087552823,-15.225860952321,2.17648960137063));
#14955=CARTESIAN_POINT('Ctrl Pts',(15.3208543776412,-15.7525640332375,2.08832456454097));
#14956=CARTESIAN_POINT('Ctrl Pts',(15.5946518761319,-16.0535332175881,2.03793255455515));
#14957=CARTESIAN_POINT('Ctrl Pts',(15.7315506253773,-16.2040188475872,2.01273965647872));
#14958=CARTESIAN_POINT('Ctrl Pts',(15.8,-16.2792607370613,2.00014043670969));
#14959=CARTESIAN_POINT('Ctrl Pts',(10.0502525316942,-9.78147886731912,3.07559947603193));
#14960=CARTESIAN_POINT('Ctrl Pts',(11.1454425256572,-10.9672359168267,2.88676320881926));
#14961=CARTESIAN_POINT('Ctrl Pts',(12.3775312688656,-12.3013551830101,2.67450622091511));
#14962=CARTESIAN_POINT('Ctrl Pts',(13.7465187613194,-13.7835653267336,2.43847871808159));
#14963=CARTESIAN_POINT('Ctrl Pts',(14.2941137583009,-14.3764510158762,2.34406982037812));
#14964=CARTESIAN_POINT('Ctrl Pts',(14.8417087552824,-14.9693534649946,2.2496825286364));
#14965=CARTESIAN_POINT('Ctrl Pts',(15.3208543776412,-15.4881379273167,2.16708696976892));
#14966=CARTESIAN_POINT('Ctrl Pts',(15.5946518761319,-15.7845797896778,2.11988125471031));
#14967=CARTESIAN_POINT('Ctrl Pts',(15.7315506253773,-15.9328023798814,2.09628053589475));
#14968=CARTESIAN_POINT('Ctrl Pts',(15.8,-16.0069121954757,2.08447826919396));
#14969=CARTESIAN_POINT('Ctrl Pts',(10.0502525316942,-9.60383008034201,3.1022368453188));
#14970=CARTESIAN_POINT('Ctrl Pts',(11.1454425256572,-10.7718807970721,2.92542368552957));
#14971=CARTESIAN_POINT('Ctrl Pts',(12.3775312688656,-12.0859609655105,2.72674232124834));
#14972=CARTESIAN_POINT('Ctrl Pts',(13.7465187613193,-13.5460266034681,2.5057485169523));
#14973=CARTESIAN_POINT('Ctrl Pts',(14.2941137583008,-14.1300531231308,2.41735366657091));
#14974=CARTESIAN_POINT('Ctrl Pts',(14.8417087552824,-14.7140823594691,2.32898625556579));
#14975=CARTESIAN_POINT('Ctrl Pts',(15.3208543776412,-15.2251071015168,2.25165628918294));
#14976=CARTESIAN_POINT('Ctrl Pts',(15.5946518761319,-15.5171202021386,2.20745725592095));
#14977=CARTESIAN_POINT('Ctrl Pts',(15.7315506253773,-15.6631270213657,2.18536045543708));
#14978=CARTESIAN_POINT('Ctrl Pts',(15.8,-15.7361301911613,2.17430963295026));
#14979=CARTESIAN_POINT('Ctrl Pts',(10.0502525316942,-9.33616641898042,3.1641697547985));
#14980=CARTESIAN_POINT('Ctrl Pts',(11.1454425256572,-10.4789053528453,3.00789330574878));
#14981=CARTESIAN_POINT('Ctrl Pts',(12.3775312688656,-11.7645911992084,2.83212323706007));
#14982=CARTESIAN_POINT('Ctrl Pts',(13.7465187613193,-13.1930250082462,2.6367816468882));
#14983=CARTESIAN_POINT('Ctrl Pts',(14.2941137583008,-13.7643997282132,2.55864547926933));
#14984=CARTESIAN_POINT('Ctrl Pts',(14.8417087552823,-14.3357867368398,2.48051412346291));
#14985=CARTESIAN_POINT('Ctrl Pts',(15.3208543776412,-14.8357465708549,2.4121476997586));
#14986=CARTESIAN_POINT('Ctrl Pts',(15.5946518761319,-15.1214332106675,2.37307933395524));
#14987=CARTESIAN_POINT('Ctrl Pts',(15.7315506253773,-15.2642777469938,2.35354562736142));
#14988=CARTESIAN_POINT('Ctrl Pts',(15.8,-15.3356989303604,2.34377834929581));
#14989=CARTESIAN_POINT('Ctrl Pts',(10.0502525316942,-9.08015411140624,3.14987939962279));
#14990=CARTESIAN_POINT('Ctrl Pts',(11.1454425256572,-10.19428901683,3.0067293155267));
#14991=CARTESIAN_POINT('Ctrl Pts',(12.3775312688656,-11.4477380681646,2.84574388114627));
#14992=CARTESIAN_POINT('Ctrl Pts',(13.7465187613193,-12.8404112867165,2.66681194224705));
#14993=CARTESIAN_POINT('Ctrl Pts',(14.2941137583008,-13.3974811152093,2.59523983509501));
#14994=CARTESIAN_POINT('Ctrl Pts',(14.8417087552823,-13.9545565014729,2.52367459367682));
#14995=CARTESIAN_POINT('Ctrl Pts',(15.3208543776412,-14.4419957464975,2.46105288517697));
#14996=CARTESIAN_POINT('Ctrl Pts',(15.5946518761319,-14.7205303350335,2.42526642923796));
#14997=CARTESIAN_POINT('Ctrl Pts',(15.7315506253773,-14.8597981794497,2.40737388088825));
#14998=CARTESIAN_POINT('Ctrl Pts',(15.8,-14.9294316110386,2.39842700063224));
#14999=CARTESIAN_POINT('Ctrl Pts',(10.0502525316942,-8.83780343943476,3.10442465522081));
#15000=CARTESIAN_POINT('Ctrl Pts',(11.1454425256572,-9.92307916160989,2.96904269314958));
#15001=CARTESIAN_POINT('Ctrl Pts',(12.3775312688656,-11.1440266947135,2.81681208487056));
#15002=CARTESIAN_POINT('Ctrl Pts',(13.7465187613194,-12.5006225450517,2.64759182043347));
#15003=CARTESIAN_POINT('Ctrl Pts',(14.2941137583009,-13.0432610264625,2.57990456259871));
#15004=CARTESIAN_POINT('Ctrl Pts',(14.8417087552824,-13.585900959023,2.51222601461465));
#15005=CARTESIAN_POINT('Ctrl Pts',(15.3208543776412,-14.0607104514503,2.45300459283688));
#15006=CARTESIAN_POINT('Ctrl Pts',(15.594651876132,-14.3320296071118,2.41916045348293));
#15007=CARTESIAN_POINT('Ctrl Pts',(15.7315506253773,-14.4676893285877,2.40223924596973));
#15008=CARTESIAN_POINT('Ctrl Pts',(15.8,-14.5355190612237,2.39377787334028));
#15009=CARTESIAN_POINT('Ctrl Pts',(10.0502525316942,-8.72224646189196,3.06201554081689));
#15010=CARTESIAN_POINT('Ctrl Pts',(11.1454425256572,-9.79262845293104,2.92828468444751));
#15011=CARTESIAN_POINT('Ctrl Pts',(12.3775312688656,-10.9969124481398,2.77780914227504));
#15012=CARTESIAN_POINT('Ctrl Pts',(13.7465187613193,-12.3349000504671,2.61064282371592));
#15013=CARTESIAN_POINT('Ctrl Pts',(14.2941137583009,-12.870096284426,2.54377597211689));
#15014=CARTESIAN_POINT('Ctrl Pts',(14.8417087552824,-13.4053047729009,2.47690579066087));
#15015=CARTESIAN_POINT('Ctrl Pts',(15.3208543776412,-13.8736084123374,2.41839541117503));
#15016=CARTESIAN_POINT('Ctrl Pts',(15.5946518761319,-14.1412058111469,2.38496218052016));
#15017=CARTESIAN_POINT('Ctrl Pts',(15.7315506253773,-14.2750057235919,2.3682452355795));
#15018=CARTESIAN_POINT('Ctrl Pts',(15.8,-14.3419045980318,2.35988705705641));
#15019=CARTESIAN_POINT('Ctrl Pts',(10.0502525316942,-8.64769560732005,3.02626384252387));
#15020=CARTESIAN_POINT('Ctrl Pts',(11.1454425256572,-9.70806748165927,2.89260526381666));
#15021=CARTESIAN_POINT('Ctrl Pts',(12.3775312688656,-10.9009858402909,2.74223936277106));
#15022=CARTESIAN_POINT('Ctrl Pts',(13.7465187613193,-12.2264506832149,2.57516613938705));
#15023=CARTESIAN_POINT('Ctrl Pts',(14.2941137583009,-12.7566366203845,2.50833685003344));
#15024=CARTESIAN_POINT('Ctrl Pts',(14.8417087552824,-13.2868225575541,2.44150756067984));
#15025=CARTESIAN_POINT('Ctrl Pts',(15.3208543776412,-13.7507352525775,2.38303193249543));
#15026=CARTESIAN_POINT('Ctrl Pts',(15.5946518761319,-14.0158282211623,2.34961728781863));
#15027=CARTESIAN_POINT('Ctrl Pts',(15.7315506253773,-14.1483747054547,2.33290996548023));
#15028=CARTESIAN_POINT('Ctrl Pts',(15.8,-14.2146479476009,2.32455630431103));
#15029=CARTESIAN_POINT('Ctrl Pts',(15.8,-14.2566004799664,2.33570557485288));
#15030=CARTESIAN_POINT('Ctrl Pts',(15.8,-14.2481979205348,2.33357202566325));
#15031=CARTESIAN_POINT('Ctrl Pts',(15.8,-14.2398013892846,2.33139031275994));
#15032=CARTESIAN_POINT('Ctrl Pts',(15.8,-14.2314108839843,2.32916045010432));
#15033=CARTESIAN_POINT('Ctrl Pts',(15.8,-14.2230264034132,2.32688244718599));
#15034=CARTESIAN_POINT('Ctrl Pts',(15.8,-14.2146479476009,2.32455630431103));
#15035=CARTESIAN_POINT('Origin',(15.8,-15.0204902775358,1.08357274193521));
#15036=CARTESIAN_POINT('Ctrl Pts',(10.0502525316942,-9.2755658561365,5.45537535466284));
#15037=CARTESIAN_POINT('Ctrl Pts',(11.1454425256572,-10.527811485966,5.54272139501843));
#15038=CARTESIAN_POINT('Ctrl Pts',(12.3775312688656,-11.9365878195243,5.64098569041847));
#15039=CARTESIAN_POINT('Ctrl Pts',(13.7465187613193,-13.5018948568112,5.75016824086296));
#15040=CARTESIAN_POINT('Ctrl Pts',(14.2941137583009,-14.1280176717259,5.79384126104075));
#15041=CARTESIAN_POINT('Ctrl Pts',(14.8417087552824,-14.7541404866407,5.83751428121855));
#15042=CARTESIAN_POINT('Ctrl Pts',(15.3208543776412,-15.3019979496911,5.87572817387412));
#15043=CARTESIAN_POINT('Ctrl Pts',(15.5946518761319,-15.6150593571485,5.89756468396302));
#15044=CARTESIAN_POINT('Ctrl Pts',(15.7315506253773,-15.7715900608772,5.90848293900746));
#15045=CARTESIAN_POINT('Ctrl Pts',(15.8,-15.8498554127416,5.91394206652969));
#15046=CARTESIAN_POINT('Ctrl Pts',(10.0502525316942,-9.09326359699885,5.66046875858054));
#15047=CARTESIAN_POINT('Ctrl Pts',(11.1454425256572,-10.3398594101876,5.77604676609019));
#15048=CARTESIAN_POINT('Ctrl Pts',(12.3775312688656,-11.7423187718539,5.90654052031257));
#15049=CARTESIAN_POINT('Ctrl Pts',(13.7465187613193,-13.3005670731329,6.05105541408884));
#15050=CARTESIAN_POINT('Ctrl Pts',(14.2941137583009,-13.9238668895967,6.10886731837785));
#15051=CARTESIAN_POINT('Ctrl Pts',(14.8417087552824,-14.5471710567224,6.16673138983645));
#15052=CARTESIAN_POINT('Ctrl Pts',(15.3208543776412,-15.0925608480023,6.21734620559881));
#15053=CARTESIAN_POINT('Ctrl Pts',(15.5946518761319,-15.4042104768461,6.24624880770452));
#15054=CARTESIAN_POINT('Ctrl Pts',(15.7315506253773,-15.5600357233504,6.26070528969669));
#15055=CARTESIAN_POINT('Ctrl Pts',(15.8,-15.6379479616747,6.26792891516604));
#15056=CARTESIAN_POINT('Ctrl Pts',(10.0502525316942,-8.78255765938311,5.94355560685309));
#15057=CARTESIAN_POINT('Ctrl Pts',(11.1454425256572,-10.0148869038525,6.10292787924083));
#15058=CARTESIAN_POINT('Ctrl Pts',(12.3775312688656,-11.4012092316412,6.2816544949474));
#15059=CARTESIAN_POINT('Ctrl Pts',(13.7465187613194,-12.9416164381759,6.48081852219944));
#15060=CARTESIAN_POINT('Ctrl Pts',(14.2941137583009,-13.5577787105922,6.56047693355264));
#15061=CARTESIAN_POINT('Ctrl Pts',(14.8417087552824,-14.1739356301478,6.64007218801815));
#15062=CARTESIAN_POINT('Ctrl Pts',(15.3208543776412,-14.7130746018355,6.70973770503938));
#15063=CARTESIAN_POINT('Ctrl Pts',(15.594651876132,-15.0211560817903,6.74957096648566));
#15064=CARTESIAN_POINT('Ctrl Pts',(15.7315506253773,-15.1751962901528,6.76948132483471));
#15065=CARTESIAN_POINT('Ctrl Pts',(15.8,-15.2522168679322,6.77944209185894));
#15066=CARTESIAN_POINT('Ctrl Pts',(10.0502525316942,-8.52639512605652,5.98584659003549));
#15067=CARTESIAN_POINT('Ctrl Pts',(11.1454425256572,-9.73363772297167,6.16614182963237));
#15068=CARTESIAN_POINT('Ctrl Pts',(12.3775312688656,-11.0917875706281,6.36925721416675));
#15069=CARTESIAN_POINT('Ctrl Pts',(13.7465187613193,-12.6008409910269,6.59465188812854));
#15070=CARTESIAN_POINT('Ctrl Pts',(14.2941137583008,-13.2044623836355,6.68481335297615));
#15071=CARTESIAN_POINT('Ctrl Pts',(14.8417087552823,-13.8080839907189,6.77500635669625));
#15072=CARTESIAN_POINT('Ctrl Pts',(15.3208543776412,-14.3362528301216,6.85391541259334));
#15073=CARTESIAN_POINT('Ctrl Pts',(15.5946518761319,-14.6380635126529,6.89899411967348));
#15074=CARTESIAN_POINT('Ctrl Pts',(15.7315506253773,-14.7889688752189,6.92153660547059));
#15075=CARTESIAN_POINT('Ctrl Pts',(15.8,-14.8644215375261,6.9328050579454));
#15076=CARTESIAN_POINT('Ctrl Pts',(10.0502525316942,-8.35233000922534,5.94770436886828));
#15077=CARTESIAN_POINT('Ctrl Pts',(11.1454425256572,-9.5384055936255,6.13452948592056));
#15078=CARTESIAN_POINT('Ctrl Pts',(12.3775312688656,-10.8728200811769,6.34492663085593));
#15079=CARTESIAN_POINT('Ctrl Pts',(13.7465187613193,-12.3554217499083,6.57847782979355));
#15080=CARTESIAN_POINT('Ctrl Pts',(14.2941137583008,-12.9484634259519,6.67190108779269));
#15081=CARTESIAN_POINT('Ctrl Pts',(14.8417087552824,-13.541513949349,6.76534871907581));
#15082=CARTESIAN_POINT('Ctrl Pts',(15.3208543776412,-14.0604304019321,6.84710780571679));
#15083=CARTESIAN_POINT('Ctrl Pts',(15.5946518761319,-14.3569506718,6.89381786952799));
#15084=CARTESIAN_POINT('Ctrl Pts',(15.7315506253773,-14.5052116854016,6.91717532204614));
#15085=CARTESIAN_POINT('Ctrl Pts',(15.8,-14.5793414094266,6.92885189186191));
#15086=CARTESIAN_POINT('Ctrl Pts',(10.0502525316942,-8.1751443698686,5.91814205125966));
#15087=CARTESIAN_POINT('Ctrl Pts',(11.1454425256572,-9.34066488658195,6.11093026523681));
#15088=CARTESIAN_POINT('Ctrl Pts',(12.3775312688656,-10.6518240329443,6.32804641946555));
#15089=CARTESIAN_POINT('Ctrl Pts',(13.7465187613193,-12.1087200255634,6.56905244176938));
#15090=CARTESIAN_POINT('Ctrl Pts',(14.2941137583008,-12.6914777697296,6.66545776271567));
#15091=CARTESIAN_POINT('Ctrl Pts',(14.8417087552823,-13.2742297865971,6.76188862893655));
#15092=CARTESIAN_POINT('Ctrl Pts',(15.3208543776412,-13.7841395850464,6.84625768114735));
#15093=CARTESIAN_POINT('Ctrl Pts',(15.5946518761319,-14.0755188249216,6.89445870116997));
#15094=CARTESIAN_POINT('Ctrl Pts',(15.7315506253773,-14.2212078760573,6.9185617481891));
#15095=CARTESIAN_POINT('Ctrl Pts',(15.8,-14.2940529083518,6.93061101156267));
#15096=CARTESIAN_POINT('Ctrl Pts',(10.0502525316942,-7.90144264462466,5.8943312499999));
#15097=CARTESIAN_POINT('Ctrl Pts',(11.1454425256572,-9.03654403267794,6.09882926548584));
#15098=CARTESIAN_POINT('Ctrl Pts',(12.3775312688656,-10.3136205759385,6.32895925304843));
#15099=CARTESIAN_POINT('Ctrl Pts',(13.7465187613193,-11.7325052253954,6.58458807992399));
#15100=CARTESIAN_POINT('Ctrl Pts',(14.2941137583008,-12.3000601956136,6.68684049565601));
#15101=CARTESIAN_POINT('Ctrl Pts',(14.8417087552823,-12.86762490695,6.7891006747503));
#15102=CARTESIAN_POINT('Ctrl Pts',(15.3208543776411,-13.364240995629,6.87857591366296));
#15103=CARTESIAN_POINT('Ctrl Pts',(15.5946518761319,-13.6480178551891,6.92970162298621));
#15104=CARTESIAN_POINT('Ctrl Pts',(15.7315506253773,-13.7899072524002,6.95526524865974));
#15105=CARTESIAN_POINT('Ctrl Pts',(15.8,-13.8608510891535,6.96804637462761));
#15106=CARTESIAN_POINT('Ctrl Pts',(10.0502525316942,-7.66237562613099,5.80163007173558));
#15107=CARTESIAN_POINT('Ctrl Pts',(11.1454425256572,-8.76621669669801,6.00977287125004));
#15108=CARTESIAN_POINT('Ctrl Pts',(12.3775312688656,-10.008064757174,6.24400287259235));
#15109=CARTESIAN_POINT('Ctrl Pts',(13.7465187613193,-11.3878685250288,6.50418764618811));
#15110=CARTESIAN_POINT('Ctrl Pts',(14.2941137583008,-11.9397903730643,6.60826243593386));
#15111=CARTESIAN_POINT('Ctrl Pts',(14.8417087552823,-12.4917152115347,6.71234494803684));
#15112=CARTESIAN_POINT('Ctrl Pts',(15.3208543776411,-12.9746485138656,6.80341474110257));
#15113=CARTESIAN_POINT('Ctrl Pts',(15.5946518761319,-13.2506092458454,6.85545164006593));
#15114=CARTESIAN_POINT('Ctrl Pts',(15.7315506253773,-13.388589908828,6.88147085648712));
#15115=CARTESIAN_POINT('Ctrl Pts',(15.8,-13.4575799757384,6.89447978145678));
#15116=CARTESIAN_POINT('Ctrl Pts',(10.0502525316942,-7.44593237535689,5.68351040711504));
#15117=CARTESIAN_POINT('Ctrl Pts',(11.1454425256572,-8.51992624992032,5.89012315163304));
#15118=CARTESIAN_POINT('Ctrl Pts',(12.3775312688656,-9.72815762348205,6.12263633930509));
#15119=CARTESIAN_POINT('Ctrl Pts',(13.7465187613194,-11.0706489050023,6.38090895110341));
#15120=CARTESIAN_POINT('Ctrl Pts',(14.2941137583009,-11.60764526865,6.4842189332274));
#15121=CARTESIAN_POINT('Ctrl Pts',(14.8417087552824,-12.1446403255654,6.58753713858487));
#15122=CARTESIAN_POINT('Ctrl Pts',(15.3208543776412,-12.6145114073305,6.6779380072571));
#15123=CARTESIAN_POINT('Ctrl Pts',(15.594651876132,-12.8830096730692,6.72959247024461));
#15124=CARTESIAN_POINT('Ctrl Pts',(15.7315506253773,-13.0172586761616,6.755420518422));
#15125=CARTESIAN_POINT('Ctrl Pts',(15.8,-13.0843832933218,6.76833381495438));
#15126=CARTESIAN_POINT('Ctrl Pts',(10.0502525316942,-7.34913449516209,5.60747221894231));
#15127=CARTESIAN_POINT('Ctrl Pts',(11.1454425256572,-8.40845336995523,5.81105284226644));
#15128=CARTESIAN_POINT('Ctrl Pts',(12.3775312688656,-9.60029668798142,6.04008639989118));
#15129=CARTESIAN_POINT('Ctrl Pts',(13.7465187613193,-10.9244551954278,6.29456266363366));
#15130=CARTESIAN_POINT('Ctrl Pts',(14.2941137583009,-11.4541199893924,6.3963532371211));
#15131=CARTESIAN_POINT('Ctrl Pts',(14.8417087552824,-11.9837969855611,6.49814440704391));
#15132=CARTESIAN_POINT('Ctrl Pts',(15.3208543776412,-12.4472605569962,6.58721149497458));
#15133=CARTESIAN_POINT('Ctrl Pts',(15.5946518761319,-12.7120921703849,6.63810674341679));
#15134=CARTESIAN_POINT('Ctrl Pts',(15.7315506253773,-12.8445091889311,6.66355442687238));
#15135=CARTESIAN_POINT('Ctrl Pts',(15.8,-12.9107166186057,6.67627821583014));
#15136=CARTESIAN_POINT('Ctrl Pts',(10.0502525316942,-7.28928030147641,5.55043285230422));
#15137=CARTESIAN_POINT('Ctrl Pts',(11.1454425256572,-8.33905665452735,5.75098891959401));
#15138=CARTESIAN_POINT('Ctrl Pts',(12.3775312688656,-9.52005505170966,5.97661449529503));
#15139=CARTESIAN_POINT('Ctrl Pts',(13.7465187613193,-10.8322754930233,6.22730957940728));
#15140=CARTESIAN_POINT('Ctrl Pts',(14.2941137583009,-11.3571636695488,6.32758761305217));
#15141=CARTESIAN_POINT('Ctrl Pts',(14.8417087552824,-11.8820518460743,6.42786564669707));
#15142=CARTESIAN_POINT('Ctrl Pts',(15.3208543776412,-12.3413290005341,6.51560892613635));
#15143=CARTESIAN_POINT('Ctrl Pts',(15.5946518761319,-12.6037730887968,6.56574794295881));
#15144=CARTESIAN_POINT('Ctrl Pts',(15.7315506253773,-12.7349951329282,6.59081745137003));
#15145=CARTESIAN_POINT('Ctrl Pts',(15.8,-12.8006061549939,6.60335220557564));
#15146=CARTESIAN_POINT('Ctrl Pts',(15.8,-12.8370600702028,6.62691983743441));
#15147=CARTESIAN_POINT('Ctrl Pts',(15.8,-12.8297280642598,6.62229417791417));
#15148=CARTESIAN_POINT('Ctrl Pts',(15.8,-12.8224166748639,6.61762457479065));
#15149=CARTESIAN_POINT('Ctrl Pts',(15.8,-12.8151258955788,6.61291104065239));
#15150=CARTESIAN_POINT('Ctrl Pts',(15.8,-12.8078557223109,6.60815358414732));
#15151=CARTESIAN_POINT('Ctrl Pts',(15.8,-12.8006061549939,6.60335220557564));
#15152=CARTESIAN_POINT('Origin',(15.8,-13.950492764499,5.67212567669951));
#15153=CARTESIAN_POINT('Ctrl Pts',(10.0502525316942,-7.13578365451838,8.05467776187827));
#15154=CARTESIAN_POINT('Ctrl Pts',(11.1454425256572,-8.29974860990865,8.52471396348012));
#15155=CARTESIAN_POINT('Ctrl Pts',(12.3775312688656,-9.6092091847227,9.05350469028219));
#15156=CARTESIAN_POINT('Ctrl Pts',(13.7465187613193,-11.0641653789605,9.6410499422845));
#15157=CARTESIAN_POINT('Ctrl Pts',(14.2941137583009,-11.6461478566557,9.87606804308543));
#15158=CARTESIAN_POINT('Ctrl Pts',(14.8417087552824,-12.2281303343508,10.1110861438864));
#15159=CARTESIAN_POINT('Ctrl Pts',(15.3208543776412,-12.737365002334,10.3167269820872));
#15160=CARTESIAN_POINT('Ctrl Pts',(15.5946518761319,-13.0283562411816,10.4342360324876));
#15161=CARTESIAN_POINT('Ctrl Pts',(15.7315506253773,-13.1738518606054,10.4929905576879));
#15162=CARTESIAN_POINT('Ctrl Pts',(15.8,-13.2465996703173,10.522367820288));
#15163=CARTESIAN_POINT('Ctrl Pts',(10.0502525316942,-6.89902655578542,8.19339868393687));
#15164=CARTESIAN_POINT('Ctrl Pts',(11.1454425256572,-8.04889405860839,8.68853919251131));
#15165=CARTESIAN_POINT('Ctrl Pts',(12.3775312688656,-9.34238794408146,9.24602752966092));
#15166=CARTESIAN_POINT('Ctrl Pts',(13.7465187613193,-10.779712402918,9.86499535005157));
#15167=CARTESIAN_POINT('Ctrl Pts',(14.2941137583009,-11.354640872798,10.1125880646808));
#15168=CARTESIAN_POINT('Ctrl Pts',(14.8417087552824,-11.9295571981554,10.3602324253388));
#15169=CARTESIAN_POINT('Ctrl Pts',(15.3208543776412,-12.4326127553978,10.5769051976768));
#15170=CARTESIAN_POINT('Ctrl Pts',(15.5946518761319,-12.7200777462785,10.7006983402633));
#15171=CARTESIAN_POINT('Ctrl Pts',(15.7315506253773,-12.8638090371883,10.7626000339661));
#15172=CARTESIAN_POINT('Ctrl Pts',(15.8,-12.9356757561148,10.793546315752));
#15173=CARTESIAN_POINT('Ctrl Pts',(10.0502525316942,-6.51604789180993,8.36661813687798));
#15174=CARTESIAN_POINT('Ctrl Pts',(11.1454425256572,-7.63881390938367,8.8990008542554));
#15175=CARTESIAN_POINT('Ctrl Pts',(12.3775312688656,-8.90205445633838,9.49738068383039));
#15176=CARTESIAN_POINT('Ctrl Pts',(13.7465187613194,-10.3055239107478,10.1628080503653));
#15177=CARTESIAN_POINT('Ctrl Pts',(14.2941137583009,-10.8669132727127,10.4289722391039));
#15178=CARTESIAN_POINT('Ctrl Pts',(14.8417087552824,-11.4283172433782,10.6950739523901));
#15179=CARTESIAN_POINT('Ctrl Pts',(15.3208543776412,-11.9195411796877,10.9279323587878));
#15180=CARTESIAN_POINT('Ctrl Pts',(15.594651876132,-12.2002349513456,11.0610183419671));
#15181=CARTESIAN_POINT('Ctrl Pts',(15.7315506253773,-12.3405832861097,11.1275551370522));
#15182=CARTESIAN_POINT('Ctrl Pts',(15.8,-12.4107561622081,11.1608290568883));
#15183=CARTESIAN_POINT('Ctrl Pts',(10.0502525316942,-6.25935291859365,8.32768215464935));
#15184=CARTESIAN_POINT('Ctrl Pts',(11.1454425256572,-7.35179456409855,8.87221159590508));
#15185=CARTESIAN_POINT('Ctrl Pts',(12.3775312688656,-8.58070593097969,9.48507728715608));
#15186=CARTESIAN_POINT('Ctrl Pts',(13.7465187613193,-9.94625006691877,10.1657641132886));
#15187=CARTESIAN_POINT('Ctrl Pts',(14.2941137583008,-10.4924666723322,10.4380421577189));
#15188=CARTESIAN_POINT('Ctrl Pts',(14.8417087552823,-11.0386735802612,10.7103508393265));
#15189=CARTESIAN_POINT('Ctrl Pts',(15.3208543776411,-11.5166076371098,10.9486114186505));
#15190=CARTESIAN_POINT('Ctrl Pts',(15.5946518761319,-11.7897165434404,11.0847485338421));
#15191=CARTESIAN_POINT('Ctrl Pts',(15.7315506253773,-11.9262700347798,11.1528201301259));
#15192=CARTESIAN_POINT('Ctrl Pts',(15.8,-11.9945476376238,11.1868532202043));
#15193=CARTESIAN_POINT('Ctrl Pts',(10.0502525316942,-6.10559301495173,8.23761851725689));
#15194=CARTESIAN_POINT('Ctrl Pts',(11.1454425256572,-7.17588579216885,8.78181727442991));
#15195=CARTESIAN_POINT('Ctrl Pts',(12.3775312688656,-8.37997276877534,9.39427431712614));
#15196=CARTESIAN_POINT('Ctrl Pts',(13.7465187613193,-9.71783944471699,10.0745443941304));
#15197=CARTESIAN_POINT('Ctrl Pts',(14.2941137583009,-10.2529862083793,10.3466552894421));
#15198=CARTESIAN_POINT('Ctrl Pts',(14.8417087552824,-10.7881338344522,10.61879266668));
#15199=CARTESIAN_POINT('Ctrl Pts',(15.3208543776412,-11.2563877393682,10.856904645461));
#15200=CARTESIAN_POINT('Ctrl Pts',(15.5946518761319,-11.5239610675182,10.9929584447386));
#15201=CARTESIAN_POINT('Ctrl Pts',(15.7315506253773,-11.6577478171298,11.060987970935));
#15202=CARTESIAN_POINT('Ctrl Pts',(15.8,-11.7246411157058,11.0950003932583));
#15203=CARTESIAN_POINT('Ctrl Pts',(10.0502525316942,-5.94621492062453,8.15474945546092));
#15204=CARTESIAN_POINT('Ctrl Pts',(11.1454425256572,-6.99511596848632,8.69826758958589));
#15205=CARTESIAN_POINT('Ctrl Pts',(12.3775312688656,-8.17501015002259,9.30992859260386));
#15206=CARTESIAN_POINT('Ctrl Pts',(13.7465187613193,-9.48612538727718,9.98934507962172));
#15207=CARTESIAN_POINT('Ctrl Pts',(14.2941137583008,-10.0105700158496,10.2611141666576));
#15208=CARTESIAN_POINT('Ctrl Pts',(14.8417087552823,-10.535001088446,10.532906293941));
#15209=CARTESIAN_POINT('Ctrl Pts',(15.3208543776412,-10.9938824879741,10.7707172481292));
#15210=CARTESIAN_POINT('Ctrl Pts',(15.5946518761319,-11.2561056460575,10.9066003574976));
#15211=CARTESIAN_POINT('Ctrl Pts',(15.7315506253773,-11.3872158805765,10.9745441973833));
#15212=CARTESIAN_POINT('Ctrl Pts',(15.8,-11.4527721960679,11.0085140807661));
#15213=CARTESIAN_POINT('Ctrl Pts',(10.0502525316942,-5.69326714724858,8.04752551167497));
#15214=CARTESIAN_POINT('Ctrl Pts',(11.1454425256572,-6.70961935691121,8.59278030111935));
#15215=CARTESIAN_POINT('Ctrl Pts',(12.3775312688656,-7.85307681747465,9.20628631668585));
#15216=CARTESIAN_POINT('Ctrl Pts',(13.7465187613193,-9.12352275260843,9.8878635484672));
#15217=CARTESIAN_POINT('Ctrl Pts',(14.2941137583008,-9.63170187793887,10.1604955992679));
#15218=CARTESIAN_POINT('Ctrl Pts',(14.8417087552824,-10.1398879487016,10.4331383564046));
#15219=CARTESIAN_POINT('Ctrl Pts',(15.3208543776412,-10.5845486031013,10.6716974431005));
#15220=CARTESIAN_POINT('Ctrl Pts',(15.5946518761319,-10.8386377334453,10.8080128020807));
#15221=CARTESIAN_POINT('Ctrl Pts',(15.7315506253773,-10.9656829874862,10.8761715434576));
#15222=CARTESIAN_POINT('Ctrl Pts',(15.8,-11.0292050005901,10.9102499677978));
#15223=CARTESIAN_POINT('Ctrl Pts',(10.0502525316942,-5.49454791241253,7.88548479029562));
#15224=CARTESIAN_POINT('Ctrl Pts',(11.1454425256572,-6.48004349322277,8.42454600598801));
#15225=CARTESIAN_POINT('Ctrl Pts',(12.3775312688655,-7.58873003819356,9.03106484753224));
#15226=CARTESIAN_POINT('Ctrl Pts',(13.7465187613193,-8.82059988637913,9.70489831419833));
#15227=CARTESIAN_POINT('Ctrl Pts',(14.2941137583008,-9.31334787493982,9.97443262085556));
#15228=CARTESIAN_POINT('Ctrl Pts',(14.8417087552823,-9.80609631914575,10.2439754326772));
#15229=CARTESIAN_POINT('Ctrl Pts',(15.3208543776411,-10.237251066285,10.4798227509908));
#15230=CARTESIAN_POINT('Ctrl Pts',(15.5946518761319,-10.4836250322036,10.614589374912));
#15231=CARTESIAN_POINT('Ctrl Pts',(15.7315506253773,-10.6068120603551,10.6819735304405));
#15232=CARTESIAN_POINT('Ctrl Pts',(15.8,-10.6684055341557,10.7156648564213));
#15233=CARTESIAN_POINT('Ctrl Pts',(10.0502525316942,-5.32519947010611,7.70626127860213));
#15234=CARTESIAN_POINT('Ctrl Pts',(11.1454425256572,-6.28278149366022,8.23464403472029));
#15235=CARTESIAN_POINT('Ctrl Pts',(12.3775312688656,-7.36002740501521,8.82914182271552));
#15236=CARTESIAN_POINT('Ctrl Pts',(13.7465187613194,-8.55700179652725,9.48962649341726));
#15237=CARTESIAN_POINT('Ctrl Pts',(14.2941137583009,-9.03579113757913,9.7538211861417));
#15238=CARTESIAN_POINT('Ctrl Pts',(14.8417087552824,-9.5145766369121,10.0180235007137));
#15239=CARTESIAN_POINT('Ctrl Pts',(15.3208543776412,-9.93351514221373,10.2491981583259));
#15240=CARTESIAN_POINT('Ctrl Pts',(15.594651876132,-10.172910051869,10.3812950302632));
#15241=CARTESIAN_POINT('Ctrl Pts',(15.7315506253773,-10.2926071256634,10.4473442221897));
#15242=CARTESIAN_POINT('Ctrl Pts',(15.8,-10.3524560021355,10.4803681444471));
#15243=CARTESIAN_POINT('Ctrl Pts',(10.0502525316942,-5.25663803961482,7.60403044672135));
#15244=CARTESIAN_POINT('Ctrl Pts',(11.1454425256572,-6.20120028598869,8.12499465989843));
#15245=CARTESIAN_POINT('Ctrl Pts',(12.3775312688656,-7.26393484617381,8.71111815506916));
#15246=CARTESIAN_POINT('Ctrl Pts',(13.7465187613193,-8.44464710847935,9.36232701259537));
#15247=CARTESIAN_POINT('Ctrl Pts',(14.2941137583009,-8.91693326542987,9.62281103116557));
#15248=CARTESIAN_POINT('Ctrl Pts',(14.8417087552824,-9.38923099717744,9.88329944620756));
#15249=CARTESIAN_POINT('Ctrl Pts',(15.3208543776412,-9.80248791688055,10.1112254436565));
#15250=CARTESIAN_POINT('Ctrl Pts',(15.5946518761319,-10.0386302748779,10.2414671792814));
#15251=CARTESIAN_POINT('Ctrl Pts',(15.7315506253773,-10.1567026019,10.3065884831493));
#15252=CARTESIAN_POINT('Ctrl Pts',(15.8,-10.2157377422983,10.3391487464728));
#15253=CARTESIAN_POINT('Ctrl Pts',(10.0502525316942,-5.21733945232202,7.53128682236137));
#15254=CARTESIAN_POINT('Ctrl Pts',(11.1454425256572,-6.15376086042613,8.04642571042556));
#15255=CARTESIAN_POINT('Ctrl Pts',(12.3775312688656,-7.20723494454326,8.62595695949777));
#15256=CARTESIAN_POINT('Ctrl Pts',(13.7465187613193,-8.3777617046734,9.269880569578));
#15257=CARTESIAN_POINT('Ctrl Pts',(14.2941137583009,-8.84597240872545,9.52745001361009));
#15258=CARTESIAN_POINT('Ctrl Pts',(14.8417087552824,-9.31418311277751,9.78501945764219));
#15259=CARTESIAN_POINT('Ctrl Pts',(15.3208543776412,-9.72386747882306,10.0103927211703));
#15260=CARTESIAN_POINT('Ctrl Pts',(15.5946518761319,-9.95797283084909,10.1391774431863));
#15261=CARTESIAN_POINT('Ctrl Pts',(15.7315506253773,-10.0750255068621,10.2035698041943));
#15262=CARTESIAN_POINT('Ctrl Pts',(15.8,-10.1335518448686,10.2357659846983));
#15263=CARTESIAN_POINT('Ctrl Pts',(15.8,-10.160938779711,10.2694450138623));
#15264=CARTESIAN_POINT('Ctrl Pts',(15.8,-10.1553950350833,10.2627800357942));
#15265=CARTESIAN_POINT('Ctrl Pts',(15.8,-10.1498844772774,10.2560796357392));
#15266=CARTESIAN_POINT('Ctrl Pts',(15.8,-10.1444070962816,10.2493438236809));
#15267=CARTESIAN_POINT('Ctrl Pts',(15.8,-10.1389628855307,10.242572606579));
#15268=CARTESIAN_POINT('Ctrl Pts',(15.8,-10.1335518448686,10.2357659846983));
#15269=CARTESIAN_POINT('Origin',(15.8,-11.5149238208745,9.70545143020505));
#15270=CARTESIAN_POINT('Ctrl Pts',(10.0502525316942,-4.29750123086779,9.86553218952113));
#15271=CARTESIAN_POINT('Ctrl Pts',(11.9668350211294,-5.98055897313701,11.2772850923971));
#15272=CARTESIAN_POINT('Ctrl Pts',(13.8834175105647,-7.66361671540623,12.689037995273));
#15273=CARTESIAN_POINT('Ctrl Pts',(15.8,-9.34667445767544,14.1007908981489));
#15274=CARTESIAN_POINT('Ctrl Pts',(10.0502525316942,-4.02946472694721,9.92430165934405));
#15275=CARTESIAN_POINT('Ctrl Pts',(11.9668350211294,-5.67542688932036,11.3702854403574));
#15276=CARTESIAN_POINT('Ctrl Pts',(13.8834175105647,-7.32120731702057,12.8166324188796));
#15277=CARTESIAN_POINT('Ctrl Pts',(15.8,-8.96716947939372,14.262616199893));
#15278=CARTESIAN_POINT('Ctrl Pts',(10.0502525316942,-3.61211062987325,9.97045860619055));
#15279=CARTESIAN_POINT('Ctrl Pts',(11.9668350211294,-5.19299729643612,11.4635526451079));
#15280=CARTESIAN_POINT('Ctrl Pts',(13.8834175105647,-6.7741160599007,12.956112555571));
#15281=CARTESIAN_POINT('Ctrl Pts',(15.8,-8.35500272646358,14.4492065944883));
#15282=CARTESIAN_POINT('Ctrl Pts',(10.0502525316942,-3.40259706500424,9.86609404202409));
#15283=CARTESIAN_POINT('Ctrl Pts',(11.9668350211294,-4.93192196434907,11.3629139742223));
#15284=CARTESIAN_POINT('Ctrl Pts',(13.8834175105647,-6.46129704742021,12.8596985741914));
#15285=CARTESIAN_POINT('Ctrl Pts',(15.8,-7.99062194676504,14.3565185063896));
#15286=CARTESIAN_POINT('Ctrl Pts',(10.0502525316942,-3.30601090928165,9.77087387154055));
#15287=CARTESIAN_POINT('Ctrl Pts',(11.9668350211295,-4.80688444200922,11.2600017151873));
#15288=CARTESIAN_POINT('Ctrl Pts',(13.8834175105647,-6.30755492143114,12.7494883087275));
#15289=CARTESIAN_POINT('Ctrl Pts',(15.8,-7.8084284541587,14.2386161523743));
#15290=CARTESIAN_POINT('Ctrl Pts',(10.0502525316942,-3.24522078037662,9.7053049496755));
#15291=CARTESIAN_POINT('Ctrl Pts',(11.9668350211294,-4.72781700580774,11.1883166806211));
#15292=CARTESIAN_POINT('Ctrl Pts',(13.8834175105647,-6.21037804061049,12.6715703878316));
#15293=CARTESIAN_POINT('Ctrl Pts',(15.8,-7.69297426604161,14.1545821187772));
#15294=CARTESIAN_POINT('Ctrl Pts',(10.0502525316942,-3.13558852137588,9.59290229251195));
#15295=CARTESIAN_POINT('Ctrl Pts',(11.9668350211294,-4.58744122478927,11.0646742694966));
#15296=CARTESIAN_POINT('Ctrl Pts',(13.8834175105647,-6.03905717649214,12.5366026187688));
#15297=CARTESIAN_POINT('Ctrl Pts',(15.8,-7.49090987990553,14.0083745957535));
#15298=CARTESIAN_POINT('Ctrl Pts',(10.0502525316942,-2.92757116168118,9.41310152025599));
#15299=CARTESIAN_POINT('Ctrl Pts',(11.9668350211294,-4.32424671627921,10.8702564567215));
#15300=CARTESIAN_POINT('Ctrl Pts',(13.8834175105647,-5.72097159497831,12.3275956094625));
#15301=CARTESIAN_POINT('Ctrl Pts',(15.8,-7.11764714957633,13.784750545928));
#15302=CARTESIAN_POINT('Ctrl Pts',(10.0502525316942,-2.78894862571459,9.19740926566326));
#15303=CARTESIAN_POINT('Ctrl Pts',(11.9668350211294,-4.13765656795514,10.6275127538178));
#15304=CARTESIAN_POINT('Ctrl Pts',(13.8834175105647,-5.48632659127462,12.0577280234798));
#15305=CARTESIAN_POINT('Ctrl Pts',(15.8,-6.83503453351517,13.4878315116343));
#15306=CARTESIAN_POINT('Ctrl Pts',(10.0502525316942,-2.6831512960299,8.97469639188219));
#15307=CARTESIAN_POINT('Ctrl Pts',(11.9668350211294,-3.99115284441713,10.3719655284903));
#15308=CARTESIAN_POINT('Ctrl Pts',(13.8834175105648,-5.29909475352164,11.7692966119437));
#15309=CARTESIAN_POINT('Ctrl Pts',(15.8,-6.60709630190888,13.1665657485518));
#15310=CARTESIAN_POINT('Ctrl Pts',(10.0502525316942,-2.64958522759923,8.85625319397989));
#15311=CARTESIAN_POINT('Ctrl Pts',(11.9668350211294,-3.93994688562079,10.2341088589535));
#15312=CARTESIAN_POINT('Ctrl Pts',(13.8834175105647,-5.23040962052304,11.612095695752));
#15313=CARTESIAN_POINT('Ctrl Pts',(15.8,-6.5207712785446,12.9899513607256));
#15314=CARTESIAN_POINT('Ctrl Pts',(10.0502525316942,-2.63468906623289,8.77492596468499));
#15315=CARTESIAN_POINT('Ctrl Pts',(11.9668350211294,-3.91464433600868,10.1386945339445));
#15316=CARTESIAN_POINT('Ctrl Pts',(13.8834175105647,-5.19459960578447,11.5024631032041));
#15317=CARTESIAN_POINT('Ctrl Pts',(15.8,-6.47455487556026,12.8662316724636));
#15318=CARTESIAN_POINT('Ctrl Pts',(15.8,-6.49019400603777,12.9067253609027));
#15319=CARTESIAN_POINT('Ctrl Pts',(15.8,-6.48698118307512,12.8986734787776));
#15320=CARTESIAN_POINT('Ctrl Pts',(15.8,-6.48381086865141,12.890598163633));
#15321=CARTESIAN_POINT('Ctrl Pts',(15.8,-6.48068305016014,12.8824994218701));
#15322=CARTESIAN_POINT('Ctrl Pts',(15.8,-6.47759771920651,12.874377258079));
#15323=CARTESIAN_POINT('Ctrl Pts',(15.8,-6.47455487556026,12.8662316724636));
#15324=CARTESIAN_POINT('Origin',(15.8,-7.95219390447097,12.7887399758658));
#15325=CARTESIAN_POINT('Ctrl Pts',(10.0502525316942,-1.03854944428814,10.7106795892491));
#15326=CARTESIAN_POINT('Ctrl Pts',(11.9668350211294,-2.20297683852746,12.5734298318033));
#15327=CARTESIAN_POINT('Ctrl Pts',(13.8834175105647,-3.36740423276678,14.4361800743576));
#15328=CARTESIAN_POINT('Ctrl Pts',(15.8,-4.5318316270061,16.2989303169119));
#15329=CARTESIAN_POINT('Ctrl Pts',(10.0502525316942,-0.765470815703814,
10.6837448416591));
#15330=CARTESIAN_POINT('Ctrl Pts',(11.9668350211294,-1.88404029388038,12.5675874193204));
#15331=CARTESIAN_POINT('Ctrl Pts',(13.8834175105647,-3.00232469790949,14.4517192592367));
#15332=CARTESIAN_POINT('Ctrl Pts',(15.8,-4.12089417608606,16.335561836898));
#15333=CARTESIAN_POINT('Ctrl Pts',(10.0502525316942,-0.354275884655605,
10.5986742216641));
#15334=CARTESIAN_POINT('Ctrl Pts',(11.9668350211295,-1.39639701818897,12.5072118829665));
#15335=CARTESIAN_POINT('Ctrl Pts',(13.8834175105647,-2.43890221878171,14.4153151096237));
#15336=CARTESIAN_POINT('Ctrl Pts',(15.8,-3.48102335231507,16.3238527709261));
#15337=CARTESIAN_POINT('Ctrl Pts',(10.0502525316942,-0.187261072828498,
10.4346757823309));
#15338=CARTESIAN_POINT('Ctrl Pts',(11.9668350211295,-1.17919268731443,12.3308235163868));
#15339=CARTESIAN_POINT('Ctrl Pts',(13.8834175105647,-2.17117887432507,14.2269575174279));
#15340=CARTESIAN_POINT('Ctrl Pts',(15.8,-3.163110488811,16.1231052514838));
#15341=CARTESIAN_POINT('Ctrl Pts',(10.0502525316942,-0.124824203483033,
10.3142698682631));
#15342=CARTESIAN_POINT('Ctrl Pts',(11.9668350211295,-1.09207394643473,12.1943100355803));
#15343=CARTESIAN_POINT('Ctrl Pts',(13.8834175105647,-2.05901454824882,14.0746341437949));
#15344=CARTESIAN_POINT('Ctrl Pts',(15.8,-3.02626429120052,15.9546743111122));
#15345=CARTESIAN_POINT('Ctrl Pts',(10.0502525316942,-0.0872711810328558,
10.2331249635989));
#15346=CARTESIAN_POINT('Ctrl Pts',(11.9668350211295,-1.03902815454411,12.1017003635113));
#15347=CARTESIAN_POINT('Ctrl Pts',(13.8834175105647,-1.99067177195528,13.9705005205662));
#15348=CARTESIAN_POINT('Ctrl Pts',(15.8,-2.94242874546654,15.8390759204785));
#15349=CARTESIAN_POINT('Ctrl Pts',(10.0502525316942,-0.0177390798696548,
10.09234540735));
#15350=CARTESIAN_POINT('Ctrl Pts',(11.9668350211294,-0.943730501418606,
11.9407308952458));
#15351=CARTESIAN_POINT('Ctrl Pts',(13.8834175105647,-1.86944300220408,13.789197555515));
#15352=CARTESIAN_POINT('Ctrl Pts',(15.8,-2.79543442375304,15.6375830434108));
#15353=CARTESIAN_POINT('Ctrl Pts',(10.0502525316942,0.124535428292433,9.85706386916291));
#15354=CARTESIAN_POINT('Ctrl Pts',(11.9668350211295,-0.753496320252986,
11.6744970487389));
#15355=CARTESIAN_POINT('Ctrl Pts',(13.8834175105647,-1.63151416409049,13.4921256030567));
#15356=CARTESIAN_POINT('Ctrl Pts',(15.8,-2.50954591263591,15.3095587826327));
#15357=CARTESIAN_POINT('Ctrl Pts',(10.0502525316942,0.189717758784555,9.60909091476054));
#15358=CARTESIAN_POINT('Ctrl Pts',(11.9668350211294,-0.651053436707715,
11.3859738307471));
#15359=CARTESIAN_POINT('Ctrl Pts',(13.8834175105647,-1.49175101418763,13.1629551482145));
#15360=CARTESIAN_POINT('Ctrl Pts',(15.8,-2.3325222096799,14.9398380642011));
#15361=CARTESIAN_POINT('Ctrl Pts',(10.0502525316942,0.221513186022213,9.36458479377687));
#15362=CARTESIAN_POINT('Ctrl Pts',(11.9668350211294,-0.590690300968109,
11.0976614182865));
#15363=CARTESIAN_POINT('Ctrl Pts',(13.8834175105648,-1.40281548080796,12.8307816497324));
#15364=CARTESIAN_POINT('Ctrl Pts',(15.8,-2.21501896779828,14.563858274242));
#15365=CARTESIAN_POINT('Ctrl Pts',(10.0502525316942,0.21682744723956,9.24156417346731));
#15366=CARTESIAN_POINT('Ctrl Pts',(11.9668350211294,-0.58459859972662,10.9507264633732));
#15367=CARTESIAN_POINT('Ctrl Pts',(13.8834175105647,-1.38608024219576,12.6600447395717));
#15368=CARTESIAN_POINT('Ctrl Pts',(15.8,-2.18750628916194,14.3692070294775));
#15369=CARTESIAN_POINT('Ctrl Pts',(10.0502525316942,0.205863042617261,9.15961421508102));
#15370=CARTESIAN_POINT('Ctrl Pts',(11.9668350211294,-0.590019092973717,
10.8521631299943));
#15371=CARTESIAN_POINT('Ctrl Pts',(13.8834175105647,-1.38590122856469,12.5447120449076));
#15372=CARTESIAN_POINT('Ctrl Pts',(15.8,-2.18178336415567,14.2372609598209));
#15373=CARTESIAN_POINT('Ctrl Pts',(15.8,-2.18414382321291,14.2806055031745));
#15374=CARTESIAN_POINT('Ctrl Pts',(15.8,-2.18357641541193,14.2719548913156));
#15375=CARTESIAN_POINT('Ctrl Pts',(15.8,-2.18305667683518,14.2632951291918));
#15376=CARTESIAN_POINT('Ctrl Pts',(15.8,-2.18258459351507,14.2546262189952));
#15377=CARTESIAN_POINT('Ctrl Pts',(15.8,-2.18216015604922,14.2459481624974));
#15378=CARTESIAN_POINT('Ctrl Pts',(15.8,-2.18178336415567,14.2372609598209));
#15379=CARTESIAN_POINT('Origin',(15.8,-3.61104784250494,14.6201775482978));
#15380=CARTESIAN_POINT('Ctrl Pts',(10.0502525316942,2.32206279789789,10.5073910450885));
#15381=CARTESIAN_POINT('Ctrl Pts',(11.1454425256572,2.01816863800157,11.7253388222013));
#15382=CARTESIAN_POINT('Ctrl Pts',(12.3775312688656,1.67628770811821,13.0955300714531));
#15383=CARTESIAN_POINT('Ctrl Pts',(13.7465187613194,1.29642000824781,14.617964792844));
#15384=CARTESIAN_POINT('Ctrl Pts',(14.2941137583009,1.14447292829964,15.2269386814004));
#15385=CARTESIAN_POINT('Ctrl Pts',(14.8417087552824,0.992525848351482,15.8359125699568));
#15386=CARTESIAN_POINT('Ctrl Pts',(15.3208543776412,0.859572153396841,16.3687647224436));
#15387=CARTESIAN_POINT('Ctrl Pts',(15.5946518761319,0.78359861342276,16.6732516667218));
#15388=CARTESIAN_POINT('Ctrl Pts',(15.7315506253773,0.74561184343572,16.8254951388609));
#15389=CARTESIAN_POINT('Ctrl Pts',(15.8,0.7266184584422,16.9016168749304));
#15390=CARTESIAN_POINT('Ctrl Pts',(10.0502525316942,2.57345271232945,10.3973886408451));
#15391=CARTESIAN_POINT('Ctrl Pts',(11.1454425256572,2.29815463811993,11.618687280661));
#15392=CARTESIAN_POINT('Ctrl Pts',(12.3775312688656,1.98887116228557,12.9928273987101));
#15393=CARTESIAN_POINT('Ctrl Pts',(13.7465187613193,1.64478997784957,14.519468077176));
#15394=CARTESIAN_POINT('Ctrl Pts',(14.2941137583009,1.50716238874916,15.1301263986154));
#15395=CARTESIAN_POINT('Ctrl Pts',(14.8417087552824,1.36958497392712,15.740805777741));
#15396=CARTESIAN_POINT('Ctrl Pts',(15.3208543776412,1.24918922664557,16.2751437253593));
#15397=CARTESIAN_POINT('Ctrl Pts',(15.5946518761319,1.18037249165619,16.5804716520035));
#15398=CARTESIAN_POINT('Ctrl Pts',(15.7315506253773,1.14596909077302,16.7331376997671));
#15399=CARTESIAN_POINT('Ctrl Pts',(15.8,1.12876296113493,16.8094688647556));
#15400=CARTESIAN_POINT('Ctrl Pts',(10.0502525316942,2.93870070814822,10.1893681184011));
#15401=CARTESIAN_POINT('Ctrl Pts',(11.1454425256572,2.70946206711307,11.4106316171747));
#15402=CARTESIAN_POINT('Ctrl Pts',(12.3775312688656,2.45105312324518,12.7843360022416));
#15403=CARTESIAN_POINT('Ctrl Pts',(13.7465187613194,2.16445481731472,14.310894320163));
#15404=CARTESIAN_POINT('Ctrl Pts',(14.2941137583009,2.04980959621706,14.9215151635443));
#15405=CARTESIAN_POINT('Ctrl Pts',(14.8417087552824,1.93510378473095,15.5321104940175));
#15406=CARTESIAN_POINT('Ctrl Pts',(15.3208543776412,1.83475492870442,16.0663892944466));
#15407=CARTESIAN_POINT('Ctrl Pts',(15.5946518761319,1.77743586902583,16.3717012113088));
#15408=CARTESIAN_POINT('Ctrl Pts',(15.7315506253773,1.74877034151339,16.5243546442885));
#15409=CARTESIAN_POINT('Ctrl Pts',(15.8,1.7344429264487,16.6006836129618));
#15410=CARTESIAN_POINT('Ctrl Pts',(10.0502525316942,3.05808383535425,9.95881139224216));
#15411=CARTESIAN_POINT('Ctrl Pts',(11.1454425256572,2.85649631904974,11.1626816238277));
#15412=CARTESIAN_POINT('Ctrl Pts',(12.3775312688655,2.62997738853437,12.5171248305866));
#15413=CARTESIAN_POINT('Ctrl Pts',(13.7465187613193,2.37801889657081,14.0219712727572));
#15414=CARTESIAN_POINT('Ctrl Pts',(14.2941137583008,2.27723855544496,14.6239108703275));
#15415=CARTESIAN_POINT('Ctrl Pts',(14.8417087552823,2.17648960137064,15.225860952321));
#15416=CARTESIAN_POINT('Ctrl Pts',(15.3208543776411,2.08832456454097,15.7525640332375));
#15417=CARTESIAN_POINT('Ctrl Pts',(15.5946518761319,2.03793255455516,16.0535332175881));
#15418=CARTESIAN_POINT('Ctrl Pts',(15.7315506253773,2.01273965647872,16.2040188475872));
#15419=CARTESIAN_POINT('Ctrl Pts',(15.7999999999999,2.00014043670969,16.2792607370613));
#15420=CARTESIAN_POINT('Ctrl Pts',(10.0502525316942,3.07559947603193,9.78147886731911));
#15421=CARTESIAN_POINT('Ctrl Pts',(11.1454425256572,2.88676320881926,10.9672359168267));
#15422=CARTESIAN_POINT('Ctrl Pts',(12.3775312688655,2.67450622091511,12.3013551830101));
#15423=CARTESIAN_POINT('Ctrl Pts',(13.7465187613193,2.43847871808159,13.7835653267336));
#15424=CARTESIAN_POINT('Ctrl Pts',(14.2941137583008,2.34406982037812,14.3764510158762));
#15425=CARTESIAN_POINT('Ctrl Pts',(14.8417087552823,2.24968252863639,14.9693534649946));
#15426=CARTESIAN_POINT('Ctrl Pts',(15.3208543776412,2.16708696976892,15.4881379273167));
#15427=CARTESIAN_POINT('Ctrl Pts',(15.5946518761319,2.11988125471031,15.7845797896778));
#15428=CARTESIAN_POINT('Ctrl Pts',(15.7315506253773,2.09628053589475,15.9328023798814));
#15429=CARTESIAN_POINT('Ctrl Pts',(15.8,2.08447826919396,16.0069121954756));
#15430=CARTESIAN_POINT('Ctrl Pts',(10.0502525316941,3.10223684531879,9.60383008034198));
#15431=CARTESIAN_POINT('Ctrl Pts',(11.1454425256572,2.92542368552957,10.771880797072));
#15432=CARTESIAN_POINT('Ctrl Pts',(12.3775312688655,2.72674232124833,12.0859609655105));
#15433=CARTESIAN_POINT('Ctrl Pts',(13.7465187613193,2.5057485169523,13.5460266034681));
#15434=CARTESIAN_POINT('Ctrl Pts',(14.2941137583008,2.41735366657091,14.1300531231308));
#15435=CARTESIAN_POINT('Ctrl Pts',(14.8417087552823,2.32898625556579,14.7140823594691));
#15436=CARTESIAN_POINT('Ctrl Pts',(15.3208543776411,2.25165628918294,15.2251071015168));
#15437=CARTESIAN_POINT('Ctrl Pts',(15.5946518761319,2.20745725592094,15.5171202021387));
#15438=CARTESIAN_POINT('Ctrl Pts',(15.7315506253773,2.18536045543708,15.6631270213657));
#15439=CARTESIAN_POINT('Ctrl Pts',(15.8,2.17430963295026,15.7361301911614));
#15440=CARTESIAN_POINT('Ctrl Pts',(10.0502525316942,3.1641697547985,9.33616641898041));
#15441=CARTESIAN_POINT('Ctrl Pts',(11.1454425256572,3.00789330574878,10.4789053528453));
#15442=CARTESIAN_POINT('Ctrl Pts',(12.3775312688656,2.83212323706008,11.7645911992084));
#15443=CARTESIAN_POINT('Ctrl Pts',(13.7465187613193,2.6367816468882,13.1930250082462));
#15444=CARTESIAN_POINT('Ctrl Pts',(14.2941137583008,2.55864547926934,13.7643997282132));
#15445=CARTESIAN_POINT('Ctrl Pts',(14.8417087552823,2.48051412346292,14.3357867368397));
#15446=CARTESIAN_POINT('Ctrl Pts',(15.3208543776412,2.4121476997586,14.8357465708549));
#15447=CARTESIAN_POINT('Ctrl Pts',(15.5946518761319,2.37307933395524,15.1214332106675));
#15448=CARTESIAN_POINT('Ctrl Pts',(15.7315506253773,2.35354562736143,15.2642777469938));
#15449=CARTESIAN_POINT('Ctrl Pts',(15.8,2.34377834929582,15.3356989303604));
#15450=CARTESIAN_POINT('Ctrl Pts',(10.0502525316942,3.14987939962279,9.08015411140619));
#15451=CARTESIAN_POINT('Ctrl Pts',(11.1454425256572,3.00672931552669,10.1942890168299));
#15452=CARTESIAN_POINT('Ctrl Pts',(12.3775312688655,2.84574388114627,11.4477380681646));
#15453=CARTESIAN_POINT('Ctrl Pts',(13.7465187613193,2.66681194224705,12.8404112867165));
#15454=CARTESIAN_POINT('Ctrl Pts',(14.2941137583008,2.59523983509501,13.3974811152093));
#15455=CARTESIAN_POINT('Ctrl Pts',(14.8417087552823,2.52367459367682,13.9545565014729));
#15456=CARTESIAN_POINT('Ctrl Pts',(15.3208543776411,2.46105288517697,14.4419957464976));
#15457=CARTESIAN_POINT('Ctrl Pts',(15.5946518761319,2.42526642923796,14.7205303350335));
#15458=CARTESIAN_POINT('Ctrl Pts',(15.7315506253773,2.40737388088825,14.8597981794497));
#15459=CARTESIAN_POINT('Ctrl Pts',(15.8,2.39842700063224,14.9294316110387));
#15460=CARTESIAN_POINT('Ctrl Pts',(10.0502525316942,3.10442465522081,8.83780343943476));
#15461=CARTESIAN_POINT('Ctrl Pts',(11.1454425256572,2.96904269314958,9.92307916160989));
#15462=CARTESIAN_POINT('Ctrl Pts',(12.3775312688656,2.81681208487056,11.1440266947135));
#15463=CARTESIAN_POINT('Ctrl Pts',(13.7465187613194,2.64759182043347,12.5006225450517));
#15464=CARTESIAN_POINT('Ctrl Pts',(14.2941137583009,2.5799045625987,13.0432610264625));
#15465=CARTESIAN_POINT('Ctrl Pts',(14.8417087552824,2.51222601461465,13.585900959023));
#15466=CARTESIAN_POINT('Ctrl Pts',(15.3208543776412,2.45300459283688,14.0607104514503));
#15467=CARTESIAN_POINT('Ctrl Pts',(15.594651876132,2.41916045348293,14.3320296071118));
#15468=CARTESIAN_POINT('Ctrl Pts',(15.7315506253773,2.40223924596973,14.4676893285878));
#15469=CARTESIAN_POINT('Ctrl Pts',(15.8,2.39377787334028,14.5355190612237));
#15470=CARTESIAN_POINT('Ctrl Pts',(10.0502525316942,3.06201554081689,8.72224646189197));
#15471=CARTESIAN_POINT('Ctrl Pts',(11.1454425256572,2.92828468444751,9.79262845293104));
#15472=CARTESIAN_POINT('Ctrl Pts',(12.3775312688656,2.77780914227504,10.9969124481398));
#15473=CARTESIAN_POINT('Ctrl Pts',(13.7465187613194,2.61064282371592,12.3349000504671));
#15474=CARTESIAN_POINT('Ctrl Pts',(14.2941137583009,2.54377597211689,12.870096284426));
#15475=CARTESIAN_POINT('Ctrl Pts',(14.8417087552824,2.47690579066087,13.4053047729009));
#15476=CARTESIAN_POINT('Ctrl Pts',(15.3208543776412,2.41839541117503,13.8736084123374));
#15477=CARTESIAN_POINT('Ctrl Pts',(15.5946518761319,2.38496218052017,14.1412058111469));
#15478=CARTESIAN_POINT('Ctrl Pts',(15.7315506253773,2.3682452355795,14.2750057235919));
#15479=CARTESIAN_POINT('Ctrl Pts',(15.8,2.35988705705641,14.3419045980318));
#15480=CARTESIAN_POINT('Ctrl Pts',(10.0502525316942,3.02626384252387,8.64769560732005));
#15481=CARTESIAN_POINT('Ctrl Pts',(11.1454425256572,2.89260526381666,9.70806748165927));
#15482=CARTESIAN_POINT('Ctrl Pts',(12.3775312688656,2.74223936277106,10.9009858402909));
#15483=CARTESIAN_POINT('Ctrl Pts',(13.7465187613194,2.57516613938705,12.2264506832149));
#15484=CARTESIAN_POINT('Ctrl Pts',(14.2941137583009,2.50833685003344,12.7566366203845));
#15485=CARTESIAN_POINT('Ctrl Pts',(14.8417087552824,2.44150756067984,13.2868225575541));
#15486=CARTESIAN_POINT('Ctrl Pts',(15.3208543776412,2.38303193249543,13.7507352525775));
#15487=CARTESIAN_POINT('Ctrl Pts',(15.5946518761319,2.34961728781863,14.0158282211623));
#15488=CARTESIAN_POINT('Ctrl Pts',(15.7315506253773,2.33290996548023,14.1483747054547));
#15489=CARTESIAN_POINT('Ctrl Pts',(15.8,2.32455630431103,14.2146479476009));
#15490=CARTESIAN_POINT('Ctrl Pts',(15.8,2.33570557485288,14.2566004799664));
#15491=CARTESIAN_POINT('Ctrl Pts',(15.8,2.33357202566325,14.2481979205348));
#15492=CARTESIAN_POINT('Ctrl Pts',(15.8,2.33139031275994,14.2398013892846));
#15493=CARTESIAN_POINT('Ctrl Pts',(15.8,2.32916045010432,14.2314108839843));
#15494=CARTESIAN_POINT('Ctrl Pts',(15.8,2.32688244718599,14.2230264034132));
#15495=CARTESIAN_POINT('Ctrl Pts',(15.8,2.32455630431103,14.2146479476009));
#15496=CARTESIAN_POINT('Origin',(15.8,1.08357274193521,15.0204902775358));
#15497=CARTESIAN_POINT('Ctrl Pts',(10.0502525316942,5.45537535466284,9.2755658561365));
#15498=CARTESIAN_POINT('Ctrl Pts',(11.1454425256572,5.54272139501843,10.527811485966));
#15499=CARTESIAN_POINT('Ctrl Pts',(12.3775312688656,5.64098569041847,11.9365878195243));
#15500=CARTESIAN_POINT('Ctrl Pts',(13.7465187613193,5.75016824086295,13.5018948568112));
#15501=CARTESIAN_POINT('Ctrl Pts',(14.2941137583009,5.79384126104075,14.1280176717259));
#15502=CARTESIAN_POINT('Ctrl Pts',(14.8417087552824,5.83751428121855,14.7541404866407));
#15503=CARTESIAN_POINT('Ctrl Pts',(15.3208543776412,5.87572817387412,15.3019979496911));
#15504=CARTESIAN_POINT('Ctrl Pts',(15.5946518761319,5.89756468396301,15.6150593571485));
#15505=CARTESIAN_POINT('Ctrl Pts',(15.7315506253773,5.90848293900746,15.7715900608772));
#15506=CARTESIAN_POINT('Ctrl Pts',(15.8,5.91394206652969,15.8498554127416));
#15507=CARTESIAN_POINT('Ctrl Pts',(10.0502525316942,5.66046875858054,9.09326359699885));
#15508=CARTESIAN_POINT('Ctrl Pts',(11.1454425256572,5.77604676609019,10.3398594101876));
#15509=CARTESIAN_POINT('Ctrl Pts',(12.3775312688656,5.90654052031257,11.7423187718539));
#15510=CARTESIAN_POINT('Ctrl Pts',(13.7465187613193,6.05105541408884,13.3005670731329));
#15511=CARTESIAN_POINT('Ctrl Pts',(14.2941137583009,6.10886731837784,13.9238668895967));
#15512=CARTESIAN_POINT('Ctrl Pts',(14.8417087552824,6.16673138983644,14.5471710567224));
#15513=CARTESIAN_POINT('Ctrl Pts',(15.3208543776412,6.2173462055988,15.0925608480022));
#15514=CARTESIAN_POINT('Ctrl Pts',(15.5946518761319,6.24624880770451,15.404210476846));
#15515=CARTESIAN_POINT('Ctrl Pts',(15.7315506253773,6.26070528969668,15.5600357233503));
#15516=CARTESIAN_POINT('Ctrl Pts',(15.8,6.26792891516603,15.6379479616746));
#15517=CARTESIAN_POINT('Ctrl Pts',(10.0502525316942,5.94355560685308,8.78255765938312));
#15518=CARTESIAN_POINT('Ctrl Pts',(11.1454425256572,6.10292787924083,10.0148869038525));
#15519=CARTESIAN_POINT('Ctrl Pts',(12.3775312688656,6.2816544949474,11.4012092316412));
#15520=CARTESIAN_POINT('Ctrl Pts',(13.7465187613194,6.48081852219945,12.9416164381759));
#15521=CARTESIAN_POINT('Ctrl Pts',(14.2941137583009,6.56047693355264,13.5577787105923));
#15522=CARTESIAN_POINT('Ctrl Pts',(14.8417087552824,6.64007218801815,14.1739356301478));
#15523=CARTESIAN_POINT('Ctrl Pts',(15.3208543776412,6.70973770503939,14.7130746018355));
#15524=CARTESIAN_POINT('Ctrl Pts',(15.5946518761319,6.74957096648566,15.0211560817904));
#15525=CARTESIAN_POINT('Ctrl Pts',(15.7315506253773,6.76948132483472,15.1751962901529));
#15526=CARTESIAN_POINT('Ctrl Pts',(15.8,6.77944209185895,15.2522168679322));
#15527=CARTESIAN_POINT('Ctrl Pts',(10.0502525316942,5.9858465900355,8.52639512605654));
#15528=CARTESIAN_POINT('Ctrl Pts',(11.1454425256572,6.16614182963238,9.73363772297169));
#15529=CARTESIAN_POINT('Ctrl Pts',(12.3775312688656,6.36925721416674,11.0917875706281));
#15530=CARTESIAN_POINT('Ctrl Pts',(13.7465187613193,6.59465188812854,12.6008409910269));
#15531=CARTESIAN_POINT('Ctrl Pts',(14.2941137583008,6.68481335297614,13.2044623836355));
#15532=CARTESIAN_POINT('Ctrl Pts',(14.8417087552823,6.77500635669624,13.8080839907189));
#15533=CARTESIAN_POINT('Ctrl Pts',(15.3208543776411,6.85391541259334,14.3362528301216));
#15534=CARTESIAN_POINT('Ctrl Pts',(15.5946518761319,6.89899411967347,14.6380635126529));
#15535=CARTESIAN_POINT('Ctrl Pts',(15.7315506253773,6.92153660547059,14.7889688752189));
#15536=CARTESIAN_POINT('Ctrl Pts',(15.8,6.93280505794539,14.8644215375261));
#15537=CARTESIAN_POINT('Ctrl Pts',(10.0502525316942,5.94770436886827,8.35233000922534));
#15538=CARTESIAN_POINT('Ctrl Pts',(11.1454425256572,6.13452948592055,9.53840559362551));
#15539=CARTESIAN_POINT('Ctrl Pts',(12.3775312688656,6.34492663085592,10.8728200811769));
#15540=CARTESIAN_POINT('Ctrl Pts',(13.7465187613193,6.57847782979354,12.3554217499083));
#15541=CARTESIAN_POINT('Ctrl Pts',(14.2941137583008,6.67190108779269,12.9484634259519));
#15542=CARTESIAN_POINT('Ctrl Pts',(14.8417087552824,6.76534871907581,13.5415139493489));
#15543=CARTESIAN_POINT('Ctrl Pts',(15.3208543776412,6.84710780571679,14.0604304019321));
#15544=CARTESIAN_POINT('Ctrl Pts',(15.5946518761319,6.89381786952799,14.3569506718));
#15545=CARTESIAN_POINT('Ctrl Pts',(15.7315506253773,6.91717532204614,14.5052116854016));
#15546=CARTESIAN_POINT('Ctrl Pts',(15.8,6.92885189186191,14.5793414094266));
#15547=CARTESIAN_POINT('Ctrl Pts',(10.0502525316942,5.91814205125966,8.17514436986861));
#15548=CARTESIAN_POINT('Ctrl Pts',(11.1454425256572,6.1109302652368,9.34066488658196));
#15549=CARTESIAN_POINT('Ctrl Pts',(12.3775312688656,6.32804641946554,10.6518240329443));
#15550=CARTESIAN_POINT('Ctrl Pts',(13.7465187613193,6.56905244176937,12.1087200255634));
#15551=CARTESIAN_POINT('Ctrl Pts',(14.2941137583008,6.66545776271566,12.6914777697296));
#15552=CARTESIAN_POINT('Ctrl Pts',(14.8417087552823,6.76188862893654,13.2742297865971));
#15553=CARTESIAN_POINT('Ctrl Pts',(15.3208543776412,6.84625768114734,13.7841395850464));
#15554=CARTESIAN_POINT('Ctrl Pts',(15.5946518761319,6.89445870116996,14.0755188249216));
#15555=CARTESIAN_POINT('Ctrl Pts',(15.7315506253773,6.91856174818909,14.2212078760573));
#15556=CARTESIAN_POINT('Ctrl Pts',(15.8,6.93061101156266,14.2940529083519));
#15557=CARTESIAN_POINT('Ctrl Pts',(10.0502525316942,5.89433124999992,7.90144264462466));
#15558=CARTESIAN_POINT('Ctrl Pts',(11.1454425256572,6.09882926548586,9.03654403267793));
#15559=CARTESIAN_POINT('Ctrl Pts',(12.3775312688656,6.32895925304843,10.3136205759384));
#15560=CARTESIAN_POINT('Ctrl Pts',(13.7465187613193,6.58458807992398,11.7325052253954));
#15561=CARTESIAN_POINT('Ctrl Pts',(14.2941137583008,6.68684049565601,12.3000601956136));
#15562=CARTESIAN_POINT('Ctrl Pts',(14.8417087552823,6.7891006747503,12.86762490695));
#15563=CARTESIAN_POINT('Ctrl Pts',(15.3208543776412,6.87857591366295,13.364240995629));
#15564=CARTESIAN_POINT('Ctrl Pts',(15.5946518761319,6.9297016229862,13.648017855189));
#15565=CARTESIAN_POINT('Ctrl Pts',(15.7315506253773,6.95526524865973,13.7899072524002));
#15566=CARTESIAN_POINT('Ctrl Pts',(15.8,6.9680463746276,13.8608510891535));
#15567=CARTESIAN_POINT('Ctrl Pts',(10.0502525316942,5.80163007173556,7.66237562613099));
#15568=CARTESIAN_POINT('Ctrl Pts',(11.1454425256572,6.00977287125003,8.76621669669801));
#15569=CARTESIAN_POINT('Ctrl Pts',(12.3775312688656,6.24400287259233,10.008064757174));
#15570=CARTESIAN_POINT('Ctrl Pts',(13.7465187613193,6.50418764618808,11.3878685250288));
#15571=CARTESIAN_POINT('Ctrl Pts',(14.2941137583008,6.60826243593383,11.9397903730643));
#15572=CARTESIAN_POINT('Ctrl Pts',(14.8417087552823,6.71234494803682,12.4917152115347));
#15573=CARTESIAN_POINT('Ctrl Pts',(15.3208543776411,6.80341474110255,12.9746485138656));
#15574=CARTESIAN_POINT('Ctrl Pts',(15.5946518761319,6.8554516400659,13.2506092458454));
#15575=CARTESIAN_POINT('Ctrl Pts',(15.7315506253773,6.8814708564871,13.3885899088279));
#15576=CARTESIAN_POINT('Ctrl Pts',(15.8,6.89447978145675,13.4575799757384));
#15577=CARTESIAN_POINT('Ctrl Pts',(10.0502525316942,5.68351040711506,7.44593237535689));
#15578=CARTESIAN_POINT('Ctrl Pts',(11.1454425256572,5.89012315163306,8.51992624992032));
#15579=CARTESIAN_POINT('Ctrl Pts',(12.3775312688656,6.12263633930511,9.72815762348206));
#15580=CARTESIAN_POINT('Ctrl Pts',(13.7465187613194,6.38090895110343,11.0706489050024));
#15581=CARTESIAN_POINT('Ctrl Pts',(14.2941137583009,6.48421893322742,11.60764526865));
#15582=CARTESIAN_POINT('Ctrl Pts',(14.8417087552824,6.5875371385849,12.1446403255654));
#15583=CARTESIAN_POINT('Ctrl Pts',(15.3208543776412,6.67793800725713,12.6145114073305));
#15584=CARTESIAN_POINT('Ctrl Pts',(15.594651876132,6.72959247024464,12.8830096730692));
#15585=CARTESIAN_POINT('Ctrl Pts',(15.7315506253773,6.75542051842203,13.0172586761616));
#15586=CARTESIAN_POINT('Ctrl Pts',(15.8,6.7683338149544,13.0843832933218));
#15587=CARTESIAN_POINT('Ctrl Pts',(10.0502525316942,5.60747221894231,7.3491344951621));
#15588=CARTESIAN_POINT('Ctrl Pts',(11.1454425256572,5.81105284226644,8.40845336995524));
#15589=CARTESIAN_POINT('Ctrl Pts',(12.3775312688656,6.04008639989118,9.60029668798143));
#15590=CARTESIAN_POINT('Ctrl Pts',(13.7465187613193,6.29456266363366,10.9244551954278));
#15591=CARTESIAN_POINT('Ctrl Pts',(14.2941137583009,6.3963532371211,11.4541199893924));
#15592=CARTESIAN_POINT('Ctrl Pts',(14.8417087552824,6.49814440704391,11.9837969855611));
#15593=CARTESIAN_POINT('Ctrl Pts',(15.3208543776412,6.58721149497458,12.4472605569962));
#15594=CARTESIAN_POINT('Ctrl Pts',(15.5946518761319,6.63810674341679,12.7120921703849));
#15595=CARTESIAN_POINT('Ctrl Pts',(15.7315506253773,6.66355442687238,12.8445091889311));
#15596=CARTESIAN_POINT('Ctrl Pts',(15.8,6.67627821583013,12.9107166186057));
#15597=CARTESIAN_POINT('Ctrl Pts',(10.0502525316942,5.55043285230422,7.28928030147641));
#15598=CARTESIAN_POINT('Ctrl Pts',(11.1454425256572,5.75098891959401,8.33905665452735));
#15599=CARTESIAN_POINT('Ctrl Pts',(12.3775312688656,5.97661449529503,9.52005505170966));
#15600=CARTESIAN_POINT('Ctrl Pts',(13.7465187613193,6.22730957940727,10.8322754930233));
#15601=CARTESIAN_POINT('Ctrl Pts',(14.2941137583009,6.32758761305217,11.3571636695488));
#15602=CARTESIAN_POINT('Ctrl Pts',(14.8417087552824,6.42786564669707,11.8820518460743));
#15603=CARTESIAN_POINT('Ctrl Pts',(15.3208543776412,6.51560892613635,12.3413290005341));
#15604=CARTESIAN_POINT('Ctrl Pts',(15.5946518761319,6.5657479429588,12.6037730887968));
#15605=CARTESIAN_POINT('Ctrl Pts',(15.7315506253773,6.59081745137003,12.7349951329282));
#15606=CARTESIAN_POINT('Ctrl Pts',(15.8,6.60335220557564,12.8006061549939));
#15607=CARTESIAN_POINT('Ctrl Pts',(15.8,6.62691983743441,12.8370600702028));
#15608=CARTESIAN_POINT('Ctrl Pts',(15.8,6.62229417791417,12.8297280642598));
#15609=CARTESIAN_POINT('Ctrl Pts',(15.8,6.61762457479065,12.8224166748639));
#15610=CARTESIAN_POINT('Ctrl Pts',(15.8,6.61291104065239,12.8151258955788));
#15611=CARTESIAN_POINT('Ctrl Pts',(15.8,6.60815358414732,12.8078557223109));
#15612=CARTESIAN_POINT('Ctrl Pts',(15.8,6.60335220557564,12.8006061549939));
#15613=CARTESIAN_POINT('Origin',(15.8,5.67212567669951,13.950492764499));
#15614=CARTESIAN_POINT('Ctrl Pts',(10.0502525316942,8.05467776187827,7.13578365451838));
#15615=CARTESIAN_POINT('Ctrl Pts',(11.1454425256572,8.52471396348012,8.29974860990865));
#15616=CARTESIAN_POINT('Ctrl Pts',(12.3775312688656,9.05350469028219,9.6092091847227));
#15617=CARTESIAN_POINT('Ctrl Pts',(13.7465187613193,9.6410499422845,11.0641653789605));
#15618=CARTESIAN_POINT('Ctrl Pts',(14.2941137583009,9.87606804308543,11.6461478566557));
#15619=CARTESIAN_POINT('Ctrl Pts',(14.8417087552824,10.1110861438864,12.2281303343508));
#15620=CARTESIAN_POINT('Ctrl Pts',(15.3208543776412,10.3167269820872,12.737365002334));
#15621=CARTESIAN_POINT('Ctrl Pts',(15.5946518761319,10.4342360324876,13.0283562411816));
#15622=CARTESIAN_POINT('Ctrl Pts',(15.7315506253773,10.4929905576879,13.1738518606054));
#15623=CARTESIAN_POINT('Ctrl Pts',(15.8,10.522367820288,13.2465996703173));
#15624=CARTESIAN_POINT('Ctrl Pts',(10.0502525316942,8.19339868393687,6.89902655578542));
#15625=CARTESIAN_POINT('Ctrl Pts',(11.1454425256572,8.68853919251131,8.04889405860839));
#15626=CARTESIAN_POINT('Ctrl Pts',(12.3775312688656,9.24602752966092,9.34238794408147));
#15627=CARTESIAN_POINT('Ctrl Pts',(13.7465187613193,9.86499535005157,10.779712402918));
#15628=CARTESIAN_POINT('Ctrl Pts',(14.2941137583009,10.1125880646808,11.354640872798));
#15629=CARTESIAN_POINT('Ctrl Pts',(14.8417087552824,10.3602324253388,11.9295571981554));
#15630=CARTESIAN_POINT('Ctrl Pts',(15.3208543776412,10.5769051976768,12.4326127553978));
#15631=CARTESIAN_POINT('Ctrl Pts',(15.5946518761319,10.7006983402633,12.7200777462785));
#15632=CARTESIAN_POINT('Ctrl Pts',(15.7315506253773,10.7626000339661,12.8638090371883));
#15633=CARTESIAN_POINT('Ctrl Pts',(15.8,10.793546315752,12.9356757561148));
#15634=CARTESIAN_POINT('Ctrl Pts',(10.0502525316942,8.36661813687799,6.51604789180993));
#15635=CARTESIAN_POINT('Ctrl Pts',(11.1454425256572,8.89900085425541,7.63881390938367));
#15636=CARTESIAN_POINT('Ctrl Pts',(12.3775312688656,9.49738068383038,8.90205445633838));
#15637=CARTESIAN_POINT('Ctrl Pts',(13.7465187613194,10.1628080503653,10.3055239107478));
#15638=CARTESIAN_POINT('Ctrl Pts',(14.2941137583009,10.4289722391039,10.8669132727127));
#15639=CARTESIAN_POINT('Ctrl Pts',(14.8417087552824,10.6950739523901,11.4283172433782));
#15640=CARTESIAN_POINT('Ctrl Pts',(15.3208543776412,10.9279323587878,11.9195411796877));
#15641=CARTESIAN_POINT('Ctrl Pts',(15.594651876132,11.0610183419671,12.2002349513456));
#15642=CARTESIAN_POINT('Ctrl Pts',(15.7315506253773,11.1275551370522,12.3405832861097));
#15643=CARTESIAN_POINT('Ctrl Pts',(15.8,11.1608290568882,12.4107561622081));
#15644=CARTESIAN_POINT('Ctrl Pts',(10.0502525316942,8.32768215464935,6.25935291859365));
#15645=CARTESIAN_POINT('Ctrl Pts',(11.1454425256572,8.87221159590509,7.35179456409855));
#15646=CARTESIAN_POINT('Ctrl Pts',(12.3775312688656,9.48507728715608,8.58070593097969));
#15647=CARTESIAN_POINT('Ctrl Pts',(13.7465187613193,10.1657641132886,9.94625006691877));
#15648=CARTESIAN_POINT('Ctrl Pts',(14.2941137583008,10.4380421577189,10.4924666723322));
#15649=CARTESIAN_POINT('Ctrl Pts',(14.8417087552823,10.7103508393265,11.0386735802612));
#15650=CARTESIAN_POINT('Ctrl Pts',(15.3208543776411,10.9486114186505,11.5166076371098));
#15651=CARTESIAN_POINT('Ctrl Pts',(15.5946518761319,11.0847485338421,11.7897165434404));
#15652=CARTESIAN_POINT('Ctrl Pts',(15.7315506253773,11.1528201301259,11.9262700347798));
#15653=CARTESIAN_POINT('Ctrl Pts',(15.8,11.1868532202043,11.9945476376238));
#15654=CARTESIAN_POINT('Ctrl Pts',(10.0502525316942,8.2376185172569,6.10559301495173));
#15655=CARTESIAN_POINT('Ctrl Pts',(11.1454425256572,8.78181727442992,7.17588579216884));
#15656=CARTESIAN_POINT('Ctrl Pts',(12.3775312688656,9.39427431712613,8.37997276877534));
#15657=CARTESIAN_POINT('Ctrl Pts',(13.7465187613193,10.0745443941304,9.71783944471699));
#15658=CARTESIAN_POINT('Ctrl Pts',(14.2941137583008,10.3466552894421,10.2529862083793));
#15659=CARTESIAN_POINT('Ctrl Pts',(14.8417087552824,10.61879266668,10.7881338344522));
#15660=CARTESIAN_POINT('Ctrl Pts',(15.3208543776412,10.856904645461,11.2563877393682));
#15661=CARTESIAN_POINT('Ctrl Pts',(15.5946518761319,10.9929584447385,11.5239610675182));
#15662=CARTESIAN_POINT('Ctrl Pts',(15.7315506253773,11.0609879709349,11.6577478171298));
#15663=CARTESIAN_POINT('Ctrl Pts',(15.8,11.0950003932583,11.7246411157058));
#15664=CARTESIAN_POINT('Ctrl Pts',(10.0502525316941,8.15474945546093,5.94621492062452));
#15665=CARTESIAN_POINT('Ctrl Pts',(11.1454425256572,8.6982675895859,6.99511596848632));
#15666=CARTESIAN_POINT('Ctrl Pts',(12.3775312688656,9.30992859260386,8.17501015002258));
#15667=CARTESIAN_POINT('Ctrl Pts',(13.7465187613193,9.98934507962172,9.48612538727718));
#15668=CARTESIAN_POINT('Ctrl Pts',(14.2941137583008,10.2611141666576,10.0105700158496));
#15669=CARTESIAN_POINT('Ctrl Pts',(14.8417087552823,10.532906293941,10.535001088446));
#15670=CARTESIAN_POINT('Ctrl Pts',(15.3208543776412,10.7707172481292,10.9938824879741));
#15671=CARTESIAN_POINT('Ctrl Pts',(15.5946518761319,10.9066003574976,11.2561056460575));
#15672=CARTESIAN_POINT('Ctrl Pts',(15.7315506253773,10.9745441973833,11.3872158805765));
#15673=CARTESIAN_POINT('Ctrl Pts',(15.8,11.0085140807661,11.4527721960679));
#15674=CARTESIAN_POINT('Ctrl Pts',(10.0502525316942,8.04752551167497,5.69326714724858));
#15675=CARTESIAN_POINT('Ctrl Pts',(11.1454425256572,8.59278030111936,6.70961935691121));
#15676=CARTESIAN_POINT('Ctrl Pts',(12.3775312688656,9.20628631668581,7.85307681747465));
#15677=CARTESIAN_POINT('Ctrl Pts',(13.7465187613193,9.88786354846716,9.12352275260843));
#15678=CARTESIAN_POINT('Ctrl Pts',(14.2941137583008,10.1604955992679,9.63170187793887));
#15679=CARTESIAN_POINT('Ctrl Pts',(14.8417087552823,10.4331383564046,10.1398879487016));
#15680=CARTESIAN_POINT('Ctrl Pts',(15.3208543776412,10.6716974431005,10.5845486031013));
#15681=CARTESIAN_POINT('Ctrl Pts',(15.5946518761319,10.8080128020806,10.8386377334452));
#15682=CARTESIAN_POINT('Ctrl Pts',(15.7315506253773,10.8761715434575,10.9656829874862));
#15683=CARTESIAN_POINT('Ctrl Pts',(15.8,10.9102499677978,11.0292050005901));
#15684=CARTESIAN_POINT('Ctrl Pts',(10.0502525316942,7.88548479029559,5.49454791241253));
#15685=CARTESIAN_POINT('Ctrl Pts',(11.1454425256572,8.42454600598798,6.48004349322277));
#15686=CARTESIAN_POINT('Ctrl Pts',(12.3775312688655,9.03106484753222,7.58873003819359));
#15687=CARTESIAN_POINT('Ctrl Pts',(13.7465187613193,9.70489831419831,8.82059988637915));
#15688=CARTESIAN_POINT('Ctrl Pts',(14.2941137583008,9.97443262085554,9.31334787493984));
#15689=CARTESIAN_POINT('Ctrl Pts',(14.8417087552823,10.2439754326772,9.80609631914578));
#15690=CARTESIAN_POINT('Ctrl Pts',(15.3208543776411,10.4798227509907,10.2372510662851));
#15691=CARTESIAN_POINT('Ctrl Pts',(15.5946518761319,10.614589374912,10.4836250322036));
#15692=CARTESIAN_POINT('Ctrl Pts',(15.7315506253773,10.6819735304405,10.6068120603551));
#15693=CARTESIAN_POINT('Ctrl Pts',(15.8,10.7156648564213,10.6684055341558));
#15694=CARTESIAN_POINT('Ctrl Pts',(10.0502525316942,7.70626127860213,5.3251994701061));
#15695=CARTESIAN_POINT('Ctrl Pts',(11.1454425256572,8.23464403472029,6.28278149366022));
#15696=CARTESIAN_POINT('Ctrl Pts',(12.3775312688656,8.82914182271548,7.36002740501519));
#15697=CARTESIAN_POINT('Ctrl Pts',(13.7465187613194,9.48962649341722,8.55700179652723));
#15698=CARTESIAN_POINT('Ctrl Pts',(14.2941137583009,9.75382118614165,9.03579113757912));
#15699=CARTESIAN_POINT('Ctrl Pts',(14.8417087552824,10.0180235007136,9.51457663691209));
#15700=CARTESIAN_POINT('Ctrl Pts',(15.3208543776412,10.2491981583259,9.93351514221371));
#15701=CARTESIAN_POINT('Ctrl Pts',(15.594651876132,10.3812950302631,10.172910051869));
#15702=CARTESIAN_POINT('Ctrl Pts',(15.7315506253773,10.4473442221896,10.2926071256633));
#15703=CARTESIAN_POINT('Ctrl Pts',(15.8,10.480368144447,10.3524560021355));
#15704=CARTESIAN_POINT('Ctrl Pts',(10.0502525316942,7.60403044672136,5.25663803961482));
#15705=CARTESIAN_POINT('Ctrl Pts',(11.1454425256572,8.12499465989844,6.2012002859887));
#15706=CARTESIAN_POINT('Ctrl Pts',(12.3775312688656,8.71111815506916,7.26393484617381));
#15707=CARTESIAN_POINT('Ctrl Pts',(13.7465187613193,9.36232701259537,8.44464710847935));
#15708=CARTESIAN_POINT('Ctrl Pts',(14.2941137583009,9.62281103116557,8.91693326542987));
#15709=CARTESIAN_POINT('Ctrl Pts',(14.8417087552824,9.88329944620756,9.38923099717744));
#15710=CARTESIAN_POINT('Ctrl Pts',(15.3208543776412,10.1112254436565,9.80248791688055));
#15711=CARTESIAN_POINT('Ctrl Pts',(15.5946518761319,10.2414671792814,10.0386302748779));
#15712=CARTESIAN_POINT('Ctrl Pts',(15.7315506253773,10.3065884831493,10.1567026019));
#15713=CARTESIAN_POINT('Ctrl Pts',(15.8,10.3391487464728,10.2157377422983));
#15714=CARTESIAN_POINT('Ctrl Pts',(10.0502525316942,7.53128682236137,5.21733945232202));
#15715=CARTESIAN_POINT('Ctrl Pts',(11.1454425256572,8.04642571042556,6.15376086042613));
#15716=CARTESIAN_POINT('Ctrl Pts',(12.3775312688656,8.62595695949776,7.20723494454326));
#15717=CARTESIAN_POINT('Ctrl Pts',(13.7465187613193,9.269880569578,8.3777617046734));
#15718=CARTESIAN_POINT('Ctrl Pts',(14.2941137583009,9.52745001361009,8.84597240872545));
#15719=CARTESIAN_POINT('Ctrl Pts',(14.8417087552824,9.78501945764218,9.31418311277751));
#15720=CARTESIAN_POINT('Ctrl Pts',(15.3208543776412,10.0103927211703,9.72386747882306));
#15721=CARTESIAN_POINT('Ctrl Pts',(15.5946518761319,10.1391774431863,9.95797283084909));
#15722=CARTESIAN_POINT('Ctrl Pts',(15.7315506253773,10.2035698041943,10.0750255068621));
#15723=CARTESIAN_POINT('Ctrl Pts',(15.8,10.2357659846983,10.1335518448686));
#15724=CARTESIAN_POINT('Ctrl Pts',(15.8,10.2694450138623,10.160938779711));
#15725=CARTESIAN_POINT('Ctrl Pts',(15.8,10.2627800357942,10.1553950350833));
#15726=CARTESIAN_POINT('Ctrl Pts',(15.8,10.2560796357392,10.1498844772774));
#15727=CARTESIAN_POINT('Ctrl Pts',(15.8,10.2493438236809,10.1444070962816));
#15728=CARTESIAN_POINT('Ctrl Pts',(15.8,10.242572606579,10.1389628855307));
#15729=CARTESIAN_POINT('Ctrl Pts',(15.8,10.2357659846983,10.1335518448686));
#15730=CARTESIAN_POINT('Origin',(15.8,9.70545143020505,11.5149238208745));
#15731=CARTESIAN_POINT('Ctrl Pts',(10.0502525316942,9.86553218952113,4.2975012308678));
#15732=CARTESIAN_POINT('Ctrl Pts',(11.9668350211294,11.2772850923971,5.98055897313701));
#15733=CARTESIAN_POINT('Ctrl Pts',(13.8834175105647,12.689037995273,7.66361671540623));
#15734=CARTESIAN_POINT('Ctrl Pts',(15.8,14.1007908981489,9.34667445767544));
#15735=CARTESIAN_POINT('Ctrl Pts',(10.0502525316942,9.92430165934404,4.02946472694721));
#15736=CARTESIAN_POINT('Ctrl Pts',(11.9668350211294,11.3702854403574,5.67542688932036));
#15737=CARTESIAN_POINT('Ctrl Pts',(13.8834175105647,12.8166324188796,7.32120731702057));
#15738=CARTESIAN_POINT('Ctrl Pts',(15.8,14.262616199893,8.96716947939373));
#15739=CARTESIAN_POINT('Ctrl Pts',(10.0502525316942,9.97045860619055,3.61211062987325));
#15740=CARTESIAN_POINT('Ctrl Pts',(11.9668350211294,11.4635526451079,5.19299729643612));
#15741=CARTESIAN_POINT('Ctrl Pts',(13.8834175105647,12.956112555571,6.77411605990067));
#15742=CARTESIAN_POINT('Ctrl Pts',(15.8,14.4492065944883,8.35500272646354));
#15743=CARTESIAN_POINT('Ctrl Pts',(10.0502525316942,9.86609404202409,3.40259706500424));
#15744=CARTESIAN_POINT('Ctrl Pts',(11.9668350211294,11.3629139742223,4.93192196434908));
#15745=CARTESIAN_POINT('Ctrl Pts',(13.8834175105647,12.8596985741914,6.4612970474202));
#15746=CARTESIAN_POINT('Ctrl Pts',(15.8,14.3565185063896,7.99062194676504));
#15747=CARTESIAN_POINT('Ctrl Pts',(10.0502525316942,9.77087387154055,3.30601090928165));
#15748=CARTESIAN_POINT('Ctrl Pts',(11.9668350211295,11.2600017151873,4.80688444200922));
#15749=CARTESIAN_POINT('Ctrl Pts',(13.8834175105647,12.7494883087274,6.30755492143114));
#15750=CARTESIAN_POINT('Ctrl Pts',(15.8,14.2386161523742,7.8084284541587));
#15751=CARTESIAN_POINT('Ctrl Pts',(10.0502525316942,9.7053049496755,3.24522078037662));
#15752=CARTESIAN_POINT('Ctrl Pts',(11.9668350211294,11.1883166806211,4.72781700580775));
#15753=CARTESIAN_POINT('Ctrl Pts',(13.8834175105647,12.6715703878316,6.21037804061048));
#15754=CARTESIAN_POINT('Ctrl Pts',(15.8,14.1545821187772,7.69297426604161));
#15755=CARTESIAN_POINT('Ctrl Pts',(10.0502525316942,9.59290229251195,3.13558852137588));
#15756=CARTESIAN_POINT('Ctrl Pts',(11.9668350211294,11.0646742694966,4.58744122478927));
#15757=CARTESIAN_POINT('Ctrl Pts',(13.8834175105647,12.5366026187688,6.03905717649215));
#15758=CARTESIAN_POINT('Ctrl Pts',(15.8,14.0083745957535,7.49090987990554));
#15759=CARTESIAN_POINT('Ctrl Pts',(10.0502525316942,9.41310152025599,2.92757116168119));
#15760=CARTESIAN_POINT('Ctrl Pts',(11.9668350211294,10.8702564567215,4.32424671627921));
#15761=CARTESIAN_POINT('Ctrl Pts',(13.8834175105647,12.3275956094625,5.72097159497831));
#15762=CARTESIAN_POINT('Ctrl Pts',(15.8,13.784750545928,7.11764714957634));
#15763=CARTESIAN_POINT('Ctrl Pts',(10.0502525316942,9.19740926566326,2.78894862571459));
#15764=CARTESIAN_POINT('Ctrl Pts',(11.9668350211294,10.6275127538178,4.13765656795514));
#15765=CARTESIAN_POINT('Ctrl Pts',(13.8834175105647,12.0577280234799,5.48632659127462));
#15766=CARTESIAN_POINT('Ctrl Pts',(15.8,13.4878315116344,6.83503453351516));
#15767=CARTESIAN_POINT('Ctrl Pts',(10.0502525316942,8.97469639188219,2.6831512960299));
#15768=CARTESIAN_POINT('Ctrl Pts',(11.9668350211294,10.3719655284903,3.99115284441714));
#15769=CARTESIAN_POINT('Ctrl Pts',(13.8834175105647,11.7692966119437,5.29909475352163));
#15770=CARTESIAN_POINT('Ctrl Pts',(15.8,13.1665657485518,6.60709630190886));
#15771=CARTESIAN_POINT('Ctrl Pts',(10.0502525316942,8.85625319397989,2.64958522759924));
#15772=CARTESIAN_POINT('Ctrl Pts',(11.9668350211294,10.2341088589535,3.9399468856208));
#15773=CARTESIAN_POINT('Ctrl Pts',(13.8834175105647,11.612095695752,5.23040962052305));
#15774=CARTESIAN_POINT('Ctrl Pts',(15.8,12.9899513607256,6.52077127854461));
#15775=CARTESIAN_POINT('Ctrl Pts',(10.0502525316942,8.77492596468499,2.63468906623289));
#15776=CARTESIAN_POINT('Ctrl Pts',(11.9668350211294,10.1386945339445,3.91464433600868));
#15777=CARTESIAN_POINT('Ctrl Pts',(13.8834175105647,11.5024631032041,5.19459960578447));
#15778=CARTESIAN_POINT('Ctrl Pts',(15.8,12.8662316724636,6.47455487556026));
#15779=CARTESIAN_POINT('Ctrl Pts',(15.8,12.9067253609027,6.49019400603778));
#15780=CARTESIAN_POINT('Ctrl Pts',(15.8,12.8986734787776,6.48698118307512));
#15781=CARTESIAN_POINT('Ctrl Pts',(15.8,12.890598163633,6.48381086865141));
#15782=CARTESIAN_POINT('Ctrl Pts',(15.8,12.8824994218701,6.48068305016015));
#15783=CARTESIAN_POINT('Ctrl Pts',(15.8,12.874377258079,6.47759771920651));
#15784=CARTESIAN_POINT('Ctrl Pts',(15.8,12.8662316724636,6.47455487556026));
#15785=CARTESIAN_POINT('Origin',(15.8,12.7887399758658,7.95219390447097));
#15786=CARTESIAN_POINT('Ctrl Pts',(10.0502525316942,10.7106795892491,1.03854944428815));
#15787=CARTESIAN_POINT('Ctrl Pts',(11.9668350211294,12.5734298318033,2.20297683852746));
#15788=CARTESIAN_POINT('Ctrl Pts',(13.8834175105647,14.4361800743576,3.36740423276678));
#15789=CARTESIAN_POINT('Ctrl Pts',(15.8,16.2989303169119,4.5318316270061));
#15790=CARTESIAN_POINT('Ctrl Pts',(10.0502525316942,10.6837448416591,0.765470815703815));
#15791=CARTESIAN_POINT('Ctrl Pts',(11.9668350211294,12.5675874193204,1.88404029388038));
#15792=CARTESIAN_POINT('Ctrl Pts',(13.8834175105647,14.4517192592367,3.00232469790949));
#15793=CARTESIAN_POINT('Ctrl Pts',(15.8,16.335561836898,4.12089417608606));
#15794=CARTESIAN_POINT('Ctrl Pts',(10.0502525316942,10.5986742216641,0.354275884655605));
#15795=CARTESIAN_POINT('Ctrl Pts',(11.9668350211295,12.5072118829665,1.39639701818897));
#15796=CARTESIAN_POINT('Ctrl Pts',(13.8834175105647,14.4153151096237,2.43890221878173));
#15797=CARTESIAN_POINT('Ctrl Pts',(15.8,16.3238527709261,3.48102335231509));
#15798=CARTESIAN_POINT('Ctrl Pts',(10.0502525316942,10.4346757823309,0.187261072828499));
#15799=CARTESIAN_POINT('Ctrl Pts',(11.9668350211295,12.3308235163868,1.17919268731443));
#15800=CARTESIAN_POINT('Ctrl Pts',(13.8834175105647,14.2269575174279,2.17117887432507));
#15801=CARTESIAN_POINT('Ctrl Pts',(15.8,16.1231052514838,3.16311048881099));
#15802=CARTESIAN_POINT('Ctrl Pts',(10.0502525316942,10.3142698682631,0.124824203483034));
#15803=CARTESIAN_POINT('Ctrl Pts',(11.9668350211295,12.1943100355803,1.09207394643473));
#15804=CARTESIAN_POINT('Ctrl Pts',(13.8834175105647,14.0746341437949,2.05901454824882));
#15805=CARTESIAN_POINT('Ctrl Pts',(15.8,15.9546743111122,3.02626429120052));
#15806=CARTESIAN_POINT('Ctrl Pts',(10.0502525316942,10.2331249635989,0.0872711810328567));
#15807=CARTESIAN_POINT('Ctrl Pts',(11.9668350211295,12.1017003635113,1.03902815454411));
#15808=CARTESIAN_POINT('Ctrl Pts',(13.8834175105647,13.9705005205662,1.99067177195528));
#15809=CARTESIAN_POINT('Ctrl Pts',(15.8,15.8390759204785,2.94242874546654));
#15810=CARTESIAN_POINT('Ctrl Pts',(10.0502525316942,10.09234540735,0.0177390798696556));
#15811=CARTESIAN_POINT('Ctrl Pts',(11.9668350211294,11.9407308952458,0.943730501418608));
#15812=CARTESIAN_POINT('Ctrl Pts',(13.8834175105647,13.789197555515,1.86944300220409));
#15813=CARTESIAN_POINT('Ctrl Pts',(15.8,15.6375830434108,2.79543442375304));
#15814=CARTESIAN_POINT('Ctrl Pts',(10.0502525316942,9.85706386916291,-0.124535428292432));
#15815=CARTESIAN_POINT('Ctrl Pts',(11.9668350211295,11.6744970487389,0.753496320252986));
#15816=CARTESIAN_POINT('Ctrl Pts',(13.8834175105647,13.4921256030567,1.6315141640905));
#15817=CARTESIAN_POINT('Ctrl Pts',(15.8,15.3095587826327,2.50954591263591));
#15818=CARTESIAN_POINT('Ctrl Pts',(10.0502525316942,9.60909091476054,-0.189717758784554));
#15819=CARTESIAN_POINT('Ctrl Pts',(11.9668350211294,11.3859738307471,0.651053436707716));
#15820=CARTESIAN_POINT('Ctrl Pts',(13.8834175105647,13.1629551482145,1.49175101418763));
#15821=CARTESIAN_POINT('Ctrl Pts',(15.8,14.9398380642011,2.3325222096799));
#15822=CARTESIAN_POINT('Ctrl Pts',(10.0502525316942,9.36458479377687,-0.221513186022212));
#15823=CARTESIAN_POINT('Ctrl Pts',(11.9668350211294,11.0976614182865,0.59069030096811));
#15824=CARTESIAN_POINT('Ctrl Pts',(13.8834175105648,12.8307816497324,1.40281548080796));
#15825=CARTESIAN_POINT('Ctrl Pts',(15.8,14.563858274242,2.21501896779828));
#15826=CARTESIAN_POINT('Ctrl Pts',(10.0502525316942,9.24156417346731,-0.216827447239559));
#15827=CARTESIAN_POINT('Ctrl Pts',(11.9668350211294,10.9507264633732,0.584598599726621));
#15828=CARTESIAN_POINT('Ctrl Pts',(13.8834175105647,12.6600447395717,1.38608024219576));
#15829=CARTESIAN_POINT('Ctrl Pts',(15.8,14.3692070294775,2.18750628916194));
#15830=CARTESIAN_POINT('Ctrl Pts',(10.0502525316942,9.15961421508102,-0.20586304261726));
#15831=CARTESIAN_POINT('Ctrl Pts',(11.9668350211294,10.8521631299943,0.590019092973717));
#15832=CARTESIAN_POINT('Ctrl Pts',(13.8834175105647,12.5447120449076,1.38590122856469));
#15833=CARTESIAN_POINT('Ctrl Pts',(15.8,14.2372609598209,2.18178336415567));
#15834=CARTESIAN_POINT('Ctrl Pts',(15.8,14.2806055031745,2.18414382321291));
#15835=CARTESIAN_POINT('Ctrl Pts',(15.8,14.2719548913156,2.18357641541193));
#15836=CARTESIAN_POINT('Ctrl Pts',(15.8,14.2632951291918,2.18305667683518));
#15837=CARTESIAN_POINT('Ctrl Pts',(15.8,14.2546262189952,2.18258459351507));
#15838=CARTESIAN_POINT('Ctrl Pts',(15.8,14.2459481624974,2.18216015604922));
#15839=CARTESIAN_POINT('Ctrl Pts',(15.8,14.2372609598209,2.18178336415567));
#15840=CARTESIAN_POINT('Origin',(15.8,14.6201775482978,3.61104784250494));
#15841=CARTESIAN_POINT('Origin',(21.,10.,0.));
#23233=UNCERTAINTY_MEASURE_WITH_UNIT(LENGTH_MEASURE(0.01),#23255,
'DISTANCE_ACCURACY_VALUE',
'Maximum model space distance between geometric entities at asserted c
onnectivities');
#23242=UNCERTAINTY_MEASURE_WITH_UNIT(LENGTH_MEASURE(0.01),#23255,
'DISTANCE_ACCURACY_VALUE',
'Maximum model space distance between geometric entities at asserted c
onnectivities');
#23245=(
GEOMETRIC_REPRESENTATION_CONTEXT(3)
GLOBAL_UNCERTAINTY_ASSIGNED_CONTEXT((#23233))
GLOBAL_UNIT_ASSIGNED_CONTEXT((#23255,#23257,#23258))
REPRESENTATION_CONTEXT('','3D')
);
#23254=(
GEOMETRIC_REPRESENTATION_CONTEXT(3)
GLOBAL_UNCERTAINTY_ASSIGNED_CONTEXT((#23242))
GLOBAL_UNIT_ASSIGNED_CONTEXT((#23255,#23257,#23258))
REPRESENTATION_CONTEXT('','3D')
);
#23255=(
LENGTH_UNIT()
NAMED_UNIT(*)
SI_UNIT(.MILLI.,.METRE.)
);
#23257=(
NAMED_UNIT(*)
PLANE_ANGLE_UNIT()
SI_UNIT($,.RADIAN.)
);
#23258=(
NAMED_UNIT(*)
SI_UNIT($,.STERADIAN.)
SOLID_ANGLE_UNIT()
);
#23261=SHAPE_DEFINITION_REPRESENTATION(#23272,#23301);
#23272=PRODUCT_DEFINITION_SHAPE('',$,#23313);
#23301=SHAPE_REPRESENTATION('',(#7279),#23245);
#23310=PRODUCT_DEFINITION_CONTEXT('part definition',#23345,'design');
#23313=PRODUCT_DEFINITION('2026-10-11-09-11-48-335',
'02_Spiral_Bevel_Input_Pinion_M1.5_Z20_LH',#23324,#23310);
#23324=PRODUCT_DEFINITION_FORMATION('',$,#23349);
#23345=APPLICATION_CONTEXT(
'Core Data for Automotive Mechanical Design Process');
#23346=PRODUCT_CONTEXT('part definition',#23345,'mechanical');
#23349=PRODUCT('2026-10-11-09-11-48-335',
'02_Spiral_Bevel_Input_Pinion_M1.5_Z20_LH',$,(#23346));
#23442=COLOUR_RGB('Light Blue',0.38,0.62,0.78);
#23443=FILL_AREA_STYLE_COLOUR('',#23442);
#23444=FILL_AREA_STYLE('',(#23443));
#23445=SURFACE_STYLE_FILL_AREA(#23444);
#23446=SURFACE_SIDE_STYLE('',(#23445));
#23447=SURFACE_STYLE_USAGE(.BOTH.,#23446);
#23448=PRESENTATION_STYLE_ASSIGNMENT((#23447));
ENDSEC;
END-ISO-10303-21;
